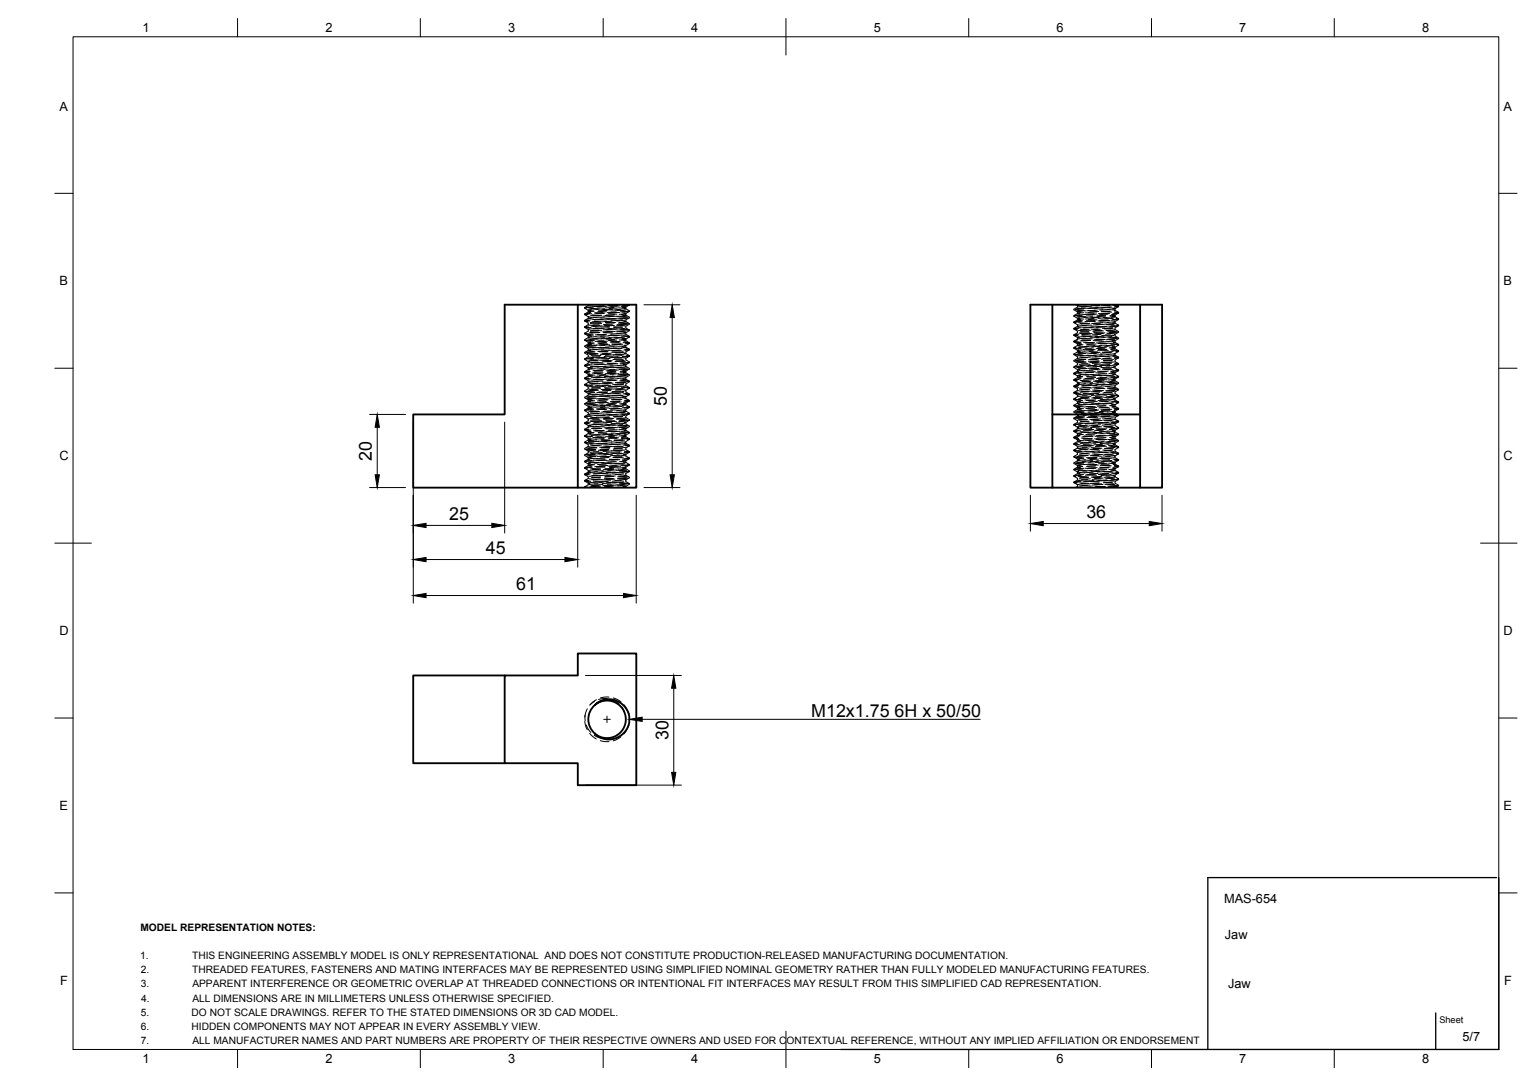
ISO-10303-21;
HEADER;
/* Generated by software containing ST-Developer
 * from STEP Tools, Inc. (www.steptools.com) 
 */

FILE_DESCRIPTION(
/* description */ ('Independent four-jaw lathe chuck,200mm body,40mm bore,36\X2\2013\X0\7
6mm nominal opposed jaw opening. Four shared machined T-jaws and model
ed partial M12x1.75 feed screws, native independent screw/slider links
, removable bolted bronze-bearing cartridges, fully captured ring/wash
er/head thrust stacks and registered bolted backplate. Custom spindle 
interface; no compatibility, speed, grip force or safety rating assign
ed.'),
/* implementation_level */ '2;1');

FILE_NAME(
/* name */ 'Jaw.step',
/* time_stamp */ '2026-11-09T20:24:54-08:00',
/* author */ (''),
/* organization */ (''),
/* preprocessor_version */ 'ST-DEVELOPER v20.2',
/* originating_system */ 'Autodesk Translation Framework v15.17.0.0',
/* authorisation */ '');

FILE_SCHEMA (('AUTOMOTIVE_DESIGN { 1 0 10303 214 3 1 1 }'));
ENDSEC;

DATA;
#10=MECHANICAL_DESIGN_GEOMETRIC_PRESENTATION_REPRESENTATION('',(#238),#69491);
#216=SHAPE_REPRESENTATION_RELATIONSHIP('SRR','None',#69573,#227);
#227=ADVANCED_BREP_SHAPE_REPRESENTATION('',(#249),#69482);
#238=STYLED_ITEM('',(#69637),#249);
#249=MANIFOLD_SOLID_BREP('Body1',#14733);
#290=B_SPLINE_SURFACE_WITH_KNOTS('',3,3,((#46765,#46766,#46767,#46768,#46769,
#46770,#46771,#46772,#46773,#46774,#46775,#46776,#46777,#46778,#46779,#46780,
#46781,#46782,#46783,#46784,#46785,#46786,#46787,#46788,#46789,#46790,#46791,
#46792,#46793,#46794,#46795,#46796,#46797,#46798,#46799,#46800,#46801,#46802,
#46803,#46804,#46805,#46806,#46807,#46808,#46809,#46810,#46811,#46812,#46813,
#46814,#46815,#46816,#46817,#46818,#46819,#46820,#46821,#46822,#46823,#46824,
#46825,#46826,#46827,#46828,#46829,#46830,#46831,#46832,#46833,#46834,#46835,
#46836,#46837,#46838,#46839,#46840,#46841,#46842,#46843,#46844,#46845,#46846,
#46847,#46848,#46849,#46850,#46851,#46852,#46853,#46854,#46855,#46856,#46857,
#46858,#46859,#46860,#46861,#46862,#46863,#46864,#46865,#46866,#46867,#46868,
#46869,#46870,#46871,#46872,#46873,#46874,#46875,#46876,#46877,#46878,#46879,
#46880,#46881,#46882,#46883,#46884,#46885,#46886,#46887,#46888,#46889,#46890,
#46891,#46892,#46893,#46894,#46895,#46896,#46897,#46898,#46899,#46900,#46901,
#46902,#46903,#46904,#46905,#46906,#46907,#46908,#46909,#46910,#46911,#46912,
#46913,#46914,#46915,#46916,#46917,#46918,#46919,#46920,#46921,#46922,#46923,
#46924,#46925,#46926,#46927,#46928,#46929,#46930,#46931,#46932,#46933,#46934,
#46935,#46936,#46937,#46938,#46939,#46940,#46941,#46942,#46943,#46944,#46945,
#46946,#46947,#46948,#46949,#46950,#46951,#46952,#46953,#46954,#46955,#46956,
#46957,#46958,#46959,#46960,#46961,#46962,#46963,#46964,#46965,#46966,#46967,
#46968,#46969,#46970,#46971,#46972,#46973,#46974,#46975,#46976,#46977,#46978,
#46979,#46980,#46981,#46982,#46983,#46984,#46985,#46986,#46987,#46988,#46989,
#46990,#46991,#46992,#46993,#46994,#46995,#46996,#46997,#46998,#46999,#47000,
#47001,#47002,#47003,#47004,#47005,#47006,#47007,#47008,#47009,#47010,#47011,
#47012,#47013,#47014,#47015,#47016,#47017,#47018,#47019,#47020,#47021,#47022,
#47023,#47024,#47025,#47026,#47027,#47028,#47029,#47030,#47031,#47032,#47033,
#47034,#47035,#47036,#47037,#47038,#47039,#47040,#47041,#47042,#47043,#47044,
#47045,#47046,#47047,#47048,#47049,#47050,#47051,#47052,#47053,#47054,#47055,
#47056,#47057,#47058,#47059,#47060,#47061,#47062,#47063,#47064,#47065,#47066,
#47067,#47068,#47069,#47070,#47071,#47072,#47073,#47074,#47075,#47076,#47077,
#47078,#47079,#47080,#47081,#47082,#47083,#47084,#47085,#47086,#47087,#47088,
#47089,#47090,#47091,#47092,#47093,#47094,#47095,#47096,#47097,#47098,#47099,
#47100,#47101,#47102,#47103,#47104,#47105,#47106,#47107,#47108,#47109,#47110,
#47111,#47112,#47113,#47114,#47115,#47116,#47117,#47118,#47119,#47120,#47121,
#47122,#47123,#47124,#47125,#47126,#47127,#47128,#47129,#47130,#47131),
(#47132,#47133,#47134,#47135,#47136,#47137,#47138,#47139,#47140,#47141,
#47142,#47143,#47144,#47145,#47146,#47147,#47148,#47149,#47150,#47151,#47152,
#47153,#47154,#47155,#47156,#47157,#47158,#47159,#47160,#47161,#47162,#47163,
#47164,#47165,#47166,#47167,#47168,#47169,#47170,#47171,#47172,#47173,#47174,
#47175,#47176,#47177,#47178,#47179,#47180,#47181,#47182,#47183,#47184,#47185,
#47186,#47187,#47188,#47189,#47190,#47191,#47192,#47193,#47194,#47195,#47196,
#47197,#47198,#47199,#47200,#47201,#47202,#47203,#47204,#47205,#47206,#47207,
#47208,#47209,#47210,#47211,#47212,#47213,#47214,#47215,#47216,#47217,#47218,
#47219,#47220,#47221,#47222,#47223,#47224,#47225,#47226,#47227,#47228,#47229,
#47230,#47231,#47232,#47233,#47234,#47235,#47236,#47237,#47238,#47239,#47240,
#47241,#47242,#47243,#47244,#47245,#47246,#47247,#47248,#47249,#47250,#47251,
#47252,#47253,#47254,#47255,#47256,#47257,#47258,#47259,#47260,#47261,#47262,
#47263,#47264,#47265,#47266,#47267,#47268,#47269,#47270,#47271,#47272,#47273,
#47274,#47275,#47276,#47277,#47278,#47279,#47280,#47281,#47282,#47283,#47284,
#47285,#47286,#47287,#47288,#47289,#47290,#47291,#47292,#47293,#47294,#47295,
#47296,#47297,#47298,#47299,#47300,#47301,#47302,#47303,#47304,#47305,#47306,
#47307,#47308,#47309,#47310,#47311,#47312,#47313,#47314,#47315,#47316,#47317,
#47318,#47319,#47320,#47321,#47322,#47323,#47324,#47325,#47326,#47327,#47328,
#47329,#47330,#47331,#47332,#47333,#47334,#47335,#47336,#47337,#47338,#47339,
#47340,#47341,#47342,#47343,#47344,#47345,#47346,#47347,#47348,#47349,#47350,
#47351,#47352,#47353,#47354,#47355,#47356,#47357,#47358,#47359,#47360,#47361,
#47362,#47363,#47364,#47365,#47366,#47367,#47368,#47369,#47370,#47371,#47372,
#47373,#47374,#47375,#47376,#47377,#47378,#47379,#47380,#47381,#47382,#47383,
#47384,#47385,#47386,#47387,#47388,#47389,#47390,#47391,#47392,#47393,#47394,
#47395,#47396,#47397,#47398,#47399,#47400,#47401,#47402,#47403,#47404,#47405,
#47406,#47407,#47408,#47409,#47410,#47411,#47412,#47413,#47414,#47415,#47416,
#47417,#47418,#47419,#47420,#47421,#47422,#47423,#47424,#47425,#47426,#47427,
#47428,#47429,#47430,#47431,#47432,#47433,#47434,#47435,#47436,#47437,#47438,
#47439,#47440,#47441,#47442,#47443,#47444,#47445,#47446,#47447,#47448,#47449,
#47450,#47451,#47452,#47453,#47454,#47455,#47456,#47457,#47458,#47459,#47460,
#47461,#47462,#47463,#47464,#47465,#47466,#47467,#47468,#47469,#47470,#47471,
#47472,#47473,#47474,#47475,#47476,#47477,#47478,#47479,#47480,#47481,#47482,
#47483,#47484,#47485,#47486,#47487,#47488,#47489,#47490,#47491,#47492,#47493,
#47494,#47495,#47496,#47497,#47498),(#47499,#47500,#47501,#47502,#47503,
#47504,#47505,#47506,#47507,#47508,#47509,#47510,#47511,#47512,#47513,#47514,
#47515,#47516,#47517,#47518,#47519,#47520,#47521,#47522,#47523,#47524,#47525,
#47526,#47527,#47528,#47529,#47530,#47531,#47532,#47533,#47534,#47535,#47536,
#47537,#47538,#47539,#47540,#47541,#47542,#47543,#47544,#47545,#47546,#47547,
#47548,#47549,#47550,#47551,#47552,#47553,#47554,#47555,#47556,#47557,#47558,
#47559,#47560,#47561,#47562,#47563,#47564,#47565,#47566,#47567,#47568,#47569,
#47570,#47571,#47572,#47573,#47574,#47575,#47576,#47577,#47578,#47579,#47580,
#47581,#47582,#47583,#47584,#47585,#47586,#47587,#47588,#47589,#47590,#47591,
#47592,#47593,#47594,#47595,#47596,#47597,#47598,#47599,#47600,#47601,#47602,
#47603,#47604,#47605,#47606,#47607,#47608,#47609,#47610,#47611,#47612,#47613,
#47614,#47615,#47616,#47617,#47618,#47619,#47620,#47621,#47622,#47623,#47624,
#47625,#47626,#47627,#47628,#47629,#47630,#47631,#47632,#47633,#47634,#47635,
#47636,#47637,#47638,#47639,#47640,#47641,#47642,#47643,#47644,#47645,#47646,
#47647,#47648,#47649,#47650,#47651,#47652,#47653,#47654,#47655,#47656,#47657,
#47658,#47659,#47660,#47661,#47662,#47663,#47664,#47665,#47666,#47667,#47668,
#47669,#47670,#47671,#47672,#47673,#47674,#47675,#47676,#47677,#47678,#47679,
#47680,#47681,#47682,#47683,#47684,#47685,#47686,#47687,#47688,#47689,#47690,
#47691,#47692,#47693,#47694,#47695,#47696,#47697,#47698,#47699,#47700,#47701,
#47702,#47703,#47704,#47705,#47706,#47707,#47708,#47709,#47710,#47711,#47712,
#47713,#47714,#47715,#47716,#47717,#47718,#47719,#47720,#47721,#47722,#47723,
#47724,#47725,#47726,#47727,#47728,#47729,#47730,#47731,#47732,#47733,#47734,
#47735,#47736,#47737,#47738,#47739,#47740,#47741,#47742,#47743,#47744,#47745,
#47746,#47747,#47748,#47749,#47750,#47751,#47752,#47753,#47754,#47755,#47756,
#47757,#47758,#47759,#47760,#47761,#47762,#47763,#47764,#47765,#47766,#47767,
#47768,#47769,#47770,#47771,#47772,#47773,#47774,#47775,#47776,#47777,#47778,
#47779,#47780,#47781,#47782,#47783,#47784,#47785,#47786,#47787,#47788,#47789,
#47790,#47791,#47792,#47793,#47794,#47795,#47796,#47797,#47798,#47799,#47800,
#47801,#47802,#47803,#47804,#47805,#47806,#47807,#47808,#47809,#47810,#47811,
#47812,#47813,#47814,#47815,#47816,#47817,#47818,#47819,#47820,#47821,#47822,
#47823,#47824,#47825,#47826,#47827,#47828,#47829,#47830,#47831,#47832,#47833,
#47834,#47835,#47836,#47837,#47838,#47839,#47840,#47841,#47842,#47843,#47844,
#47845,#47846,#47847,#47848,#47849,#47850,#47851,#47852,#47853,#47854,#47855,
#47856,#47857,#47858,#47859,#47860,#47861,#47862,#47863,#47864,#47865),
(#47866,#47867,#47868,#47869,#47870,#47871,#47872,#47873,#47874,#47875,
#47876,#47877,#47878,#47879,#47880,#47881,#47882,#47883,#47884,#47885,#47886,
#47887,#47888,#47889,#47890,#47891,#47892,#47893,#47894,#47895,#47896,#47897,
#47898,#47899,#47900,#47901,#47902,#47903,#47904,#47905,#47906,#47907,#47908,
#47909,#47910,#47911,#47912,#47913,#47914,#47915,#47916,#47917,#47918,#47919,
#47920,#47921,#47922,#47923,#47924,#47925,#47926,#47927,#47928,#47929,#47930,
#47931,#47932,#47933,#47934,#47935,#47936,#47937,#47938,#47939,#47940,#47941,
#47942,#47943,#47944,#47945,#47946,#47947,#47948,#47949,#47950,#47951,#47952,
#47953,#47954,#47955,#47956,#47957,#47958,#47959,#47960,#47961,#47962,#47963,
#47964,#47965,#47966,#47967,#47968,#47969,#47970,#47971,#47972,#47973,#47974,
#47975,#47976,#47977,#47978,#47979,#47980,#47981,#47982,#47983,#47984,#47985,
#47986,#47987,#47988,#47989,#47990,#47991,#47992,#47993,#47994,#47995,#47996,
#47997,#47998,#47999,#48000,#48001,#48002,#48003,#48004,#48005,#48006,#48007,
#48008,#48009,#48010,#48011,#48012,#48013,#48014,#48015,#48016,#48017,#48018,
#48019,#48020,#48021,#48022,#48023,#48024,#48025,#48026,#48027,#48028,#48029,
#48030,#48031,#48032,#48033,#48034,#48035,#48036,#48037,#48038,#48039,#48040,
#48041,#48042,#48043,#48044,#48045,#48046,#48047,#48048,#48049,#48050,#48051,
#48052,#48053,#48054,#48055,#48056,#48057,#48058,#48059,#48060,#48061,#48062,
#48063,#48064,#48065,#48066,#48067,#48068,#48069,#48070,#48071,#48072,#48073,
#48074,#48075,#48076,#48077,#48078,#48079,#48080,#48081,#48082,#48083,#48084,
#48085,#48086,#48087,#48088,#48089,#48090,#48091,#48092,#48093,#48094,#48095,
#48096,#48097,#48098,#48099,#48100,#48101,#48102,#48103,#48104,#48105,#48106,
#48107,#48108,#48109,#48110,#48111,#48112,#48113,#48114,#48115,#48116,#48117,
#48118,#48119,#48120,#48121,#48122,#48123,#48124,#48125,#48126,#48127,#48128,
#48129,#48130,#48131,#48132,#48133,#48134,#48135,#48136,#48137,#48138,#48139,
#48140,#48141,#48142,#48143,#48144,#48145,#48146,#48147,#48148,#48149,#48150,
#48151,#48152,#48153,#48154,#48155,#48156,#48157,#48158,#48159,#48160,#48161,
#48162,#48163,#48164,#48165,#48166,#48167,#48168,#48169,#48170,#48171,#48172,
#48173,#48174,#48175,#48176,#48177,#48178,#48179,#48180,#48181,#48182,#48183,
#48184,#48185,#48186,#48187,#48188,#48189,#48190,#48191,#48192,#48193,#48194,
#48195,#48196,#48197,#48198,#48199,#48200,#48201,#48202,#48203,#48204,#48205,
#48206,#48207,#48208,#48209,#48210,#48211,#48212,#48213,#48214,#48215,#48216,
#48217,#48218,#48219,#48220,#48221,#48222,#48223,#48224,#48225,#48226,#48227,
#48228,#48229,#48230,#48231,#48232)),.UNSPECIFIED.,.F.,.F.,.F.,(4,4),(4,
1,1,1,1,1,1,1,1,1,1,1,1,1,1,1,1,1,1,1,1,1,1,1,1,1,1,1,1,1,1,1,1,1,1,1,1,
1,1,1,1,1,1,1,1,1,1,1,1,1,1,1,1,1,1,1,1,1,1,1,1,1,1,1,1,1,1,1,1,1,1,1,1,
1,1,1,1,1,1,1,1,1,1,1,1,1,1,1,1,1,1,1,1,1,1,1,1,1,1,1,1,1,1,1,1,1,1,1,1,
1,1,1,1,1,1,1,1,1,1,1,1,1,1,1,1,1,1,1,1,1,1,1,1,1,1,1,1,1,1,1,1,1,1,1,1,
1,1,1,1,1,1,1,1,1,1,1,1,1,1,1,1,1,1,1,1,1,1,1,1,1,1,1,1,1,1,1,1,1,1,1,1,
1,1,1,1,1,1,1,1,1,1,1,1,1,1,1,1,1,1,1,1,1,1,1,1,1,1,1,1,1,1,1,1,1,1,1,1,
1,1,1,1,1,1,1,1,1,1,1,1,1,1,1,1,1,1,1,1,1,1,1,1,1,1,1,1,1,1,1,1,1,1,1,1,
1,1,1,1,1,1,1,1,1,1,1,1,1,1,1,1,1,1,1,1,1,1,1,1,1,1,1,1,1,1,1,1,1,1,1,1,
1,1,1,1,1,1,1,1,1,1,1,1,1,1,1,1,1,1,1,1,1,1,1,1,1,1,1,1,1,1,1,1,1,1,1,1,
1,1,1,1,1,1,1,1,1,1,1,1,1,1,1,1,1,1,1,1,1,1,1,1,1,1,1,1,1,1,1,1,1,1,1,1,
1,1,1,4),(0.,0.112756507572734),(11.8517336648509,12.3504803140147,12.8492269631785,
13.3479736123423,13.8467202615061,14.3454669106698,14.8442135598336,15.3429602089974,
15.8417068581612,16.340453507325,16.8392001564888,17.3379468056525,17.8366934548163,
18.3354401039801,18.8341867531439,19.3329334023077,19.8316800514714,20.3304267006352,
20.829173349799,21.3279199989628,21.8266666481266,22.3254132972903,22.8241599464541,
23.3229065956179,23.8216532447817,24.3203998939455,24.8191465431093,25.317893192273,
25.8166398414368,26.3153864906006,26.8141331397644,27.3128797889282,27.8116264380919,
28.3103730872557,28.8091197364195,29.3078663855833,29.8066130347471,30.3053596839108,
30.8041063330746,31.3028529822384,31.8015996314022,32.300346280566,32.7990929297298,
33.2978395788935,33.7965862280573,34.2953328772211,34.7940795263849,35.2928261755487,
35.7915728247124,36.2903194738762,36.78906612304,37.2878127722038,37.7865594213676,
38.2853060705313,38.7840527196951,39.2827993688589,39.7815460180227,40.2802926671865,
40.7790393163503,41.277785965514,41.7765326146778,42.2752792638416,42.7740259130054,
43.2727725621692,43.7715192113329,44.2702658604967,44.7690125096605,45.2677591588243,
45.7665058079881,46.2652524571519,46.7639991063156,47.2627457554794,47.7614924046432,
48.260239053807,48.7589857029708,49.2577323521345,49.7564790012983,50.2552256504621,
50.7539722996259,51.2527189487897,51.7514655979534,52.2502122471172,52.748958896281,
53.2477055454448,53.7464521946086,54.2451988437724,54.7439454929361,55.2426921420999,
55.7414387912637,56.2401854404275,56.7389320895913,57.237678738755,57.7364253879188,
58.2351720370826,58.7339186862464,59.2326653354102,59.731411984574,60.2301586337377,
60.7289052829015,61.2276519320653,61.7263985812291,62.2251452303929,62.7238918795566,
63.2226385287204,63.7213851778842,64.220131827048,64.7188784762118,65.2176251253755,
65.7163717745393,66.2151184237031,66.7138650728669,67.2126117220307,67.7113583711945,
68.2101050203582,68.708851669522,69.2075983186858,69.7063449678496,70.2050916170134,
70.7038382661771,71.2025849153409,71.7013315645047,72.2000782136685,72.6988248628323,
73.197571511996,73.6963181611598,74.1950648103236,74.6938114594874,75.1925581086512,
75.6913047578149,76.1900514069787,76.6887980561425,77.1875447053063,77.6862913544701,
78.1850380036339,78.6837846527976,79.1825313019614,79.6812779511252,80.180024600289,
80.6787712494528,81.1775178986165,81.6762645477803,82.1750111969441,82.6737578461079,
83.1725044952717,83.6712511444355,84.1699977935992,84.668744442763,85.1674910919268,
85.6662377410906,86.1649843902544,86.6637310394181,87.1624776885819,87.6612243377457,
88.1599709869095,88.6587176360733,89.1574642852371,89.6562109344008,90.1549575835646,
90.6537042327284,91.1524508818922,91.651197531056,92.1499441802197,92.6486908293835,
93.1474374785473,93.6461841277111,94.1449307768749,94.6436774260386,95.1424240752024,
95.6411707243662,96.13991737353,96.6386640226938,97.1374106718576,97.6361573210213,
98.1349039701851,98.6336506193489,99.1323972685127,99.6311439176765,100.12989056684,
100.628637216004,101.127383865168,101.626130514332,102.124877163495,102.623623812659,
103.122370461823,103.621117110987,104.11986376015,104.618610409314,105.117357058478,
105.616103707642,106.114850356806,106.613597005969,107.112343655133,107.611090304297,
108.109836953461,108.608583602625,109.107330251788,109.606076900952,110.104823550116,
110.60357019928,111.102316848443,111.601063497607,112.099810146771,112.598556795935,
113.097303445099,113.596050094262,114.094796743426,114.59354339259,115.092290041754,
115.591036690917,116.089783340081,116.588529989245,117.087276638409,117.586023287573,
118.084769936736,118.5835165859,119.082263235064,119.581009884228,120.079756533392,
120.578503182555,121.077249831719,121.575996480883,122.074743130047,122.57348977921,
123.072236428374,123.570983077538,124.069729726702,124.568476375866,125.067223025029,
125.565969674193,126.064716323357,126.563462972521,127.062209621684,127.560956270848,
128.059702920012,128.558449569176,129.05719621834,129.555942867503,130.054689516667,
130.553436165831,131.052182814995,131.550929464158,132.049676113322,132.548422762486,
133.04716941165,133.545916060814,134.044662709977,134.543409359141,135.042156008305,
135.540902657469,136.039649306632,136.538395955796,137.03714260496,137.535889254124,
138.034635903288,138.533382552451,139.032129201615,139.530875850779,140.029622499943,
140.528369149107,141.02711579827,141.525862447434,142.024609096598,142.523355745762,
143.022102394925,143.520849044089,144.019595693253,144.518342342417,145.017088991581,
145.515835640744,146.014582289908,146.513328939072,147.012075588236,147.510822237399,
148.009568886563,148.508315535727,149.007062184891,149.505808834055,150.004555483218,
150.503302132382,151.002048781546,151.50079543071,151.999542079873,152.498288729037,
152.997035378201,153.495782027365,153.994528676529,154.493275325692,154.992021974856,
155.49076862402,155.989515273184,156.488261922348,156.987008571511,157.485755220675,
157.984501869839,158.483248519003,158.981995168166,159.48074181733,159.979488466494,
160.478235115658,160.976981764822,161.475728413985,161.974475063149,162.473221712313,
162.971968361477,163.47071501064,163.969461659804,164.468208308968,164.966954958132,
165.465701607296,165.964448256459,166.463194905623,166.961941554787,167.460688203951,
167.959434853114,168.458181502278,168.956928151442,169.455674800606,169.95442144977,
170.453168098933,170.951914748097,171.450661397261,171.949408046425,172.448154695589,
172.946901344752,173.445647993916,173.94439464308,174.443141292244,174.941887941407,
175.440634590571,175.939381239735,176.438127888899,176.936874538063,177.435621187226,
177.93436783639,178.433114485554,178.931861134718,179.430607783881,179.929354433045,
180.428101082209,180.926847731373,181.425594380537,181.9243410297,182.423087678864,
182.921834328028,183.420580977192,183.919327626356,184.418074275519,184.916820924683,
185.415567573847,185.914314223011,186.413060872174,186.911807521338,187.410554170502,
187.909300819666,188.40804746883,188.906794117993,189.405540767157,189.904287416321,
190.403034065485,190.901780714648,191.400527363812,191.899274012976,192.39802066214,
192.896767311304,193.395513960467),.UNSPECIFIED.);
#291=B_SPLINE_SURFACE_WITH_KNOTS('',3,3,((#48500,#48501,#48502,#48503,#48504,
#48505,#48506,#48507,#48508,#48509,#48510,#48511,#48512,#48513,#48514,#48515,
#48516,#48517,#48518,#48519,#48520,#48521,#48522,#48523,#48524,#48525,#48526,
#48527,#48528,#48529,#48530,#48531,#48532,#48533,#48534,#48535,#48536,#48537,
#48538,#48539,#48540,#48541,#48542,#48543,#48544,#48545,#48546,#48547,#48548,
#48549,#48550,#48551,#48552,#48553,#48554,#48555,#48556,#48557,#48558,#48559,
#48560,#48561,#48562,#48563,#48564,#48565,#48566,#48567,#48568,#48569,#48570,
#48571,#48572,#48573,#48574,#48575,#48576,#48577,#48578,#48579,#48580,#48581,
#48582,#48583,#48584,#48585,#48586,#48587,#48588,#48589,#48590,#48591,#48592,
#48593,#48594,#48595,#48596,#48597,#48598,#48599,#48600,#48601,#48602,#48603,
#48604,#48605,#48606,#48607,#48608,#48609,#48610,#48611,#48612,#48613,#48614,
#48615,#48616,#48617,#48618,#48619,#48620,#48621,#48622,#48623,#48624,#48625,
#48626,#48627,#48628,#48629,#48630,#48631,#48632,#48633,#48634,#48635,#48636,
#48637,#48638,#48639,#48640,#48641,#48642,#48643,#48644,#48645,#48646,#48647,
#48648,#48649,#48650,#48651,#48652,#48653,#48654,#48655,#48656,#48657,#48658,
#48659,#48660,#48661,#48662,#48663,#48664,#48665,#48666,#48667,#48668,#48669,
#48670,#48671,#48672,#48673,#48674,#48675,#48676,#48677,#48678,#48679,#48680,
#48681,#48682,#48683,#48684,#48685,#48686,#48687,#48688,#48689,#48690,#48691,
#48692,#48693,#48694,#48695,#48696,#48697,#48698,#48699,#48700,#48701,#48702,
#48703,#48704,#48705,#48706,#48707,#48708,#48709,#48710,#48711,#48712,#48713,
#48714,#48715,#48716,#48717,#48718,#48719,#48720,#48721,#48722,#48723,#48724,
#48725,#48726,#48727,#48728,#48729,#48730,#48731,#48732,#48733,#48734,#48735,
#48736,#48737,#48738,#48739,#48740,#48741,#48742,#48743,#48744,#48745,#48746,
#48747,#48748,#48749,#48750,#48751,#48752,#48753,#48754,#48755,#48756,#48757,
#48758,#48759,#48760,#48761,#48762,#48763,#48764,#48765,#48766,#48767,#48768,
#48769,#48770,#48771,#48772,#48773,#48774,#48775,#48776,#48777,#48778,#48779,
#48780,#48781,#48782,#48783,#48784,#48785,#48786,#48787,#48788,#48789,#48790,
#48791,#48792,#48793,#48794,#48795,#48796,#48797,#48798,#48799,#48800,#48801,
#48802,#48803,#48804,#48805,#48806,#48807,#48808,#48809,#48810,#48811,#48812,
#48813,#48814,#48815,#48816,#48817,#48818,#48819,#48820,#48821,#48822,#48823,
#48824,#48825,#48826,#48827,#48828,#48829,#48830,#48831,#48832,#48833,#48834,
#48835,#48836,#48837,#48838,#48839,#48840,#48841,#48842,#48843,#48844,#48845,
#48846,#48847,#48848,#48849,#48850,#48851,#48852,#48853,#48854,#48855,#48856,
#48857,#48858,#48859,#48860,#48861,#48862,#48863,#48864,#48865,#48866),
(#48867,#48868,#48869,#48870,#48871,#48872,#48873,#48874,#48875,#48876,
#48877,#48878,#48879,#48880,#48881,#48882,#48883,#48884,#48885,#48886,#48887,
#48888,#48889,#48890,#48891,#48892,#48893,#48894,#48895,#48896,#48897,#48898,
#48899,#48900,#48901,#48902,#48903,#48904,#48905,#48906,#48907,#48908,#48909,
#48910,#48911,#48912,#48913,#48914,#48915,#48916,#48917,#48918,#48919,#48920,
#48921,#48922,#48923,#48924,#48925,#48926,#48927,#48928,#48929,#48930,#48931,
#48932,#48933,#48934,#48935,#48936,#48937,#48938,#48939,#48940,#48941,#48942,
#48943,#48944,#48945,#48946,#48947,#48948,#48949,#48950,#48951,#48952,#48953,
#48954,#48955,#48956,#48957,#48958,#48959,#48960,#48961,#48962,#48963,#48964,
#48965,#48966,#48967,#48968,#48969,#48970,#48971,#48972,#48973,#48974,#48975,
#48976,#48977,#48978,#48979,#48980,#48981,#48982,#48983,#48984,#48985,#48986,
#48987,#48988,#48989,#48990,#48991,#48992,#48993,#48994,#48995,#48996,#48997,
#48998,#48999,#49000,#49001,#49002,#49003,#49004,#49005,#49006,#49007,#49008,
#49009,#49010,#49011,#49012,#49013,#49014,#49015,#49016,#49017,#49018,#49019,
#49020,#49021,#49022,#49023,#49024,#49025,#49026,#49027,#49028,#49029,#49030,
#49031,#49032,#49033,#49034,#49035,#49036,#49037,#49038,#49039,#49040,#49041,
#49042,#49043,#49044,#49045,#49046,#49047,#49048,#49049,#49050,#49051,#49052,
#49053,#49054,#49055,#49056,#49057,#49058,#49059,#49060,#49061,#49062,#49063,
#49064,#49065,#49066,#49067,#49068,#49069,#49070,#49071,#49072,#49073,#49074,
#49075,#49076,#49077,#49078,#49079,#49080,#49081,#49082,#49083,#49084,#49085,
#49086,#49087,#49088,#49089,#49090,#49091,#49092,#49093,#49094,#49095,#49096,
#49097,#49098,#49099,#49100,#49101,#49102,#49103,#49104,#49105,#49106,#49107,
#49108,#49109,#49110,#49111,#49112,#49113,#49114,#49115,#49116,#49117,#49118,
#49119,#49120,#49121,#49122,#49123,#49124,#49125,#49126,#49127,#49128,#49129,
#49130,#49131,#49132,#49133,#49134,#49135,#49136,#49137,#49138,#49139,#49140,
#49141,#49142,#49143,#49144,#49145,#49146,#49147,#49148,#49149,#49150,#49151,
#49152,#49153,#49154,#49155,#49156,#49157,#49158,#49159,#49160,#49161,#49162,
#49163,#49164,#49165,#49166,#49167,#49168,#49169,#49170,#49171,#49172,#49173,
#49174,#49175,#49176,#49177,#49178,#49179,#49180,#49181,#49182,#49183,#49184,
#49185,#49186,#49187,#49188,#49189,#49190,#49191,#49192,#49193,#49194,#49195,
#49196,#49197,#49198,#49199,#49200,#49201,#49202,#49203,#49204,#49205,#49206,
#49207,#49208,#49209,#49210,#49211,#49212,#49213,#49214,#49215,#49216,#49217,
#49218,#49219,#49220,#49221,#49222,#49223,#49224,#49225,#49226,#49227,#49228,
#49229,#49230,#49231,#49232,#49233),(#49234,#49235,#49236,#49237,#49238,
#49239,#49240,#49241,#49242,#49243,#49244,#49245,#49246,#49247,#49248,#49249,
#49250,#49251,#49252,#49253,#49254,#49255,#49256,#49257,#49258,#49259,#49260,
#49261,#49262,#49263,#49264,#49265,#49266,#49267,#49268,#49269,#49270,#49271,
#49272,#49273,#49274,#49275,#49276,#49277,#49278,#49279,#49280,#49281,#49282,
#49283,#49284,#49285,#49286,#49287,#49288,#49289,#49290,#49291,#49292,#49293,
#49294,#49295,#49296,#49297,#49298,#49299,#49300,#49301,#49302,#49303,#49304,
#49305,#49306,#49307,#49308,#49309,#49310,#49311,#49312,#49313,#49314,#49315,
#49316,#49317,#49318,#49319,#49320,#49321,#49322,#49323,#49324,#49325,#49326,
#49327,#49328,#49329,#49330,#49331,#49332,#49333,#49334,#49335,#49336,#49337,
#49338,#49339,#49340,#49341,#49342,#49343,#49344,#49345,#49346,#49347,#49348,
#49349,#49350,#49351,#49352,#49353,#49354,#49355,#49356,#49357,#49358,#49359,
#49360,#49361,#49362,#49363,#49364,#49365,#49366,#49367,#49368,#49369,#49370,
#49371,#49372,#49373,#49374,#49375,#49376,#49377,#49378,#49379,#49380,#49381,
#49382,#49383,#49384,#49385,#49386,#49387,#49388,#49389,#49390,#49391,#49392,
#49393,#49394,#49395,#49396,#49397,#49398,#49399,#49400,#49401,#49402,#49403,
#49404,#49405,#49406,#49407,#49408,#49409,#49410,#49411,#49412,#49413,#49414,
#49415,#49416,#49417,#49418,#49419,#49420,#49421,#49422,#49423,#49424,#49425,
#49426,#49427,#49428,#49429,#49430,#49431,#49432,#49433,#49434,#49435,#49436,
#49437,#49438,#49439,#49440,#49441,#49442,#49443,#49444,#49445,#49446,#49447,
#49448,#49449,#49450,#49451,#49452,#49453,#49454,#49455,#49456,#49457,#49458,
#49459,#49460,#49461,#49462,#49463,#49464,#49465,#49466,#49467,#49468,#49469,
#49470,#49471,#49472,#49473,#49474,#49475,#49476,#49477,#49478,#49479,#49480,
#49481,#49482,#49483,#49484,#49485,#49486,#49487,#49488,#49489,#49490,#49491,
#49492,#49493,#49494,#49495,#49496,#49497,#49498,#49499,#49500,#49501,#49502,
#49503,#49504,#49505,#49506,#49507,#49508,#49509,#49510,#49511,#49512,#49513,
#49514,#49515,#49516,#49517,#49518,#49519,#49520,#49521,#49522,#49523,#49524,
#49525,#49526,#49527,#49528,#49529,#49530,#49531,#49532,#49533,#49534,#49535,
#49536,#49537,#49538,#49539,#49540,#49541,#49542,#49543,#49544,#49545,#49546,
#49547,#49548,#49549,#49550,#49551,#49552,#49553,#49554,#49555,#49556,#49557,
#49558,#49559,#49560,#49561,#49562,#49563,#49564,#49565,#49566,#49567,#49568,
#49569,#49570,#49571,#49572,#49573,#49574,#49575,#49576,#49577,#49578,#49579,
#49580,#49581,#49582,#49583,#49584,#49585,#49586,#49587,#49588,#49589,#49590,
#49591,#49592,#49593,#49594,#49595,#49596,#49597,#49598,#49599,#49600),
(#49601,#49602,#49603,#49604,#49605,#49606,#49607,#49608,#49609,#49610,
#49611,#49612,#49613,#49614,#49615,#49616,#49617,#49618,#49619,#49620,#49621,
#49622,#49623,#49624,#49625,#49626,#49627,#49628,#49629,#49630,#49631,#49632,
#49633,#49634,#49635,#49636,#49637,#49638,#49639,#49640,#49641,#49642,#49643,
#49644,#49645,#49646,#49647,#49648,#49649,#49650,#49651,#49652,#49653,#49654,
#49655,#49656,#49657,#49658,#49659,#49660,#49661,#49662,#49663,#49664,#49665,
#49666,#49667,#49668,#49669,#49670,#49671,#49672,#49673,#49674,#49675,#49676,
#49677,#49678,#49679,#49680,#49681,#49682,#49683,#49684,#49685,#49686,#49687,
#49688,#49689,#49690,#49691,#49692,#49693,#49694,#49695,#49696,#49697,#49698,
#49699,#49700,#49701,#49702,#49703,#49704,#49705,#49706,#49707,#49708,#49709,
#49710,#49711,#49712,#49713,#49714,#49715,#49716,#49717,#49718,#49719,#49720,
#49721,#49722,#49723,#49724,#49725,#49726,#49727,#49728,#49729,#49730,#49731,
#49732,#49733,#49734,#49735,#49736,#49737,#49738,#49739,#49740,#49741,#49742,
#49743,#49744,#49745,#49746,#49747,#49748,#49749,#49750,#49751,#49752,#49753,
#49754,#49755,#49756,#49757,#49758,#49759,#49760,#49761,#49762,#49763,#49764,
#49765,#49766,#49767,#49768,#49769,#49770,#49771,#49772,#49773,#49774,#49775,
#49776,#49777,#49778,#49779,#49780,#49781,#49782,#49783,#49784,#49785,#49786,
#49787,#49788,#49789,#49790,#49791,#49792,#49793,#49794,#49795,#49796,#49797,
#49798,#49799,#49800,#49801,#49802,#49803,#49804,#49805,#49806,#49807,#49808,
#49809,#49810,#49811,#49812,#49813,#49814,#49815,#49816,#49817,#49818,#49819,
#49820,#49821,#49822,#49823,#49824,#49825,#49826,#49827,#49828,#49829,#49830,
#49831,#49832,#49833,#49834,#49835,#49836,#49837,#49838,#49839,#49840,#49841,
#49842,#49843,#49844,#49845,#49846,#49847,#49848,#49849,#49850,#49851,#49852,
#49853,#49854,#49855,#49856,#49857,#49858,#49859,#49860,#49861,#49862,#49863,
#49864,#49865,#49866,#49867,#49868,#49869,#49870,#49871,#49872,#49873,#49874,
#49875,#49876,#49877,#49878,#49879,#49880,#49881,#49882,#49883,#49884,#49885,
#49886,#49887,#49888,#49889,#49890,#49891,#49892,#49893,#49894,#49895,#49896,
#49897,#49898,#49899,#49900,#49901,#49902,#49903,#49904,#49905,#49906,#49907,
#49908,#49909,#49910,#49911,#49912,#49913,#49914,#49915,#49916,#49917,#49918,
#49919,#49920,#49921,#49922,#49923,#49924,#49925,#49926,#49927,#49928,#49929,
#49930,#49931,#49932,#49933,#49934,#49935,#49936,#49937,#49938,#49939,#49940,
#49941,#49942,#49943,#49944,#49945,#49946,#49947,#49948,#49949,#49950,#49951,
#49952,#49953,#49954,#49955,#49956,#49957,#49958,#49959,#49960,#49961,#49962,
#49963,#49964,#49965,#49966,#49967)),.UNSPECIFIED.,.F.,.F.,.F.,(4,4),(4,
1,1,1,1,1,1,1,1,1,1,1,1,1,1,1,1,1,1,1,1,1,1,1,1,1,1,1,1,1,1,1,1,1,1,1,1,
1,1,1,1,1,1,1,1,1,1,1,1,1,1,1,1,1,1,1,1,1,1,1,1,1,1,1,1,1,1,1,1,1,1,1,1,
1,1,1,1,1,1,1,1,1,1,1,1,1,1,1,1,1,1,1,1,1,1,1,1,1,1,1,1,1,1,1,1,1,1,1,1,
1,1,1,1,1,1,1,1,1,1,1,1,1,1,1,1,1,1,1,1,1,1,1,1,1,1,1,1,1,1,1,1,1,1,1,1,
1,1,1,1,1,1,1,1,1,1,1,1,1,1,1,1,1,1,1,1,1,1,1,1,1,1,1,1,1,1,1,1,1,1,1,1,
1,1,1,1,1,1,1,1,1,1,1,1,1,1,1,1,1,1,1,1,1,1,1,1,1,1,1,1,1,1,1,1,1,1,1,1,
1,1,1,1,1,1,1,1,1,1,1,1,1,1,1,1,1,1,1,1,1,1,1,1,1,1,1,1,1,1,1,1,1,1,1,1,
1,1,1,1,1,1,1,1,1,1,1,1,1,1,1,1,1,1,1,1,1,1,1,1,1,1,1,1,1,1,1,1,1,1,1,1,
1,1,1,1,1,1,1,1,1,1,1,1,1,1,1,1,1,1,1,1,1,1,1,1,1,1,1,1,1,1,1,1,1,1,1,1,
1,1,1,1,1,1,1,1,1,1,1,1,1,1,1,1,1,1,1,1,1,1,1,1,1,1,1,1,1,1,1,1,1,1,1,1,
1,1,1,4),(0.,0.112756507572734),(14.3984001269719,14.8971467761357,15.3958934252995,
15.8946400744633,16.393386723627,16.8921333727908,17.3908800219546,17.8896266711184,
18.3883733202822,18.887119969446,19.3858666186097,19.8846132677735,20.3833599169373,
20.8821065661011,21.3808532152649,21.8795998644286,22.3783465135924,22.8770931627562,
23.37583981192,23.8745864610838,24.3733331102476,24.8720797594113,25.3708264085751,
25.8695730577389,26.3683197069027,26.8670663560665,27.3658130052302,27.864559654394,
28.3633063035578,28.8620529527216,29.3607996018854,29.8595462510491,30.3582929002129,
30.8570395493767,31.3557861985405,31.8545328477043,32.353279496868,32.8520261460318,
33.3507727951956,33.8495194443594,34.3482660935232,34.847012742687,35.3457593918507,
35.8445060410145,36.3432526901783,36.8419993393421,37.3407459885059,37.8394926376697,
38.3382392868334,38.8369859359972,39.335732585161,39.8344792343248,40.3332258834886,
40.8319725326523,41.3307191818161,41.8294658309799,42.3282124801437,42.8269591293075,
43.3257057784712,43.824452427635,44.3231990767988,44.8219457259626,45.3206923751264,
45.8194390242901,46.3181856734539,46.8169323226177,47.3156789717815,47.8144256209453,
48.313172270109,48.8119189192728,49.3106655684366,49.8094122176004,50.3081588667642,
50.806905515928,51.3056521650917,51.8043988142555,52.3031454634193,52.8018921125831,
53.3006387617469,53.7993854109106,54.2981320600744,54.7968787092382,55.295625358402,
55.7943720075658,56.2931186567296,56.7918653058933,57.2906119550571,57.7893586042209,
58.2881052533847,58.7868519025485,59.2855985517122,59.784345200876,60.2830918500398,
60.7818384992036,61.2805851483674,61.7793317975311,62.2780784466949,62.7768250958587,
63.2755717450225,63.7743183941863,64.2730650433501,64.7718116925138,65.2705583416776,
65.7693049908414,66.2680516400052,66.766798289169,67.2655449383327,67.7642915874965,
68.2630382366603,68.7617848858241,69.2605315349879,69.7592781841516,70.2580248333154,
70.7567714824792,71.255518131643,71.7542647808068,72.2530114299706,72.7517580791343,
73.2505047282981,73.7492513774619,74.2479980266257,74.7467446757895,75.2454913249532,
75.744237974117,76.2429846232808,76.7417312724446,77.2404779216084,77.7392245707722,
78.2379712199359,78.7367178690997,79.2354645182635,79.7342111674273,80.2329578165911,
80.7317044657548,81.2304511149186,81.7291977640824,82.2279444132462,82.72669106241,
83.2254377115737,83.7241843607375,84.2229310099013,84.7216776590651,85.2204243082289,
85.7191709573926,86.2179176065564,86.7166642557202,87.215410904884,87.7141575540478,
88.2129042032116,88.7116508523753,89.2103975015391,89.7091441507029,90.2078907998667,
90.7066374490305,91.2053840981942,91.704130747358,92.2028773965218,92.7016240456856,
93.2003706948494,93.6991173440131,94.1978639931769,94.6966106423407,95.1953572915045,
95.6941039406683,96.1928505898321,96.6915972389958,97.1903438881596,97.6890905373234,
98.1878371864872,98.686583835651,99.1853304848147,99.6840771339785,100.182823783142,
100.681570432306,101.18031708147,101.679063730634,102.177810379797,102.676557028961,
103.175303678125,103.674050327289,104.172796976453,104.671543625616,105.17029027478,
105.669036923944,106.167783573108,106.666530222271,107.165276871435,107.664023520599,
108.162770169763,108.661516818927,109.16026346809,109.659010117254,110.157756766418,
110.656503415582,111.155250064746,111.653996713909,112.152743363073,112.651490012237,
113.150236661401,113.648983310564,114.147729959728,114.646476608892,115.145223258056,
115.64396990722,116.142716556383,116.641463205547,117.140209854711,117.638956503875,
118.137703153038,118.636449802202,119.135196451366,119.63394310053,120.132689749694,
120.631436398857,121.130183048021,121.628929697185,122.127676346349,122.626422995512,
123.125169644676,123.62391629384,124.122662943004,124.621409592168,125.120156241331,
125.618902890495,126.117649539659,126.616396188823,127.115142837986,127.61388948715,
128.112636136314,128.611382785478,129.110129434642,129.608876083805,130.107622732969,
130.606369382133,131.105116031297,131.603862680461,132.102609329624,132.601355978788,
133.100102627952,133.598849277116,134.097595926279,134.596342575443,135.095089224607,
135.593835873771,136.092582522935,136.591329172098,137.090075821262,137.588822470426,
138.08756911959,138.586315768753,139.085062417917,139.583809067081,140.082555716245,
140.581302365409,141.080049014572,141.578795663736,142.0775423129,142.576288962064,
143.075035611227,143.573782260391,144.072528909555,144.571275558719,145.070022207883,
145.568768857046,146.06751550621,146.566262155374,147.065008804538,147.563755453702,
148.062502102865,148.561248752029,149.059995401193,149.558742050357,150.05748869952,
150.556235348684,151.054981997848,151.553728647012,152.052475296176,152.551221945339,
153.049968594503,153.548715243667,154.047461892831,154.546208541994,155.044955191158,
155.543701840322,156.042448489486,156.54119513865,157.039941787813,157.538688436977,
158.037435086141,158.536181735305,159.034928384469,159.533675033632,160.032421682796,
160.53116833196,161.029914981124,161.528661630287,162.027408279451,162.526154928615,
163.024901577779,163.523648226943,164.022394876106,164.52114152527,165.019888174434,
165.518634823598,166.017381472761,166.516128121925,167.014874771089,167.513621420253,
168.012368069417,168.51111471858,169.009861367744,169.508608016908,170.007354666072,
170.506101315235,171.004847964399,171.503594613563,172.002341262727,172.501087911891,
172.999834561054,173.498581210218,173.997327859382,174.496074508546,174.99482115771,
175.493567806873,175.992314456037,176.491061105201,176.989807754365,177.488554403528,
177.987301052692,178.486047701856,178.98479435102,179.483541000184,179.982287649347,
180.481034298511,180.979780947675,181.478527596839,181.977274246002,182.476020895166,
182.97476754433,183.473514193494,183.972260842658,184.471007491821,184.969754140985,
185.468500790149,185.967247439313,186.465994088476,186.96474073764,187.463487386804,
187.962234035968,188.460980685132,188.959727334295,189.458473983459,189.957220632623,
190.455967281787,190.954713930951,191.453460580114,191.952207229278,192.450953878442,
192.949700527606,193.448447176769,193.947193825933,194.445940475097,194.944687124261,
195.443433773425,195.942180422588),.UNSPECIFIED.);
#343=FACE_BOUND('',#1808,.T.);
#344=FACE_BOUND('',#1820,.T.);
#450=PLANE('',#15433);
#451=PLANE('',#15435);
#452=PLANE('',#15436);
#453=PLANE('',#15437);
#454=PLANE('',#15438);
#455=PLANE('',#15439);
#456=PLANE('',#15440);
#457=PLANE('',#15441);
#458=PLANE('',#15442);
#459=PLANE('',#15443);
#460=PLANE('',#15444);
#461=PLANE('',#15445);
#921=FACE_OUTER_BOUND('',#1747,.T.);
#922=FACE_OUTER_BOUND('',#1748,.T.);
#923=FACE_OUTER_BOUND('',#1749,.T.);
#924=FACE_OUTER_BOUND('',#1750,.T.);
#925=FACE_OUTER_BOUND('',#1751,.T.);
#926=FACE_OUTER_BOUND('',#1752,.T.);
#927=FACE_OUTER_BOUND('',#1753,.T.);
#928=FACE_OUTER_BOUND('',#1754,.T.);
#929=FACE_OUTER_BOUND('',#1755,.T.);
#930=FACE_OUTER_BOUND('',#1756,.T.);
#931=FACE_OUTER_BOUND('',#1757,.T.);
#932=FACE_OUTER_BOUND('',#1758,.T.);
#933=FACE_OUTER_BOUND('',#1759,.T.);
#934=FACE_OUTER_BOUND('',#1760,.T.);
#935=FACE_OUTER_BOUND('',#1761,.T.);
#936=FACE_OUTER_BOUND('',#1762,.T.);
#937=FACE_OUTER_BOUND('',#1763,.T.);
#938=FACE_OUTER_BOUND('',#1764,.T.);
#939=FACE_OUTER_BOUND('',#1765,.T.);
#940=FACE_OUTER_BOUND('',#1766,.T.);
#941=FACE_OUTER_BOUND('',#1767,.T.);
#942=FACE_OUTER_BOUND('',#1768,.T.);
#943=FACE_OUTER_BOUND('',#1769,.T.);
#944=FACE_OUTER_BOUND('',#1770,.T.);
#945=FACE_OUTER_BOUND('',#1771,.T.);
#946=FACE_OUTER_BOUND('',#1772,.T.);
#947=FACE_OUTER_BOUND('',#1773,.T.);
#948=FACE_OUTER_BOUND('',#1774,.T.);
#949=FACE_OUTER_BOUND('',#1775,.T.);
#950=FACE_OUTER_BOUND('',#1776,.T.);
#951=FACE_OUTER_BOUND('',#1777,.T.);
#952=FACE_OUTER_BOUND('',#1778,.T.);
#953=FACE_OUTER_BOUND('',#1779,.T.);
#954=FACE_OUTER_BOUND('',#1780,.T.);
#955=FACE_OUTER_BOUND('',#1781,.T.);
#956=FACE_OUTER_BOUND('',#1782,.T.);
#957=FACE_OUTER_BOUND('',#1783,.T.);
#958=FACE_OUTER_BOUND('',#1784,.T.);
#959=FACE_OUTER_BOUND('',#1785,.T.);
#960=FACE_OUTER_BOUND('',#1786,.T.);
#961=FACE_OUTER_BOUND('',#1787,.T.);
#962=FACE_OUTER_BOUND('',#1788,.T.);
#963=FACE_OUTER_BOUND('',#1789,.T.);
#964=FACE_OUTER_BOUND('',#1790,.T.);
#965=FACE_OUTER_BOUND('',#1791,.T.);
#966=FACE_OUTER_BOUND('',#1792,.T.);
#967=FACE_OUTER_BOUND('',#1793,.T.);
#968=FACE_OUTER_BOUND('',#1794,.T.);
#969=FACE_OUTER_BOUND('',#1795,.T.);
#970=FACE_OUTER_BOUND('',#1796,.T.);
#971=FACE_OUTER_BOUND('',#1797,.T.);
#972=FACE_OUTER_BOUND('',#1798,.T.);
#973=FACE_OUTER_BOUND('',#1799,.T.);
#974=FACE_OUTER_BOUND('',#1800,.T.);
#975=FACE_OUTER_BOUND('',#1801,.T.);
#976=FACE_OUTER_BOUND('',#1802,.T.);
#977=FACE_OUTER_BOUND('',#1803,.T.);
#978=FACE_OUTER_BOUND('',#1804,.T.);
#979=FACE_OUTER_BOUND('',#1805,.T.);
#980=FACE_OUTER_BOUND('',#1806,.T.);
#981=FACE_OUTER_BOUND('',#1807,.T.);
#982=FACE_OUTER_BOUND('',#1809,.T.);
#983=FACE_OUTER_BOUND('',#1810,.T.);
#984=FACE_OUTER_BOUND('',#1811,.T.);
#985=FACE_OUTER_BOUND('',#1812,.T.);
#986=FACE_OUTER_BOUND('',#1813,.T.);
#987=FACE_OUTER_BOUND('',#1814,.T.);
#988=FACE_OUTER_BOUND('',#1815,.T.);
#989=FACE_OUTER_BOUND('',#1816,.T.);
#990=FACE_OUTER_BOUND('',#1817,.T.);
#991=FACE_OUTER_BOUND('',#1818,.T.);
#992=FACE_OUTER_BOUND('',#1819,.T.);
#993=FACE_OUTER_BOUND('',#1821,.T.);
#1747=EDGE_LOOP('',(#11237,#11238,#11239,#11240));
#1748=EDGE_LOOP('',(#11241,#11242,#11243,#11244));
#1749=EDGE_LOOP('',(#11245,#11246,#11247,#11248));
#1750=EDGE_LOOP('',(#11249,#11250,#11251,#11252));
#1751=EDGE_LOOP('',(#11253,#11254,#11255,#11256));
#1752=EDGE_LOOP('',(#11257,#11258,#11259,#11260));
#1753=EDGE_LOOP('',(#11261,#11262,#11263,#11264));
#1754=EDGE_LOOP('',(#11265,#11266,#11267,#11268));
#1755=EDGE_LOOP('',(#11269,#11270,#11271,#11272));
#1756=EDGE_LOOP('',(#11273,#11274,#11275,#11276));
#1757=EDGE_LOOP('',(#11277,#11278,#11279,#11280));
#1758=EDGE_LOOP('',(#11281,#11282,#11283,#11284));
#1759=EDGE_LOOP('',(#11285,#11286,#11287,#11288));
#1760=EDGE_LOOP('',(#11289,#11290,#11291,#11292));
#1761=EDGE_LOOP('',(#11293,#11294,#11295,#11296));
#1762=EDGE_LOOP('',(#11297,#11298,#11299,#11300));
#1763=EDGE_LOOP('',(#11301,#11302,#11303,#11304));
#1764=EDGE_LOOP('',(#11305,#11306,#11307,#11308));
#1765=EDGE_LOOP('',(#11309,#11310,#11311,#11312));
#1766=EDGE_LOOP('',(#11313,#11314,#11315,#11316));
#1767=EDGE_LOOP('',(#11317,#11318,#11319,#11320));
#1768=EDGE_LOOP('',(#11321,#11322,#11323,#11324));
#1769=EDGE_LOOP('',(#11325,#11326,#11327,#11328));
#1770=EDGE_LOOP('',(#11329,#11330,#11331,#11332));
#1771=EDGE_LOOP('',(#11333,#11334,#11335,#11336));
#1772=EDGE_LOOP('',(#11337,#11338,#11339,#11340));
#1773=EDGE_LOOP('',(#11341,#11342,#11343,#11344));
#1774=EDGE_LOOP('',(#11345,#11346,#11347,#11348));
#1775=EDGE_LOOP('',(#11349,#11350,#11351,#11352));
#1776=EDGE_LOOP('',(#11353,#11354,#11355,#11356));
#1777=EDGE_LOOP('',(#11357,#11358,#11359,#11360));
#1778=EDGE_LOOP('',(#11361,#11362,#11363,#11364));
#1779=EDGE_LOOP('',(#11365,#11366,#11367,#11368));
#1780=EDGE_LOOP('',(#11369,#11370,#11371,#11372));
#1781=EDGE_LOOP('',(#11373,#11374,#11375,#11376));
#1782=EDGE_LOOP('',(#11377,#11378,#11379,#11380));
#1783=EDGE_LOOP('',(#11381,#11382,#11383,#11384));
#1784=EDGE_LOOP('',(#11385,#11386,#11387,#11388));
#1785=EDGE_LOOP('',(#11389,#11390,#11391,#11392));
#1786=EDGE_LOOP('',(#11393,#11394,#11395,#11396));
#1787=EDGE_LOOP('',(#11397,#11398,#11399,#11400));
#1788=EDGE_LOOP('',(#11401,#11402,#11403,#11404));
#1789=EDGE_LOOP('',(#11405,#11406,#11407,#11408));
#1790=EDGE_LOOP('',(#11409,#11410,#11411,#11412));
#1791=EDGE_LOOP('',(#11413,#11414,#11415,#11416));
#1792=EDGE_LOOP('',(#11417,#11418,#11419,#11420));
#1793=EDGE_LOOP('',(#11421,#11422,#11423,#11424));
#1794=EDGE_LOOP('',(#11425,#11426,#11427,#11428));
#1795=EDGE_LOOP('',(#11429,#11430,#11431,#11432));
#1796=EDGE_LOOP('',(#11433,#11434,#11435,#11436));
#1797=EDGE_LOOP('',(#11437,#11438,#11439,#11440));
#1798=EDGE_LOOP('',(#11441,#11442,#11443,#11444));
#1799=EDGE_LOOP('',(#11445,#11446,#11447,#11448));
#1800=EDGE_LOOP('',(#11449,#11450,#11451,#11452));
#1801=EDGE_LOOP('',(#11453,#11454,#11455,#11456));
#1802=EDGE_LOOP('',(#11457,#11458,#11459,#11460));
#1803=EDGE_LOOP('',(#11461,#11462,#11463,#11464));
#1804=EDGE_LOOP('',(#11465,#11466,#11467,#11468));
#1805=EDGE_LOOP('',(#11469,#11470,#11471,#11472,#11473,#11474,#11475,#11476,
#11477,#11478,#11479,#11480,#11481,#11482,#11483,#11484,#11485,#11486,#11487,
#11488,#11489,#11490,#11491,#11492,#11493,#11494,#11495,#11496,#11497,#11498,
#11499,#11500,#11501,#11502,#11503,#11504,#11505,#11506,#11507,#11508,#11509,
#11510,#11511,#11512,#11513,#11514,#11515,#11516,#11517,#11518,#11519,#11520,
#11521,#11522,#11523,#11524,#11525,#11526,#11527,#11528,#11529));
#1806=EDGE_LOOP('',(#11530,#11531,#11532,#11533,#11534,#11535,#11536,#11537,
#11538,#11539,#11540,#11541,#11542,#11543,#11544,#11545,#11546,#11547,#11548,
#11549,#11550,#11551,#11552,#11553,#11554,#11555,#11556,#11557,#11558,#11559,
#11560,#11561,#11562,#11563,#11564,#11565,#11566,#11567,#11568,#11569,#11570,
#11571,#11572,#11573,#11574,#11575,#11576,#11577,#11578,#11579,#11580,#11581,
#11582,#11583,#11584,#11585,#11586,#11587,#11588,#11589,#11590));
#1807=EDGE_LOOP('',(#11591,#11592,#11593,#11594,#11595,#11596,#11597,#11598));
#1808=EDGE_LOOP('',(#11599,#11600,#11601,#11602));
#1809=EDGE_LOOP('',(#11603,#11604,#11605,#11606));
#1810=EDGE_LOOP('',(#11607,#11608,#11609,#11610));
#1811=EDGE_LOOP('',(#11611,#11612,#11613,#11614));
#1812=EDGE_LOOP('',(#11615,#11616,#11617,#11618));
#1813=EDGE_LOOP('',(#11619,#11620,#11621,#11622,#11623,#11624));
#1814=EDGE_LOOP('',(#11625,#11626,#11627,#11628,#11629,#11630));
#1815=EDGE_LOOP('',(#11631,#11632,#11633,#11634));
#1816=EDGE_LOOP('',(#11635,#11636,#11637,#11638));
#1817=EDGE_LOOP('',(#11639,#11640,#11641,#11642));
#1818=EDGE_LOOP('',(#11643,#11644,#11645,#11646));
#1819=EDGE_LOOP('',(#11647,#11648,#11649,#11650,#11651,#11652,#11653,#11654));
#1820=EDGE_LOOP('',(#11655,#11656,#11657,#11658));
#1821=EDGE_LOOP('',(#11659,#11660,#11661,#11662));
#2287=CIRCLE('',#15372,5.13675);
#2288=CIRCLE('',#15400,5.13675);
#2289=CIRCLE('',#15402,6.11324999999999);
#2290=CIRCLE('',#15431,6.11325);
#2951=B_SPLINE_CURVE_WITH_KNOTS('',3,(#43271,#43272,#43273,#43274,#43275,
#43276,#43277,#43278,#43279,#43280,#43281,#43282,#43283,#43284,#43285,#43286,
#43287,#43288,#43289,#43290,#43291,#43292,#43293,#43294,#43295,#43296,#43297,
#43298),.UNSPECIFIED.,.F.,.F.,(4,3,3,3,3,3,3,3,3,4),(177.238751742006,177.553807102306,
178.05255375147,178.551300400634,179.050047049798,179.548793698961,180.047540348125,
180.546286997289,181.045033646453,181.543780295616),.UNSPECIFIED.);
#2952=B_SPLINE_CURVE_WITH_KNOTS('',3,(#43301,#43302,#43303,#43304,#43305,
#43306,#43307,#43308,#43309,#43310,#43311,#43312,#43313,#43314,#43315,#43316,
#43317,#43318,#43319,#43320,#43321,#43322,#43323,#43324,#43325,#43326,#43327,
#43328,#43329,#43330,#43331,#43332,#43333,#43334,#43335,#43336,#43337,#43338,
#43339,#43340),.UNSPECIFIED.,.F.,.F.,(4,3,3,3,3,3,3,3,3,3,3,3,3,4),(-179.519580205131,
-179.050047049798,-178.551300400634,-178.05255375147,-177.553807102306,
-177.055060453142,-176.556313803979,-176.057567154815,-175.558820505651,
-175.060073856487,-174.561327207324,-174.06258055816,-173.563833908996,
-173.502232896947),.UNSPECIFIED.);
#2953=B_SPLINE_CURVE_WITH_KNOTS('',3,(#43345,#43346,#43347,#43348,#43349,
#43350,#43351,#43352,#43353,#43354,#43355,#43356,#43357,#43358,#43359,#43360,
#43361,#43362,#43363,#43364,#43365,#43366,#43367,#43368,#43369,#43370,#43371,
#43372,#43373,#43374,#43375,#43376,#43377,#43378,#43379,#43380,#43381,#43382,
#43383,#43384,#43385,#43386,#43387),.UNSPECIFIED.,.F.,.F.,(4,3,3,3,3,3,
3,3,3,3,3,3,3,3,4),(170.955566434826,171.070100663177,171.568847312341,
172.067593961505,172.566340610668,173.065087259832,173.563833908996,174.06258055816,
174.561327207323,175.060073856487,175.558820505651,176.057567154815,176.556313803979,
177.055060453142,177.238751742006),.UNSPECIFIED.);
#2954=B_SPLINE_CURVE_WITH_KNOTS('',3,(#43388,#43389,#43390,#43391,#43392,
#43393,#43394,#43395,#43396,#43397,#43398,#43399,#43400,#43401,#43402,#43403,
#43404,#43405,#43406,#43407,#43408,#43409,#43410,#43411,#43412,#43413,#43414,
#43415,#43416,#43417,#43418,#43419,#43420,#43421,#43422,#43423,#43424,#43425,
#43426,#43427),.UNSPECIFIED.,.F.,.F.,(4,3,3,3,3,3,3,3,3,3,3,3,3,4),(-173.502232896947,
-173.065087259832,-172.566340610668,-172.067593961505,-171.568847312341,
-171.070100663177,-170.571354014013,-170.072607364849,-169.573860715686,
-169.075114066522,-168.576367417358,-168.077620768194,-167.578874119031,
-167.219047589767),.UNSPECIFIED.);
#2955=B_SPLINE_CURVE_WITH_KNOTS('',3,(#43432,#43433,#43434,#43435,#43436,
#43437,#43438,#43439,#43440,#43441,#43442,#43443,#43444,#43445,#43446,#43447,
#43448,#43449,#43450,#43451,#43452,#43453,#43454,#43455,#43456,#43457,#43458,
#43459,#43460,#43461,#43462,#43463,#43464,#43465,#43466,#43467,#43468,#43469,
#43470,#43471),.UNSPECIFIED.,.F.,.F.,(4,3,3,3,3,3,3,3,3,3,3,3,3,4),(164.672381127646,
165.085140873212,165.583887522375,166.082634171539,166.581380820703,167.080127469867,
167.578874119031,168.077620768194,168.576367417358,169.075114066522,169.573860715686,
170.072607364849,170.571354014013,170.955566434826),.UNSPECIFIED.);
#2956=B_SPLINE_CURVE_WITH_KNOTS('',3,(#43472,#43473,#43474,#43475,#43476,
#43477,#43478,#43479,#43480,#43481,#43482,#43483,#43484,#43485,#43486,#43487,
#43488,#43489,#43490,#43491,#43492,#43493,#43494,#43495,#43496,#43497,#43498,
#43499,#43500,#43501,#43502,#43503,#43504,#43505,#43506,#43507,#43508,#43509,
#43510,#43511,#43512,#43513,#43514),.UNSPECIFIED.,.F.,.F.,(4,3,3,3,3,3,
3,3,3,3,3,3,3,3,4),(-167.219047589767,-167.080127469867,-166.581380820703,
-166.082634171539,-165.583887522375,-165.085140873212,-164.586394224048,
-164.087647574884,-163.58890092572,-163.090154276557,-162.591407627393,
-162.092660978229,-161.593914329065,-161.095167679901,-160.935862282588),
 .UNSPECIFIED.);
#2957=B_SPLINE_CURVE_WITH_KNOTS('',3,(#43519,#43520,#43521,#43522,#43523,
#43524,#43525,#43526,#43527,#43528,#43529,#43530,#43531,#43532,#43533,#43534,
#43535,#43536,#43537,#43538,#43539,#43540,#43541,#43542,#43543,#43544,#43545,
#43546,#43547,#43548,#43549,#43550,#43551,#43552,#43553,#43554,#43555,#43556,
#43557,#43558,#43559,#43560,#43561),.UNSPECIFIED.,.F.,.F.,(4,3,3,3,3,3,
3,3,3,3,3,3,3,3,4),(158.389195820467,158.601434434082,159.100181083246,
159.59892773241,160.097674381574,160.596421030738,161.095167679901,161.593914329065,
162.092660978229,162.591407627393,163.090154276556,163.58890092572,164.087647574884,
164.586394224048,164.672381127646),.UNSPECIFIED.);
#2958=B_SPLINE_CURVE_WITH_KNOTS('',3,(#43562,#43563,#43564,#43565,#43566,
#43567,#43568,#43569,#43570,#43571,#43572,#43573,#43574,#43575,#43576,#43577,
#43578,#43579,#43580,#43581,#43582,#43583,#43584,#43585,#43586,#43587,#43588,
#43589,#43590,#43591,#43592,#43593,#43594,#43595,#43596,#43597,#43598,#43599,
#43600,#43601),.UNSPECIFIED.,.F.,.F.,(4,3,3,3,3,3,3,3,3,3,3,3,3,4),(-160.935862282588,
-160.596421030738,-160.097674381574,-159.59892773241,-159.100181083246,
-158.601434434082,-158.102687784919,-157.603941135755,-157.105194486591,
-156.606447837427,-156.107701188264,-155.6089545391,-155.110207889936,-154.652676975408),
 .UNSPECIFIED.);
#2959=B_SPLINE_CURVE_WITH_KNOTS('',3,(#43606,#43607,#43608,#43609,#43610,
#43611,#43612,#43613,#43614,#43615,#43616,#43617,#43618,#43619,#43620,#43621,
#43622,#43623,#43624,#43625,#43626,#43627,#43628,#43629,#43630,#43631,#43632,
#43633,#43634,#43635,#43636,#43637,#43638,#43639,#43640,#43641,#43642,#43643,
#43644,#43645,#43646,#43647,#43648),.UNSPECIFIED.,.F.,.F.,(4,3,3,3,3,3,
3,3,3,3,3,3,3,3,4),(152.106010513287,152.117727994953,152.616474644117,
153.115221293281,153.613967942445,154.112714591608,154.611461240772,155.110207889936,
155.6089545391,156.107701188264,156.606447837427,157.105194486591,157.603941135755,
158.102687784919,158.389195820467),.UNSPECIFIED.);
#2960=B_SPLINE_CURVE_WITH_KNOTS('',3,(#43649,#43650,#43651,#43652,#43653,
#43654,#43655,#43656,#43657,#43658,#43659,#43660,#43661,#43662,#43663,#43664,
#43665,#43666,#43667,#43668,#43669,#43670,#43671,#43672,#43673,#43674,#43675,
#43676,#43677,#43678,#43679,#43680,#43681,#43682,#43683,#43684,#43685,#43686,
#43687,#43688,#43689,#43690,#43691),.UNSPECIFIED.,.F.,.F.,(4,3,3,3,3,3,
3,3,3,3,3,3,3,3,4),(-154.652676975408,-154.611461240772,-154.112714591608,
-153.613967942445,-153.115221293281,-152.616474644117,-152.117727994953,
-151.61898134579,-151.120234696626,-150.621488047462,-150.122741398298,
-149.623994749134,-149.125248099971,-148.626501450807,-148.369491668229),
 .UNSPECIFIED.);
#2961=B_SPLINE_CURVE_WITH_KNOTS('',3,(#43696,#43697,#43698,#43699,#43700,
#43701,#43702,#43703,#43704,#43705,#43706,#43707,#43708,#43709,#43710,#43711,
#43712,#43713,#43714,#43715,#43716,#43717,#43718,#43719,#43720,#43721,#43722,
#43723,#43724,#43725,#43726,#43727,#43728,#43729,#43730,#43731,#43732,#43733,
#43734,#43735),.UNSPECIFIED.,.F.,.F.,(4,3,3,3,3,3,3,3,3,3,3,3,3,4),(145.822825206108,
146.132768204988,146.631514854152,147.130261503315,147.629008152479,148.127754801643,
148.626501450807,149.125248099971,149.623994749134,150.122741398298,150.621488047462,
151.120234696626,151.61898134579,152.106010513287),.UNSPECIFIED.);
#2962=B_SPLINE_CURVE_WITH_KNOTS('',3,(#43736,#43737,#43738,#43739,#43740,
#43741,#43742,#43743,#43744,#43745,#43746,#43747,#43748,#43749,#43750,#43751,
#43752,#43753,#43754,#43755,#43756,#43757,#43758,#43759,#43760,#43761,#43762,
#43763,#43764,#43765,#43766,#43767,#43768,#43769,#43770,#43771,#43772,#43773,
#43774,#43775,#43776,#43777,#43778),.UNSPECIFIED.,.F.,.F.,(4,3,3,3,3,3,
3,3,3,3,3,3,3,3,4),(-148.369491668229,-148.127754801643,-147.629008152479,
-147.130261503316,-146.631514854152,-146.132768204988,-145.634021555824,
-145.13527490666,-144.636528257497,-144.137781608333,-143.639034959169,
-143.140288310005,-142.641541660841,-142.142795011678,-142.086306361049),
 .UNSPECIFIED.);
#2963=B_SPLINE_CURVE_WITH_KNOTS('',3,(#43783,#43784,#43785,#43786,#43787,
#43788,#43789,#43790,#43791,#43792,#43793,#43794,#43795,#43796,#43797,#43798,
#43799,#43800,#43801,#43802,#43803,#43804,#43805,#43806,#43807,#43808,#43809,
#43810,#43811,#43812,#43813,#43814,#43815,#43816,#43817,#43818,#43819,#43820,
#43821,#43822,#43823,#43824,#43825),.UNSPECIFIED.,.F.,.F.,(4,3,3,3,3,3,
3,3,3,3,3,3,3,3,4),(139.539639898928,139.649061765859,140.147808415023,
140.646555064186,141.14530171335,141.644048362514,142.142795011678,142.641541660841,
143.140288310005,143.639034959169,144.137781608333,144.636528257497,145.13527490666,
145.634021555824,145.822825206108),.UNSPECIFIED.);
#2964=B_SPLINE_CURVE_WITH_KNOTS('',3,(#43826,#43827,#43828,#43829,#43830,
#43831,#43832,#43833,#43834,#43835,#43836,#43837,#43838,#43839,#43840,#43841,
#43842,#43843,#43844,#43845,#43846,#43847,#43848,#43849,#43850,#43851,#43852,
#43853,#43854,#43855,#43856,#43857,#43858,#43859,#43860,#43861,#43862,#43863,
#43864,#43865),.UNSPECIFIED.,.F.,.F.,(4,3,3,3,3,3,3,3,3,3,3,3,3,4),(-142.086306361049,
-141.644048362514,-141.14530171335,-140.646555064186,-140.147808415023,
-139.649061765859,-139.150315116695,-138.651568467531,-138.152821818367,
-137.654075169204,-137.15532852004,-136.656581870876,-136.157835221712,
-135.80312105387),.UNSPECIFIED.);
#2965=B_SPLINE_CURVE_WITH_KNOTS('',3,(#43870,#43871,#43872,#43873,#43874,
#43875,#43876,#43877,#43878,#43879,#43880,#43881,#43882,#43883,#43884,#43885,
#43886,#43887,#43888,#43889,#43890,#43891,#43892,#43893,#43894,#43895,#43896,
#43897,#43898,#43899,#43900,#43901,#43902,#43903,#43904,#43905,#43906,#43907,
#43908,#43909),.UNSPECIFIED.,.F.,.F.,(4,3,3,3,3,3,3,3,3,3,3,3,3,4),(133.256454591749,
133.664101975893,134.162848625057,134.661595274221,135.160341923385,135.659088572549,
136.157835221712,136.656581870876,137.15532852004,137.654075169204,138.152821818367,
138.651568467531,139.150315116695,139.539639898928),.UNSPECIFIED.);
#2966=B_SPLINE_CURVE_WITH_KNOTS('',3,(#43910,#43911,#43912,#43913,#43914,
#43915,#43916,#43917,#43918,#43919,#43920,#43921,#43922,#43923,#43924,#43925,
#43926,#43927,#43928,#43929,#43930,#43931,#43932,#43933,#43934,#43935,#43936,
#43937,#43938,#43939,#43940,#43941,#43942,#43943,#43944,#43945,#43946,#43947,
#43948,#43949,#43950,#43951,#43952),.UNSPECIFIED.,.F.,.F.,(4,3,3,3,3,3,
3,3,3,3,3,3,3,3,4),(-135.80312105387,-135.659088572549,-135.160341923385,
-134.661595274221,-134.162848625057,-133.664101975893,-133.16535532673,
-132.666608677566,-132.167862028402,-131.669115379238,-131.170368730075,
-130.671622080911,-130.172875431747,-129.674128782583,-129.51993574669),
 .UNSPECIFIED.);
#2967=B_SPLINE_CURVE_WITH_KNOTS('',3,(#43957,#43958,#43959,#43960,#43961,
#43962,#43963,#43964,#43965,#43966,#43967,#43968,#43969,#43970,#43971,#43972,
#43973,#43974,#43975,#43976,#43977,#43978,#43979,#43980,#43981,#43982,#43983,
#43984,#43985,#43986,#43987,#43988,#43989,#43990,#43991,#43992,#43993,#43994,
#43995,#43996,#43997,#43998,#43999),.UNSPECIFIED.,.F.,.F.,(4,3,3,3,3,3,
3,3,3,3,3,3,3,3,4),(126.973269284569,127.180395536764,127.679142185928,
128.177888835092,128.676635484256,129.175382133419,129.674128782583,130.172875431747,
130.671622080911,131.170368730074,131.669115379238,132.167862028402,132.666608677566,
133.16535532673,133.256454591749),.UNSPECIFIED.);
#2968=B_SPLINE_CURVE_WITH_KNOTS('',3,(#44000,#44001,#44002,#44003,#44004,
#44005,#44006,#44007,#44008,#44009,#44010,#44011,#44012,#44013,#44014,#44015,
#44016,#44017,#44018,#44019,#44020,#44021,#44022,#44023,#44024,#44025,#44026,
#44027,#44028,#44029,#44030,#44031,#44032,#44033,#44034,#44035,#44036,#44037,
#44038,#44039),.UNSPECIFIED.,.F.,.F.,(4,3,3,3,3,3,3,3,3,3,3,3,3,4),(-129.51993574669,
-129.175382133419,-128.676635484256,-128.177888835092,-127.679142185928,
-127.180395536764,-126.6816488876,-126.182902238437,-125.684155589273,-125.185408940109,
-124.686662290945,-124.187915641782,-123.689168992618,-123.23675043951),
 .UNSPECIFIED.);
#2969=B_SPLINE_CURVE_WITH_KNOTS('',3,(#44044,#44045,#44046,#44047,#44048,
#44049,#44050,#44051,#44052,#44053,#44054,#44055,#44056,#44057,#44058,#44059,
#44060,#44061,#44062,#44063,#44064,#44065,#44066,#44067,#44068,#44069,#44070,
#44071,#44072,#44073,#44074,#44075,#44076,#44077,#44078,#44079,#44080,#44081,
#44082,#44083,#44084,#44085,#44086),.UNSPECIFIED.,.F.,.F.,(4,3,3,3,3,3,
3,3,3,3,3,3,3,3,4),(120.690083977389,120.696689097635,121.195435746799,
121.694182395963,122.192929045126,122.69167569429,123.190422343454,123.689168992618,
124.187915641782,124.686662290945,125.185408940109,125.684155589273,126.182902238437,
126.6816488876,126.973269284569),.UNSPECIFIED.);
#2970=B_SPLINE_CURVE_WITH_KNOTS('',3,(#44087,#44088,#44089,#44090,#44091,
#44092,#44093,#44094,#44095,#44096,#44097,#44098,#44099,#44100,#44101,#44102,
#44103,#44104,#44105,#44106,#44107,#44108,#44109,#44110,#44111,#44112,#44113,
#44114,#44115,#44116,#44117,#44118,#44119,#44120,#44121,#44122,#44123,#44124,
#44125,#44126,#44127,#44128,#44129),.UNSPECIFIED.,.F.,.F.,(4,3,3,3,3,3,
3,3,3,3,3,3,3,3,4),(-123.23675043951,-123.190422343454,-122.69167569429,
-122.192929045126,-121.694182395963,-121.195435746799,-120.696689097635,
-120.197942448471,-119.699195799308,-119.200449150144,-118.70170250098,
-118.202955851816,-117.704209202652,-117.205462553489,-116.953565132331),
 .UNSPECIFIED.);
#2971=B_SPLINE_CURVE_WITH_KNOTS('',3,(#44134,#44135,#44136,#44137,#44138,
#44139,#44140,#44141,#44142,#44143,#44144,#44145,#44146,#44147,#44148,#44149,
#44150,#44151,#44152,#44153,#44154,#44155,#44156,#44157,#44158,#44159,#44160,
#44161,#44162,#44163,#44164,#44165,#44166,#44167,#44168,#44169,#44170,#44171,
#44172,#44173),.UNSPECIFIED.,.F.,.F.,(4,3,3,3,3,3,3,3,3,3,3,3,3,4),(114.40689867021,
114.71172930767,115.210475956833,115.709222605997,116.207969255161,116.706715904325,
117.205462553489,117.704209202652,118.202955851816,118.70170250098,119.200449150144,
119.699195799308,120.197942448471,120.690083977389),.UNSPECIFIED.);
#2972=B_SPLINE_CURVE_WITH_KNOTS('',3,(#44174,#44175,#44176,#44177,#44178,
#44179,#44180,#44181,#44182,#44183,#44184,#44185,#44186,#44187,#44188,#44189,
#44190,#44191,#44192,#44193,#44194,#44195,#44196,#44197,#44198,#44199,#44200,
#44201,#44202,#44203,#44204,#44205,#44206,#44207,#44208,#44209,#44210,#44211,
#44212,#44213,#44214,#44215,#44216),.UNSPECIFIED.,.F.,.F.,(4,3,3,3,3,3,
3,3,3,3,3,3,3,3,4),(-116.953565132331,-116.706715904325,-116.207969255161,
-115.709222605997,-115.210475956834,-114.71172930767,-114.212982658506,
-113.714236009342,-113.215489360178,-112.716742711015,-112.217996061851,
-111.719249412687,-111.220502763523,-110.721756114359,-110.670379825151),
 .UNSPECIFIED.);
#2973=B_SPLINE_CURVE_WITH_KNOTS('',3,(#44221,#44222,#44223,#44224,#44225,
#44226,#44227,#44228,#44229,#44230,#44231,#44232,#44233,#44234,#44235,#44236,
#44237,#44238,#44239,#44240,#44241,#44242,#44243,#44244,#44245,#44246,#44247,
#44248,#44249,#44250,#44251,#44252,#44253,#44254,#44255,#44256,#44257,#44258,
#44259,#44260,#44261,#44262,#44263),.UNSPECIFIED.,.F.,.F.,(4,3,3,3,3,3,
3,3,3,3,3,3,3,3,4),(108.12371336303,108.228022868541,108.726769517704,109.225516166868,
109.724262816032,110.223009465196,110.721756114359,111.220502763523,111.719249412687,
112.217996061851,112.716742711015,113.215489360178,113.714236009342,114.212982658506,
114.40689867021),.UNSPECIFIED.);
#2974=B_SPLINE_CURVE_WITH_KNOTS('',3,(#44264,#44265,#44266,#44267,#44268,
#44269,#44270,#44271,#44272,#44273,#44274,#44275,#44276,#44277,#44278,#44279,
#44280,#44281,#44282,#44283,#44284,#44285,#44286,#44287,#44288,#44289,#44290,
#44291,#44292,#44293,#44294,#44295,#44296,#44297,#44298,#44299,#44300,#44301,
#44302,#44303),.UNSPECIFIED.,.F.,.F.,(4,3,3,3,3,3,3,3,3,3,3,3,3,4),(-110.670379825151,
-110.223009465196,-109.724262816032,-109.225516166868,-108.726769517704,
-108.228022868541,-107.729276219377,-107.230529570213,-106.731782921049,
-106.233036271885,-105.734289622722,-105.235542973558,-104.736796324394,
-104.387194517972),.UNSPECIFIED.);
#2975=B_SPLINE_CURVE_WITH_KNOTS('',3,(#44308,#44309,#44310,#44311,#44312,
#44313,#44314,#44315,#44316,#44317,#44318,#44319,#44320,#44321,#44322,#44323,
#44324,#44325,#44326,#44327,#44328,#44329,#44330,#44331,#44332,#44333,#44334,
#44335,#44336,#44337,#44338,#44339,#44340,#44341,#44342,#44343,#44344,#44345,
#44346,#44347),.UNSPECIFIED.,.F.,.F.,(4,3,3,3,3,3,3,3,3,3,3,3,3,4),(101.840528055851,
102.243063078575,102.741809727739,103.240556376903,103.739303026067,104.23804967523,
104.736796324394,105.235542973558,105.734289622722,106.233036271885,106.731782921049,
107.230529570213,107.729276219377,108.12371336303),.UNSPECIFIED.);
#2976=B_SPLINE_CURVE_WITH_KNOTS('',3,(#44348,#44349,#44350,#44351,#44352,
#44353,#44354,#44355,#44356,#44357,#44358,#44359,#44360,#44361,#44362,#44363,
#44364,#44365,#44366,#44367,#44368,#44369,#44370,#44371,#44372,#44373,#44374,
#44375,#44376,#44377,#44378,#44379,#44380,#44381,#44382,#44383,#44384,#44385,
#44386,#44387,#44388,#44389,#44390),.UNSPECIFIED.,.F.,.F.,(4,3,3,3,3,3,
3,3,3,3,3,3,3,3,4),(-104.387194517972,-104.23804967523,-103.739303026067,
-103.240556376903,-102.741809727739,-102.243063078575,-101.744316429411,
-101.245569780248,-100.746823131084,-100.24807648192,-99.7493298327563,
-99.2505831835925,-98.7518365344287,-98.2530898852649,-98.104009210792),
 .UNSPECIFIED.);
#2977=B_SPLINE_CURVE_WITH_KNOTS('',3,(#44395,#44396,#44397,#44398,#44399,
#44400,#44401,#44402,#44403,#44404,#44405,#44406,#44407,#44408,#44409,#44410,
#44411,#44412,#44413,#44414,#44415,#44416,#44417,#44418,#44419,#44420,#44421,
#44422,#44423,#44424,#44425,#44426,#44427,#44428,#44429,#44430,#44431,#44432,
#44433,#44434,#44435,#44436,#44437),.UNSPECIFIED.,.F.,.F.,(4,3,3,3,3,3,
3,3,3,3,3,3,3,3,4),(95.557342748671,95.759356639446,96.2581032886098,96.7568499377736,
97.2555965869374,97.7543432361011,98.2530898852649,98.7518365344287,99.2505831835925,
99.7493298327563,100.24807648192,100.746823131084,101.245569780248,101.744316429411,
101.840528055851),.UNSPECIFIED.);
#2978=B_SPLINE_CURVE_WITH_KNOTS('',3,(#44438,#44439,#44440,#44441,#44442,
#44443,#44444,#44445,#44446,#44447,#44448,#44449,#44450,#44451,#44452,#44453,
#44454,#44455,#44456,#44457,#44458,#44459,#44460,#44461,#44462,#44463,#44464,
#44465,#44466,#44467,#44468,#44469,#44470,#44471,#44472,#44473,#44474,#44475,
#44476,#44477),.UNSPECIFIED.,.F.,.F.,(4,3,3,3,3,3,3,3,3,3,3,3,3,4),(-98.104009210792,
-97.7543432361011,-97.2555965869374,-96.7568499377736,-96.2581032886098,
-95.759356639446,-95.2606099902822,-94.7618633411185,-94.2631166919547,
-93.7643700427909,-93.2656233936271,-92.7668767444633,-92.2681300952996,
-91.8208239036124),.UNSPECIFIED.);
#2979=B_SPLINE_CURVE_WITH_KNOTS('',3,(#44482,#44483,#44484,#44485,#44486,
#44487,#44488,#44489,#44490,#44491,#44492,#44493,#44494,#44495,#44496,#44497,
#44498,#44499,#44500,#44501,#44502,#44503,#44504,#44505,#44506,#44507,#44508,
#44509,#44510,#44511,#44512,#44513,#44514,#44515,#44516,#44517,#44518,#44519,
#44520,#44521),.UNSPECIFIED.,.F.,.F.,(4,3,3,3,3,3,3,3,3,3,3,3,3,4),(89.2741574414915,
89.7743968494806,90.2731434986444,90.7718901478082,91.270636796972,91.7693834461358,
92.2681300952995,92.7668767444633,93.2656233936271,93.7643700427909,94.2631166919547,
94.7618633411184,95.2606099902822,95.557342748671),.UNSPECIFIED.);
#2980=B_SPLINE_CURVE_WITH_KNOTS('',3,(#44522,#44523,#44524,#44525,#44526,
#44527,#44528,#44529,#44530,#44531,#44532,#44533,#44534,#44535,#44536,#44537,
#44538,#44539,#44540,#44541,#44542,#44543,#44544,#44545,#44546,#44547,#44548,
#44549,#44550,#44551,#44552,#44553,#44554,#44555,#44556,#44557,#44558,#44559,
#44560,#44561,#44562,#44563,#44564),.UNSPECIFIED.,.F.,.F.,(4,3,3,3,3,3,
3,3,3,3,3,3,3,3,4),(-91.8208239036124,-91.7693834461358,-91.270636796972,
-90.7718901478082,-90.2731434986444,-89.7743968494807,-89.2756502003169,
-88.7769035511531,-88.2781569019893,-87.7794102528255,-87.2806636036618,
-86.781916954498,-86.2831703053342,-85.7844236561704,-85.5376385964328),
 .UNSPECIFIED.);
#2981=B_SPLINE_CURVE_WITH_KNOTS('',3,(#44569,#44570,#44571,#44572,#44573,
#44574,#44575,#44576,#44577,#44578,#44579,#44580,#44581,#44582,#44583,#44584,
#44585,#44586,#44587,#44588,#44589,#44590,#44591,#44592,#44593,#44594,#44595,
#44596,#44597,#44598,#44599,#44600,#44601,#44602,#44603,#44604,#44605,#44606,
#44607,#44608),.UNSPECIFIED.,.F.,.F.,(4,3,3,3,3,3,3,3,3,3,3,3,3,4),(82.9909721343118,
83.2906904103515,83.7894370595153,84.288183708679,84.7869303578428,85.2856770070066,
85.7844236561704,86.2831703053342,86.7819169544979,87.2806636036617,87.7794102528255,
88.2781569019893,88.7769035511531,89.2741574414915),.UNSPECIFIED.);
#2982=B_SPLINE_CURVE_WITH_KNOTS('',3,(#44609,#44610,#44611,#44612,#44613,
#44614,#44615,#44616,#44617,#44618,#44619,#44620,#44621,#44622,#44623,#44624,
#44625,#44626,#44627,#44628,#44629,#44630,#44631,#44632,#44633,#44634,#44635,
#44636,#44637,#44638,#44639,#44640,#44641,#44642,#44643,#44644,#44645,#44646,
#44647,#44648,#44649,#44650,#44651),.UNSPECIFIED.,.F.,.F.,(4,3,3,3,3,3,
3,3,3,3,3,3,3,3,4),(-85.5376385964328,-85.2856770070066,-84.7869303578428,
-84.2881837086791,-83.7894370595153,-83.2906904103515,-82.7919437611877,
-82.2931971120239,-81.7944504628602,-81.2957038136964,-80.7969571645326,
-80.2982105153688,-79.799463866205,-79.3007172170413,-79.2544532892532),
 .UNSPECIFIED.);
#2983=B_SPLINE_CURVE_WITH_KNOTS('',3,(#44656,#44657,#44658,#44659,#44660,
#44661,#44662,#44663,#44664,#44665,#44666,#44667,#44668,#44669,#44670,#44671,
#44672,#44673,#44674,#44675,#44676,#44677,#44678,#44679,#44680,#44681,#44682,
#44683,#44684,#44685,#44686,#44687,#44688,#44689,#44690,#44691,#44692,#44693,
#44694,#44695,#44696,#44697,#44698),.UNSPECIFIED.,.F.,.F.,(4,3,3,3,3,3,
3,3,3,3,3,3,3,3,4),(76.7077868271323,76.8069839712223,77.3057306203861,
77.8044772695499,78.3032239187137,78.8019705678775,79.3007172170412,79.799463866205,
80.2982105153688,80.7969571645326,81.2957038136963,81.7944504628601,82.2931971120239,
82.7919437611877,82.9909721343118),.UNSPECIFIED.);
#2984=B_SPLINE_CURVE_WITH_KNOTS('',3,(#44699,#44700,#44701,#44702,#44703,
#44704,#44705,#44706,#44707,#44708,#44709,#44710,#44711,#44712,#44713,#44714,
#44715,#44716,#44717,#44718,#44719,#44720,#44721,#44722,#44723,#44724,#44725,
#44726,#44727,#44728,#44729,#44730,#44731,#44732,#44733,#44734,#44735,#44736,
#44737,#44738),.UNSPECIFIED.,.F.,.F.,(4,3,3,3,3,3,3,3,3,3,3,3,3,4),(-79.2544532892532,
-78.8019705678775,-78.3032239187137,-77.8044772695499,-77.3057306203861,
-76.8069839712224,-76.3082373220585,-75.8094906728948,-75.310744023731,
-74.8119973745672,-74.3132507254034,-73.8145040762396,-73.3157574270759,
-72.9712679820736),.UNSPECIFIED.);
#2985=B_SPLINE_CURVE_WITH_KNOTS('',3,(#44743,#44744,#44745,#44746,#44747,
#44748,#44749,#44750,#44751,#44752,#44753,#44754,#44755,#44756,#44757,#44758,
#44759,#44760,#44761,#44762,#44763,#44764,#44765,#44766,#44767,#44768,#44769,
#44770,#44771,#44772,#44773,#44774,#44775,#44776,#44777,#44778,#44779,#44780,
#44781,#44782),.UNSPECIFIED.,.F.,.F.,(4,3,3,3,3,3,3,3,3,3,3,3,3,4),(70.4246015199527,
70.8220241812569,71.3207708304207,71.8195174795845,72.3182641287483,72.8170107779121,
73.3157574270759,73.8145040762396,74.3132507254034,74.8119973745672,75.310744023731,
75.8094906728948,76.3082373220586,76.7077868271323),.UNSPECIFIED.);
#2986=B_SPLINE_CURVE_WITH_KNOTS('',3,(#44783,#44784,#44785,#44786,#44787,
#44788,#44789,#44790,#44791,#44792,#44793,#44794,#44795,#44796,#44797,#44798,
#44799,#44800,#44801,#44802,#44803,#44804,#44805,#44806,#44807,#44808,#44809,
#44810,#44811,#44812,#44813,#44814,#44815,#44816,#44817,#44818,#44819,#44820,
#44821,#44822,#44823,#44824,#44825),.UNSPECIFIED.,.F.,.F.,(4,3,3,3,3,3,
3,3,3,3,3,3,3,3,4),(-72.9712679820736,-72.8170107779121,-72.3182641287483,
-71.8195174795845,-71.3207708304207,-70.8220241812569,-70.3232775320932,
-69.8245308829294,-69.3257842337656,-68.8270375846018,-68.328290935438,
-67.8295442862743,-67.3307976371105,-66.8320509879467,-66.688082674894),
 .UNSPECIFIED.);
#2987=B_SPLINE_CURVE_WITH_KNOTS('',3,(#44830,#44831,#44832,#44833,#44834,
#44835,#44836,#44837,#44838,#44839,#44840,#44841,#44842,#44843,#44844,#44845,
#44846,#44847,#44848,#44849,#44850,#44851,#44852,#44853,#44854,#44855,#44856,
#44857,#44858,#44859,#44860,#44861,#44862,#44863,#44864,#44865,#44866,#44867,
#44868,#44869,#44870,#44871,#44872),.UNSPECIFIED.,.F.,.F.,(4,3,3,3,3,3,
3,3,3,3,3,3,3,3,4),(64.1414162127731,64.3383177421278,64.8370643912916,
65.3358110404554,65.8345576896191,66.3333043387829,66.8320509879467,67.3307976371105,
67.8295442862743,68.328290935438,68.8270375846018,69.3257842337656,69.8245308829294,
70.3232775320932,70.4246015199527),.UNSPECIFIED.);
#2988=B_SPLINE_CURVE_WITH_KNOTS('',3,(#44873,#44874,#44875,#44876,#44877,
#44878,#44879,#44880,#44881,#44882,#44883,#44884,#44885,#44886,#44887,#44888,
#44889,#44890,#44891,#44892,#44893,#44894,#44895,#44896,#44897,#44898,#44899,
#44900,#44901,#44902,#44903,#44904,#44905,#44906,#44907,#44908,#44909,#44910,
#44911,#44912),.UNSPECIFIED.,.F.,.F.,(4,3,3,3,3,3,3,3,3,3,3,3,3,4),(-66.688082674894,
-66.3333043387829,-65.8345576896191,-65.3358110404554,-64.8370643912916,
-64.3383177421278,-63.839571092964,-63.3408244438002,-62.8420777946365,
-62.3433311454727,-61.8445844963089,-61.3458378471451,-60.8470911979813,
-60.4048973677144),.UNSPECIFIED.);
#2989=B_SPLINE_CURVE_WITH_KNOTS('',3,(#44917,#44918,#44919,#44920,#44921,
#44922,#44923,#44924,#44925,#44926,#44927,#44928,#44929,#44930,#44931,#44932,
#44933,#44934,#44935,#44936,#44937,#44938,#44939,#44940,#44941,#44942,#44943,
#44944,#44945,#44946,#44947,#44948,#44949,#44950,#44951,#44952,#44953,#44954,
#44955,#44956),.UNSPECIFIED.,.F.,.F.,(4,3,3,3,3,3,3,3,3,3,3,3,3,4),(57.8582309055935,
58.3533579521624,58.8521046013262,59.35085125049,59.8495978996538,60.3483445488176,
60.8470911979813,61.3458378471451,61.8445844963089,62.3433311454727,62.8420777946365,
63.3408244438002,63.839571092964,64.1414162127731),.UNSPECIFIED.);
#2990=B_SPLINE_CURVE_WITH_KNOTS('',3,(#44957,#44958,#44959,#44960,#44961,
#44962,#44963,#44964,#44965,#44966,#44967,#44968,#44969,#44970,#44971,#44972,
#44973,#44974,#44975,#44976,#44977,#44978,#44979,#44980,#44981,#44982,#44983,
#44984,#44985,#44986,#44987,#44988,#44989,#44990,#44991,#44992,#44993,#44994,
#44995,#44996,#44997,#44998,#44999),.UNSPECIFIED.,.F.,.F.,(4,3,3,3,3,3,
3,3,3,3,3,3,3,3,4),(-60.4048973677144,-60.3483445488176,-59.8495978996538,
-59.35085125049,-58.8521046013262,-58.3533579521624,-57.8546113029987,-57.3558646538349,
-56.8571180046711,-56.3583713555073,-55.8596247063435,-55.3608780571797,
-54.862131408016,-54.3633847588522,-54.1217120605348),.UNSPECIFIED.);
#2991=B_SPLINE_CURVE_WITH_KNOTS('',3,(#45004,#45005,#45006,#45007,#45008,
#45009,#45010,#45011,#45012,#45013,#45014,#45015,#45016,#45017,#45018,#45019,
#45020,#45021,#45022,#45023,#45024,#45025,#45026,#45027,#45028,#45029,#45030,
#45031,#45032,#45033,#45034,#45035,#45036,#45037,#45038,#45039,#45040,#45041,
#45042,#45043,#45044,#45045,#45046),.UNSPECIFIED.,.F.,.F.,(4,3,3,3,3,3,
3,3,3,3,3,3,3,3,4),(51.5750455984139,51.8696515130333,52.3683981621971,
52.8671448113608,53.3658914605246,53.8646381096884,54.3633847588522,54.862131408016,
55.3608780571797,55.8596247063435,56.3583713555073,56.8571180046711,57.3558646538349,
57.8546113029986,57.8582309055935),.UNSPECIFIED.);
#2992=B_SPLINE_CURVE_WITH_KNOTS('',3,(#45047,#45048,#45049,#45050,#45051,
#45052,#45053,#45054,#45055,#45056,#45057,#45058,#45059,#45060,#45061,#45062,
#45063,#45064,#45065,#45066,#45067,#45068,#45069,#45070,#45071,#45072,#45073,
#45074,#45075,#45076,#45077,#45078,#45079,#45080,#45081,#45082,#45083,#45084,
#45085,#45086,#45087,#45088,#45089),.UNSPECIFIED.,.F.,.F.,(4,3,3,3,3,3,
3,3,3,3,3,3,3,3,4),(-54.1217120605348,-53.8646381096884,-53.3658914605246,
-52.8671448113608,-52.3683981621971,-51.8696515130333,-51.3709048638695,
-50.8721582147057,-50.3734115655419,-49.8746649163781,-49.3759182672144,
-48.8771716180506,-48.3784249688868,-47.879678319723,-47.8385267533553),
 .UNSPECIFIED.);
#2993=B_SPLINE_CURVE_WITH_KNOTS('',3,(#45094,#45095,#45096,#45097,#45098,
#45099,#45100,#45101,#45102,#45103,#45104,#45105,#45106,#45107,#45108,#45109,
#45110,#45111,#45112,#45113,#45114,#45115,#45116,#45117,#45118,#45119,#45120,
#45121,#45122,#45123,#45124,#45125,#45126,#45127,#45128,#45129,#45130,#45131,
#45132,#45133,#45134,#45135,#45136),.UNSPECIFIED.,.F.,.F.,(4,3,3,3,3,3,
3,3,3,3,3,3,3,3,4),(45.2918602912343,45.3859450739041,45.8846917230679,
46.3834383722317,46.8821850213954,47.3809316705592,47.879678319723,48.3784249688868,
48.8771716180506,49.3759182672144,49.8746649163781,50.3734115655419,50.8721582147057,
51.3709048638695,51.5750455984139),.UNSPECIFIED.);
#2994=B_SPLINE_CURVE_WITH_KNOTS('',3,(#45137,#45138,#45139,#45140,#45141,
#45142,#45143,#45144,#45145,#45146,#45147,#45148,#45149,#45150,#45151,#45152,
#45153,#45154,#45155,#45156,#45157,#45158,#45159,#45160,#45161,#45162,#45163,
#45164,#45165,#45166,#45167,#45168,#45169,#45170,#45171,#45172,#45173,#45174,
#45175,#45176),.UNSPECIFIED.,.F.,.F.,(4,3,3,3,3,3,3,3,3,3,3,3,3,4),(-47.8385267533553,
-47.3809316705592,-46.8821850213955,-46.3834383722317,-45.8846917230679,
-45.3859450739041,-44.8871984247403,-44.3884517755765,-43.8897051264128,
-43.390958477249,-42.8922118280852,-42.3934651789214,-41.8947185297576,
-41.5553414461757),.UNSPECIFIED.);
#2995=B_SPLINE_CURVE_WITH_KNOTS('',3,(#45181,#45182,#45183,#45184,#45185,
#45186,#45187,#45188,#45189,#45190,#45191,#45192,#45193,#45194,#45195,#45196,
#45197,#45198,#45199,#45200,#45201,#45202,#45203,#45204,#45205,#45206,#45207,
#45208,#45209,#45210,#45211,#45212,#45213,#45214,#45215,#45216,#45217,#45218,
#45219,#45220),.UNSPECIFIED.,.F.,.F.,(4,3,3,3,3,3,3,3,3,3,3,3,3,4),(39.0086749840547,
39.4009852839387,39.8997319331025,40.3984785822663,40.8972252314301,41.3959718805938,
41.8947185297576,42.3934651789214,42.8922118280852,43.390958477249,43.8897051264128,
44.3884517755765,44.8871984247403,45.2918602912343),.UNSPECIFIED.);
#2996=B_SPLINE_CURVE_WITH_KNOTS('',3,(#45221,#45222,#45223,#45224,#45225,
#45226,#45227,#45228,#45229,#45230,#45231,#45232,#45233,#45234,#45235,#45236,
#45237,#45238,#45239,#45240,#45241,#45242,#45243,#45244,#45245,#45246,#45247,
#45248,#45249,#45250,#45251,#45252,#45253,#45254,#45255,#45256,#45257,#45258,
#45259,#45260,#45261,#45262,#45263),.UNSPECIFIED.,.F.,.F.,(4,3,3,3,3,3,
3,3,3,3,3,3,3,3,4),(-41.5553414461757,-41.3959718805939,-40.8972252314301,
-40.3984785822663,-39.8997319331025,-39.4009852839387,-38.902238634775,
-38.4034919856112,-37.9047453364474,-37.4059986872836,-36.9072520381198,
-36.4085053889561,-35.9097587397923,-35.4110120906285,-35.2721561389961),
 .UNSPECIFIED.);
#2997=B_SPLINE_CURVE_WITH_KNOTS('',3,(#45268,#45269,#45270,#45271,#45272,
#45273,#45274,#45275,#45276,#45277,#45278,#45279,#45280,#45281,#45282,#45283,
#45284,#45285,#45286,#45287,#45288,#45289,#45290,#45291,#45292,#45293,#45294,
#45295,#45296,#45297,#45298,#45299,#45300,#45301,#45302,#45303,#45304,#45305,
#45306,#45307,#45308,#45309,#45310),.UNSPECIFIED.,.F.,.F.,(4,3,3,3,3,3,
3,3,3,3,3,3,3,3,4),(32.7254896768751,32.9172788448096,33.4160254939734,
33.9147721431371,34.4135187923009,34.9122654414647,35.4110120906285,35.9097587397923,
36.408505388956,36.9072520381198,37.4059986872836,37.9047453364474,38.4034919856112,
38.9022386347749,39.0086749840547),.UNSPECIFIED.);
#2998=B_SPLINE_CURVE_WITH_KNOTS('',3,(#45311,#45312,#45313,#45314,#45315,
#45316,#45317,#45318,#45319,#45320,#45321,#45322,#45323,#45324,#45325,#45326,
#45327,#45328,#45329,#45330,#45331,#45332,#45333,#45334,#45335,#45336,#45337,
#45338,#45339,#45340,#45341,#45342,#45343,#45344,#45345,#45346,#45347,#45348,
#45349,#45350),.UNSPECIFIED.,.F.,.F.,(4,3,3,3,3,3,3,3,3,3,3,3,3,4),(-35.2721561389961,
-34.9122654414647,-34.4135187923009,-33.9147721431371,-33.4160254939734,
-32.9172788448096,-32.4185321956458,-31.919785546482,-31.4210388973182,
-30.9222922481544,-30.4235455989907,-29.9247989498269,-29.4260523006631,
-28.9889708318165),.UNSPECIFIED.);
#2999=B_SPLINE_CURVE_WITH_KNOTS('',3,(#45355,#45356,#45357,#45358,#45359,
#45360,#45361,#45362,#45363,#45364,#45365,#45366,#45367,#45368,#45369,#45370,
#45371,#45372,#45373,#45374,#45375,#45376,#45377,#45378,#45379,#45380,#45381,
#45382,#45383,#45384,#45385,#45386,#45387,#45388,#45389,#45390,#45391,#45392,
#45393,#45394),.UNSPECIFIED.,.F.,.F.,(4,3,3,3,3,3,3,3,3,3,3,3,3,4),(26.4423043696955,
26.9323190548442,27.431065704008,27.9298123531718,28.4285590023355,28.9273056514993,
29.4260523006631,29.9247989498269,30.4235455989907,30.9222922481544,31.4210388973182,
31.919785546482,32.4185321956458,32.7254896768751),.UNSPECIFIED.);
#3000=B_SPLINE_CURVE_WITH_KNOTS('',3,(#45395,#45396,#45397,#45398,#45399,
#45400,#45401,#45402,#45403,#45404,#45405,#45406,#45407,#45408,#45409,#45410,
#45411,#45412,#45413,#45414,#45415,#45416,#45417,#45418,#45419,#45420,#45421,
#45422,#45423,#45424,#45425,#45426,#45427,#45428,#45429,#45430,#45431,#45432,
#45433,#45434,#45435,#45436,#45437),.UNSPECIFIED.,.F.,.F.,(4,3,3,3,3,3,
3,3,3,3,3,3,3,3,4),(-28.9889708318165,-28.9273056514993,-28.4285590023355,
-27.9298123531718,-27.431065704008,-26.9323190548442,-26.4335724056804,
-25.9348257565166,-25.4360791073528,-24.9373324581891,-24.4385858090253,
-23.9398391598615,-23.4410925106977,-22.9423458615339,-22.7057855246369),
 .UNSPECIFIED.);
#3001=B_SPLINE_CURVE_WITH_KNOTS('',3,(#45442,#45443,#45444,#45445,#45446,
#45447,#45448,#45449,#45450,#45451,#45452,#45453,#45454,#45455,#45456,#45457,
#45458,#45459,#45460,#45461,#45462,#45463,#45464,#45465,#45466,#45467,#45468,
#45469,#45470,#45471,#45472,#45473,#45474,#45475,#45476,#45477,#45478,#45479,
#45480,#45481,#45482,#45483,#45484),.UNSPECIFIED.,.F.,.F.,(4,3,3,3,3,3,
3,3,3,3,3,3,3,3,4),(20.1591190625159,20.448612615715,20.9473592648788,21.4461059140426,
21.9448525632064,22.4435992123702,22.9423458615339,23.4410925106977,23.9398391598615,
24.4385858090253,24.9373324581891,25.4360791073529,25.9348257565166,26.4335724056804,
26.4423043696955),.UNSPECIFIED.);
#3002=B_SPLINE_CURVE_WITH_KNOTS('',3,(#45485,#45486,#45487,#45488,#45489,
#45490,#45491,#45492,#45493,#45494,#45495,#45496,#45497,#45498,#45499,#45500,
#45501,#45502,#45503,#45504,#45505,#45506,#45507,#45508,#45509,#45510,#45511,
#45512,#45513,#45514,#45515,#45516,#45517,#45518,#45519,#45520,#45521,#45522,
#45523,#45524,#45525,#45526,#45527),.UNSPECIFIED.,.F.,.F.,(4,3,3,3,3,3,
3,3,3,3,3,3,3,3,4),(-22.7057855246369,-22.4435992123702,-21.9448525632064,
-21.4461059140426,-20.9473592648788,-20.448612615715,-19.9498659665513,
-19.4511193173875,-18.9523726682237,-18.4536260190599,-17.9548793698961,
-17.4561327207323,-16.9573860715686,-16.4586394224048,-16.4226002174573),
 .UNSPECIFIED.);
#3003=B_SPLINE_CURVE_WITH_KNOTS('',3,(#45532,#45533,#45534,#45535,#45536,
#45537,#45538,#45539,#45540,#45541,#45542,#45543,#45544,#45545,#45546,#45547,
#45548,#45549,#45550,#45551,#45552,#45553,#45554,#45555,#45556,#45557,#45558,
#45559,#45560,#45561,#45562,#45563,#45564,#45565,#45566,#45567,#45568,#45569,
#45570,#45571,#45572,#45573,#45574),.UNSPECIFIED.,.F.,.F.,(4,3,3,3,3,3,
3,3,3,3,3,3,3,3,4),(13.8759337553364,13.9649061765859,14.4636528257497,
14.9623994749134,15.4611461240772,15.959892773241,16.4586394224048,16.9573860715686,
17.4561327207323,17.9548793698961,18.4536260190599,18.9523726682237,19.4511193173875,
19.9498659665513,20.1591190625159),.UNSPECIFIED.);
#3004=B_SPLINE_CURVE_WITH_KNOTS('',3,(#45575,#45576,#45577,#45578,#45579,
#45580,#45581,#45582,#45583,#45584,#45585,#45586,#45587,#45588,#45589,#45590,
#45591,#45592,#45593,#45594,#45595,#45596,#45597,#45598,#45599,#45600,#45601,
#45602,#45603,#45604,#45605,#45606,#45607,#45608,#45609,#45610,#45611,#45612,
#45613,#45614),.UNSPECIFIED.,.F.,.F.,(4,3,3,3,3,3,3,3,3,3,3,3,3,4),(-16.4226002174573,
-15.959892773241,-15.4611461240772,-14.9623994749134,-14.4636528257497,
-13.9649061765859,-13.4661595274221,-12.9674128782583,-12.4686662290945,
-11.9699195799308,-11.471172930767,-10.9724262816032,-10.4736796324394,
-10.1394149102777),.UNSPECIFIED.);
#3005=B_SPLINE_CURVE_WITH_KNOTS('',3,(#45620,#45621,#45622,#45623,#45624,
#45625,#45626,#45627,#45628,#45629,#45630,#45631,#45632,#45633,#45634,#45635,
#45636,#45637,#45638,#45639,#45640,#45641,#45642,#45643,#45644),
 .UNSPECIFIED.,.F.,.F.,(4,3,3,3,3,3,3,3,4),(-3.85622960309811,-3.49122654414647,
-2.99247989498269,-2.49373324581891,-1.99498659665513,-1.49623994749134,
-0.997493298327563,-0.498746649163781,0.),.UNSPECIFIED.);
#3006=B_SPLINE_CURVE_WITH_KNOTS('',3,(#45647,#45648,#45649,#45650,#45651,
#45652,#45653,#45654,#45655,#45656,#45657,#45658,#45659,#45660,#45661,#45662,
#45663,#45664,#45665,#45666,#45667,#45668,#45669,#45670,#45671,#45672,#45673,
#45674,#45675,#45676,#45677,#45678,#45679,#45680,#45681,#45682,#45683),
 .UNSPECIFIED.,.F.,.F.,(4,3,3,3,3,3,3,3,3,3,3,3,4),(2.02420009048538,2.49373324581891,
2.99247989498269,3.49122654414647,3.98997319331025,4.48871984247403,4.98746649163781,
5.4862131408016,5.98495978996538,6.48370643912916,6.98245308829294,7.48119973745672,
7.59274844815678),.UNSPECIFIED.);
#3007=B_SPLINE_CURVE_WITH_KNOTS('',3,(#45689,#45690,#45691,#45692,#45693,
#45694,#45695),.UNSPECIFIED.,.F.,.F.,(4,1,1,1,4),(191.637151868977,191.899274012976,
192.39802066214,192.896767311304,193.395513960467),.UNSPECIFIED.);
#3008=B_SPLINE_CURVE_WITH_KNOTS('',3,(#45698,#45699,#45700,#45701,#45702,
#45703,#45704,#45705),.UNSPECIFIED.,.F.,.F.,(4,1,1,1,1,4),(191.637151868977,
191.952207229278,192.450953878442,192.949700527606,193.448447176769,193.917980332103),
 .UNSPECIFIED.);
#3009=B_SPLINE_CURVE_WITH_KNOTS('',3,(#45710,#45711,#45712,#45713,#45714,
#45715,#45716,#45717,#45718,#45719,#45720,#45721,#45722,#45723,#45724,#45725,
#45726),.UNSPECIFIED.,.F.,.F.,(4,1,1,1,1,1,1,1,1,1,1,1,1,1,4),(185.353966561798,
185.415567573847,185.914314223011,186.413060872174,186.911807521338,187.410554170502,
187.909300819666,188.40804746883,188.906794117993,189.405540767157,189.904287416321,
190.403034065485,190.901780714648,191.400527363812,191.637151868977),
 .UNSPECIFIED.);
#3010=B_SPLINE_CURVE_WITH_KNOTS('',3,(#45727,#45728,#45729,#45730,#45731,
#45732,#45733,#45734,#45735,#45736,#45737,#45738,#45739,#45740,#45741,#45742,
#45743),.UNSPECIFIED.,.F.,.F.,(4,1,1,1,1,1,1,1,1,1,1,1,1,1,4),(185.353966561798,
185.468500790149,185.967247439313,186.465994088476,186.96474073764,187.463487386804,
187.962234035968,188.460980685132,188.959727334295,189.458473983459,189.957220632623,
190.455967281787,190.954713930951,191.453460580114,191.637151868977),
 .UNSPECIFIED.);
#3011=B_SPLINE_CURVE_WITH_KNOTS('',3,(#45748,#45749,#45750,#45751,#45752,
#45753,#45754,#45755,#45756,#45757,#45758,#45759,#45760,#45761,#45762,#45763),
 .UNSPECIFIED.,.F.,.F.,(4,1,1,1,1,1,1,1,1,1,1,1,1,4),(179.070781254618,
179.430607783881,179.929354433045,180.428101082209,180.926847731373,181.425594380537,
181.9243410297,182.423087678864,182.921834328028,183.420580977192,183.919327626356,
184.418074275519,184.916820924683,185.353966561798),.UNSPECIFIED.);
#3012=B_SPLINE_CURVE_WITH_KNOTS('',3,(#45764,#45765,#45766,#45767,#45768,
#45769,#45770,#45771,#45772,#45773,#45774,#45775,#45776,#45777,#45778,#45779),
 .UNSPECIFIED.,.F.,.F.,(4,1,1,1,1,1,1,1,1,1,1,1,1,4),(179.070781254618,
179.483541000184,179.982287649347,180.481034298511,180.979780947675,181.478527596839,
181.977274246002,182.476020895166,182.97476754433,183.473514193494,183.972260842658,
184.471007491821,184.969754140985,185.353966561798),.UNSPECIFIED.);
#3013=B_SPLINE_CURVE_WITH_KNOTS('',3,(#45784,#45785,#45786,#45787,#45788,
#45789,#45790,#45791,#45792,#45793,#45794,#45795,#45796,#45797,#45798,#45799,
#45800),.UNSPECIFIED.,.F.,.F.,(4,1,1,1,1,1,1,1,1,1,1,1,1,1,4),(172.787595947439,
172.946901344752,173.445647993916,173.94439464308,174.443141292244,174.941887941407,
175.440634590571,175.939381239735,176.438127888899,176.936874538063,177.435621187226,
177.93436783639,178.433114485554,178.931861134718,179.070781254618),
 .UNSPECIFIED.);
#3014=B_SPLINE_CURVE_WITH_KNOTS('',3,(#45801,#45802,#45803,#45804,#45805,
#45806,#45807,#45808,#45809,#45810,#45811,#45812,#45813,#45814,#45815,#45816,
#45817),.UNSPECIFIED.,.F.,.F.,(4,1,1,1,1,1,1,1,1,1,1,1,1,1,4),(172.787595947439,
172.999834561054,173.498581210218,173.997327859382,174.496074508546,174.99482115771,
175.493567806873,175.992314456037,176.491061105201,176.989807754365,177.488554403528,
177.987301052692,178.486047701856,178.98479435102,179.070781254618),
 .UNSPECIFIED.);
#3015=B_SPLINE_CURVE_WITH_KNOTS('',3,(#45822,#45823,#45824,#45825,#45826,
#45827,#45828,#45829,#45830,#45831,#45832,#45833,#45834,#45835,#45836,#45837),
 .UNSPECIFIED.,.F.,.F.,(4,1,1,1,1,1,1,1,1,1,1,1,1,4),(166.504410640259,
166.961941554787,167.460688203951,167.959434853114,168.458181502278,168.956928151442,
169.455674800606,169.95442144977,170.453168098933,170.951914748097,171.450661397261,
171.949408046425,172.448154695589,172.787595947439),.UNSPECIFIED.);
#3016=B_SPLINE_CURVE_WITH_KNOTS('',3,(#45838,#45839,#45840,#45841,#45842,
#45843,#45844,#45845,#45846,#45847,#45848,#45849,#45850,#45851,#45852,#45853,
#45854),.UNSPECIFIED.,.F.,.F.,(4,1,1,1,1,1,1,1,1,1,1,1,1,1,4),(166.504410640259,
166.516128121925,167.014874771089,167.513621420253,168.012368069417,168.51111471858,
169.009861367744,169.508608016908,170.007354666072,170.506101315235,171.004847964399,
171.503594613563,172.002341262727,172.501087911891,172.787595947439),
 .UNSPECIFIED.);
#3017=B_SPLINE_CURVE_WITH_KNOTS('',3,(#45859,#45860,#45861,#45862,#45863,
#45864,#45865,#45866,#45867,#45868,#45869,#45870,#45871,#45872,#45873,#45874,
#45875),.UNSPECIFIED.,.F.,.F.,(4,1,1,1,1,1,1,1,1,1,1,1,1,1,4),(160.22122533308,
160.478235115658,160.976981764822,161.475728413985,161.974475063149,162.473221712313,
162.971968361477,163.47071501064,163.969461659804,164.468208308968,164.966954958132,
165.465701607296,165.964448256459,166.463194905623,166.504410640259),
 .UNSPECIFIED.);
#3018=B_SPLINE_CURVE_WITH_KNOTS('',3,(#45876,#45877,#45878,#45879,#45880,
#45881,#45882,#45883,#45884,#45885,#45886,#45887,#45888,#45889,#45890,#45891),
 .UNSPECIFIED.,.F.,.F.,(4,1,1,1,1,1,1,1,1,1,1,1,1,4),(160.22122533308,160.53116833196,
161.029914981124,161.528661630287,162.027408279451,162.526154928615,163.024901577779,
163.523648226943,164.022394876106,164.52114152527,165.019888174434,165.518634823598,
166.017381472761,166.504410640259),.UNSPECIFIED.);
#3019=B_SPLINE_CURVE_WITH_KNOTS('',3,(#45896,#45897,#45898,#45899,#45900,
#45901,#45902,#45903,#45904,#45905,#45906,#45907,#45908,#45909,#45910,#45911,
#45912),.UNSPECIFIED.,.F.,.F.,(4,1,1,1,1,1,1,1,1,1,1,1,1,1,4),(153.9380400259,
153.994528676529,154.493275325692,154.992021974856,155.49076862402,155.989515273184,
156.488261922348,156.987008571511,157.485755220675,157.984501869839,158.483248519003,
158.981995168166,159.48074181733,159.979488466494,160.22122533308),
 .UNSPECIFIED.);
#3020=B_SPLINE_CURVE_WITH_KNOTS('',3,(#45913,#45914,#45915,#45916,#45917,
#45918,#45919,#45920,#45921,#45922,#45923,#45924,#45925,#45926,#45927,#45928,
#45929),.UNSPECIFIED.,.F.,.F.,(4,1,1,1,1,1,1,1,1,1,1,1,1,1,4),(153.9380400259,
154.047461892831,154.546208541994,155.044955191158,155.543701840322,156.042448489486,
156.54119513865,157.039941787813,157.538688436977,158.037435086141,158.536181735305,
159.034928384469,159.533675033632,160.032421682796,160.22122533308),
 .UNSPECIFIED.);
#3021=B_SPLINE_CURVE_WITH_KNOTS('',3,(#45934,#45935,#45936,#45937,#45938,
#45939,#45940,#45941,#45942,#45943,#45944,#45945,#45946,#45947,#45948,#45949),
 .UNSPECIFIED.,.F.,.F.,(4,1,1,1,1,1,1,1,1,1,1,1,1,4),(147.65485471872,148.009568886563,
148.508315535727,149.007062184891,149.505808834055,150.004555483218,150.503302132382,
151.002048781546,151.50079543071,151.999542079873,152.498288729037,152.997035378201,
153.495782027365,153.9380400259),.UNSPECIFIED.);
#3022=B_SPLINE_CURVE_WITH_KNOTS('',3,(#45950,#45951,#45952,#45953,#45954,
#45955,#45956,#45957,#45958,#45959,#45960,#45961,#45962,#45963,#45964,#45965),
 .UNSPECIFIED.,.F.,.F.,(4,1,1,1,1,1,1,1,1,1,1,1,1,4),(147.65485471872,148.062502102865,
148.561248752029,149.059995401193,149.558742050357,150.05748869952,150.556235348684,
151.054981997848,151.553728647012,152.052475296176,152.551221945339,153.049968594503,
153.548715243667,153.9380400259),.UNSPECIFIED.);
#3023=B_SPLINE_CURVE_WITH_KNOTS('',3,(#45970,#45971,#45972,#45973,#45974,
#45975,#45976,#45977,#45978,#45979,#45980,#45981,#45982,#45983,#45984,#45985,
#45986),.UNSPECIFIED.,.F.,.F.,(4,1,1,1,1,1,1,1,1,1,1,1,1,1,4),(141.371669411541,
141.525862447434,142.024609096598,142.523355745762,143.022102394925,143.520849044089,
144.019595693253,144.518342342417,145.017088991581,145.515835640744,146.014582289908,
146.513328939072,147.012075588236,147.510822237399,147.65485471872),
 .UNSPECIFIED.);
#3024=B_SPLINE_CURVE_WITH_KNOTS('',3,(#45987,#45988,#45989,#45990,#45991,
#45992,#45993,#45994,#45995,#45996,#45997,#45998,#45999,#46000,#46001,#46002,
#46003),.UNSPECIFIED.,.F.,.F.,(4,1,1,1,1,1,1,1,1,1,1,1,1,1,4),(141.371669411541,
141.578795663736,142.0775423129,142.576288962064,143.075035611227,143.573782260391,
144.072528909555,144.571275558719,145.070022207883,145.568768857046,146.06751550621,
146.566262155374,147.065008804538,147.563755453702,147.65485471872),
 .UNSPECIFIED.);
#3025=B_SPLINE_CURVE_WITH_KNOTS('',3,(#46008,#46009,#46010,#46011,#46012,
#46013,#46014,#46015,#46016,#46017,#46018,#46019,#46020,#46021,#46022,#46023),
 .UNSPECIFIED.,.F.,.F.,(4,1,1,1,1,1,1,1,1,1,1,1,1,4),(135.088484104361,
135.540902657469,136.039649306632,136.538395955796,137.03714260496,137.535889254124,
138.034635903288,138.533382552451,139.032129201615,139.530875850779,140.029622499943,
140.528369149107,141.02711579827,141.371669411541),.UNSPECIFIED.);
#3026=B_SPLINE_CURVE_WITH_KNOTS('',3,(#46024,#46025,#46026,#46027,#46028,
#46029,#46030,#46031,#46032,#46033,#46034,#46035,#46036,#46037,#46038,#46039,
#46040),.UNSPECIFIED.,.F.,.F.,(4,1,1,1,1,1,1,1,1,1,1,1,1,1,4),(135.088484104361,
135.095089224607,135.593835873771,136.092582522935,136.591329172098,137.090075821262,
137.588822470426,138.08756911959,138.586315768753,139.085062417917,139.583809067081,
140.082555716245,140.581302365409,141.080049014572,141.371669411541),
 .UNSPECIFIED.);
#3027=B_SPLINE_CURVE_WITH_KNOTS('',3,(#46045,#46046,#46047,#46048,#46049,
#46050,#46051,#46052,#46053,#46054,#46055,#46056,#46057,#46058,#46059,#46060,
#46061),.UNSPECIFIED.,.F.,.F.,(4,1,1,1,1,1,1,1,1,1,1,1,1,1,4),(128.805298797182,
129.05719621834,129.555942867503,130.054689516667,130.553436165831,131.052182814995,
131.550929464158,132.049676113322,132.548422762486,133.04716941165,133.545916060814,
134.044662709977,134.543409359141,135.042156008305,135.088484104361),
 .UNSPECIFIED.);
#3028=B_SPLINE_CURVE_WITH_KNOTS('',3,(#46062,#46063,#46064,#46065,#46066,
#46067,#46068,#46069,#46070,#46071,#46072,#46073,#46074,#46075,#46076,#46077),
 .UNSPECIFIED.,.F.,.F.,(4,1,1,1,1,1,1,1,1,1,1,1,1,4),(128.805298797182,
129.110129434642,129.608876083805,130.107622732969,130.606369382133,131.105116031297,
131.603862680461,132.102609329624,132.601355978788,133.100102627952,133.598849277116,
134.097595926279,134.596342575443,135.088484104361),.UNSPECIFIED.);
#3029=B_SPLINE_CURVE_WITH_KNOTS('',3,(#46082,#46083,#46084,#46085,#46086,
#46087,#46088,#46089,#46090,#46091,#46092,#46093,#46094,#46095,#46096,#46097,
#46098),.UNSPECIFIED.,.F.,.F.,(4,1,1,1,1,1,1,1,1,1,1,1,1,1,4),(122.522113490002,
122.57348977921,123.072236428374,123.570983077538,124.069729726702,124.568476375866,
125.067223025029,125.565969674193,126.064716323357,126.563462972521,127.062209621684,
127.560956270848,128.059702920012,128.558449569176,128.805298797182),
 .UNSPECIFIED.);
#3030=B_SPLINE_CURVE_WITH_KNOTS('',3,(#46099,#46100,#46101,#46102,#46103,
#46104,#46105,#46106,#46107,#46108,#46109,#46110,#46111,#46112,#46113,#46114,
#46115),.UNSPECIFIED.,.F.,.F.,(4,1,1,1,1,1,1,1,1,1,1,1,1,1,4),(122.522113490002,
122.626422995512,123.125169644676,123.62391629384,124.122662943004,124.621409592168,
125.120156241331,125.618902890495,126.117649539659,126.616396188823,127.115142837986,
127.61388948715,128.112636136314,128.611382785478,128.805298797182),
 .UNSPECIFIED.);
#3031=B_SPLINE_CURVE_WITH_KNOTS('',3,(#46120,#46121,#46122,#46123,#46124,
#46125,#46126,#46127,#46128,#46129,#46130,#46131,#46132,#46133,#46134,#46135),
 .UNSPECIFIED.,.F.,.F.,(4,1,1,1,1,1,1,1,1,1,1,1,1,4),(116.238928182823,
116.588529989245,117.087276638409,117.586023287573,118.084769936736,118.5835165859,
119.082263235064,119.581009884228,120.079756533392,120.578503182555,121.077249831719,
121.575996480883,122.074743130047,122.522113490002),.UNSPECIFIED.);
#3032=B_SPLINE_CURVE_WITH_KNOTS('',3,(#46136,#46137,#46138,#46139,#46140,
#46141,#46142,#46143,#46144,#46145,#46146,#46147,#46148,#46149,#46150,#46151),
 .UNSPECIFIED.,.F.,.F.,(4,1,1,1,1,1,1,1,1,1,1,1,1,4),(116.238928182823,
116.641463205547,117.140209854711,117.638956503875,118.137703153038,118.636449802202,
119.135196451366,119.63394310053,120.132689749694,120.631436398857,121.130183048021,
121.628929697185,122.127676346349,122.522113490002),.UNSPECIFIED.);
#3033=B_SPLINE_CURVE_WITH_KNOTS('',3,(#46156,#46157,#46158,#46159,#46160,
#46161,#46162,#46163,#46164,#46165,#46166,#46167,#46168,#46169,#46170,#46171,
#46172),.UNSPECIFIED.,.F.,.F.,(4,1,1,1,1,1,1,1,1,1,1,1,1,1,4),(109.955742875643,
110.104823550116,110.60357019928,111.102316848443,111.601063497607,112.099810146771,
112.598556795935,113.097303445099,113.596050094262,114.094796743426,114.59354339259,
115.092290041754,115.591036690917,116.089783340081,116.238928182823),
 .UNSPECIFIED.);
#3034=B_SPLINE_CURVE_WITH_KNOTS('',3,(#46173,#46174,#46175,#46176,#46177,
#46178,#46179,#46180,#46181,#46182,#46183,#46184,#46185,#46186,#46187,#46188,
#46189),.UNSPECIFIED.,.F.,.F.,(4,1,1,1,1,1,1,1,1,1,1,1,1,1,4),(109.955742875643,
110.157756766418,110.656503415582,111.155250064746,111.653996713909,112.152743363073,
112.651490012237,113.150236661401,113.648983310564,114.147729959728,114.646476608892,
115.145223258056,115.64396990722,116.142716556383,116.238928182823),
 .UNSPECIFIED.);
#3035=B_SPLINE_CURVE_WITH_KNOTS('',3,(#46194,#46195,#46196,#46197,#46198,
#46199,#46200,#46201,#46202,#46203,#46204,#46205,#46206,#46207,#46208,#46209),
 .UNSPECIFIED.,.F.,.F.,(4,1,1,1,1,1,1,1,1,1,1,1,1,4),(103.672557568463,
104.11986376015,104.618610409314,105.117357058478,105.616103707642,106.114850356806,
106.613597005969,107.112343655133,107.611090304297,108.109836953461,108.608583602625,
109.107330251788,109.606076900952,109.955742875643),.UNSPECIFIED.);
#3036=B_SPLINE_CURVE_WITH_KNOTS('',3,(#46210,#46211,#46212,#46213,#46214,
#46215,#46216,#46217,#46218,#46219,#46220,#46221,#46222,#46223,#46224,#46225,
#46226),.UNSPECIFIED.,.F.,.F.,(4,1,1,1,1,1,1,1,1,1,1,1,1,1,4),(103.672557568463,
103.674050327289,104.172796976453,104.671543625616,105.17029027478,105.669036923944,
106.167783573108,106.666530222271,107.165276871435,107.664023520599,108.162770169763,
108.661516818927,109.16026346809,109.659010117254,109.955742875643),
 .UNSPECIFIED.);
#3037=B_SPLINE_CURVE_WITH_KNOTS('',3,(#46231,#46232,#46233,#46234,#46235,
#46236,#46237,#46238,#46239,#46240,#46241,#46242,#46243,#46244,#46245,#46246,
#46247),.UNSPECIFIED.,.F.,.F.,(4,1,1,1,1,1,1,1,1,1,1,1,1,1,4),(97.3893722612838,
97.6361573210213,98.1349039701851,98.6336506193489,99.1323972685127,99.6311439176765,
100.12989056684,100.628637216004,101.127383865168,101.626130514332,102.124877163495,
102.623623812659,103.122370461823,103.621117110987,103.672557568463),
 .UNSPECIFIED.);
#3038=B_SPLINE_CURVE_WITH_KNOTS('',3,(#46248,#46249,#46250,#46251,#46252,
#46253,#46254,#46255,#46256,#46257,#46258,#46259,#46260,#46261,#46262,#46263),
 .UNSPECIFIED.,.F.,.F.,(4,1,1,1,1,1,1,1,1,1,1,1,1,4),(97.3893722612837,
97.6890905373234,98.1878371864872,98.686583835651,99.1853304848147,99.6840771339785,
100.182823783142,100.681570432306,101.18031708147,101.679063730634,102.177810379797,
102.676557028961,103.175303678125,103.672557568463),.UNSPECIFIED.);
#3039=B_SPLINE_CURVE_WITH_KNOTS('',3,(#46268,#46269,#46270,#46271,#46272,
#46273,#46274,#46275,#46276,#46277,#46278,#46279,#46280,#46281,#46282,#46283,
#46284),.UNSPECIFIED.,.F.,.F.,(4,1,1,1,1,1,1,1,1,1,1,1,1,1,4),(91.1061869541041,
91.1524508818922,91.651197531056,92.1499441802197,92.6486908293835,93.1474374785473,
93.6461841277111,94.1449307768749,94.6436774260386,95.1424240752024,95.6411707243662,
96.13991737353,96.6386640226938,97.1374106718576,97.3893722612838),
 .UNSPECIFIED.);
#3040=B_SPLINE_CURVE_WITH_KNOTS('',3,(#46285,#46286,#46287,#46288,#46289,
#46290,#46291,#46292,#46293,#46294,#46295,#46296,#46297,#46298,#46299,#46300,
#46301),.UNSPECIFIED.,.F.,.F.,(4,1,1,1,1,1,1,1,1,1,1,1,1,1,4),(91.1061869541041,
91.2053840981942,91.704130747358,92.2028773965218,92.7016240456856,93.2003706948494,
93.6991173440131,94.1978639931769,94.6966106423407,95.1953572915045,95.6941039406683,
96.1928505898321,96.6915972389958,97.1903438881596,97.3893722612837),
 .UNSPECIFIED.);
#3041=B_SPLINE_CURVE_WITH_KNOTS('',3,(#46306,#46307,#46308,#46309,#46310,
#46311,#46312,#46313,#46314,#46315,#46316,#46317,#46318,#46319,#46320,#46321),
 .UNSPECIFIED.,.F.,.F.,(4,1,1,1,1,1,1,1,1,1,1,1,1,4),(84.8230016469246,
85.1674910919268,85.6662377410906,86.1649843902544,86.6637310394181,87.1624776885819,
87.6612243377457,88.1599709869095,88.6587176360733,89.1574642852371,89.6562109344008,
90.1549575835646,90.6537042327284,91.1061869541041),.UNSPECIFIED.);
#3042=B_SPLINE_CURVE_WITH_KNOTS('',3,(#46322,#46323,#46324,#46325,#46326,
#46327,#46328,#46329,#46330,#46331,#46332,#46333,#46334,#46335,#46336,#46337),
 .UNSPECIFIED.,.F.,.F.,(4,1,1,1,1,1,1,1,1,1,1,1,1,4),(84.8230016469245,
85.2204243082289,85.7191709573926,86.2179176065564,86.7166642557202,87.215410904884,
87.7141575540478,88.2129042032116,88.7116508523753,89.2103975015391,89.7091441507029,
90.2078907998667,90.7066374490305,91.1061869541041),.UNSPECIFIED.);
#3043=B_SPLINE_CURVE_WITH_KNOTS('',3,(#46342,#46343,#46344,#46345,#46346,
#46347,#46348,#46349,#46350,#46351,#46352,#46353,#46354,#46355,#46356,#46357,
#46358),.UNSPECIFIED.,.F.,.F.,(4,1,1,1,1,1,1,1,1,1,1,1,1,1,4),(78.539816339745,
78.6837846527976,79.1825313019614,79.6812779511252,80.180024600289,80.6787712494528,
81.1775178986165,81.6762645477803,82.1750111969441,82.6737578461079,83.1725044952717,
83.6712511444355,84.1699977935992,84.668744442763,84.8230016469246),
 .UNSPECIFIED.);
#3044=B_SPLINE_CURVE_WITH_KNOTS('',3,(#46359,#46360,#46361,#46362,#46363,
#46364,#46365,#46366,#46367,#46368,#46369,#46370,#46371,#46372,#46373,#46374,
#46375),.UNSPECIFIED.,.F.,.F.,(4,1,1,1,1,1,1,1,1,1,1,1,1,1,4),(78.539816339745,
78.7367178690997,79.2354645182635,79.7342111674273,80.2329578165911,80.7317044657548,
81.2304511149186,81.7291977640824,82.2279444132462,82.72669106241,83.2254377115737,
83.7241843607375,84.2229310099013,84.7216776590651,84.8230016469245),
 .UNSPECIFIED.);
#3045=B_SPLINE_CURVE_WITH_KNOTS('',3,(#46380,#46381,#46382,#46383,#46384,
#46385,#46386,#46387,#46388,#46389,#46390,#46391,#46392,#46393,#46394,#46395),
 .UNSPECIFIED.,.F.,.F.,(4,1,1,1,1,1,1,1,1,1,1,1,1,4),(72.2566310325654,
72.6988248628323,73.197571511996,73.6963181611598,74.1950648103236,74.6938114594874,
75.1925581086512,75.6913047578149,76.1900514069787,76.6887980561425,77.1875447053063,
77.6862913544701,78.1850380036339,78.539816339745),.UNSPECIFIED.);
#3046=B_SPLINE_CURVE_WITH_KNOTS('',3,(#46396,#46397,#46398,#46399,#46400,
#46401,#46402,#46403,#46404,#46405,#46406,#46407,#46408,#46409,#46410,#46411),
 .UNSPECIFIED.,.F.,.F.,(4,1,1,1,1,1,1,1,1,1,1,1,1,4),(72.2566310325654,
72.7517580791343,73.2505047282981,73.7492513774619,74.2479980266257,74.7467446757895,
75.2454913249532,75.744237974117,76.2429846232808,76.7417312724446,77.2404779216084,
77.7392245707722,78.2379712199359,78.539816339745),.UNSPECIFIED.);
#3047=B_SPLINE_CURVE_WITH_KNOTS('',3,(#46416,#46417,#46418,#46419,#46420,
#46421,#46422,#46423,#46424,#46425,#46426,#46427,#46428,#46429,#46430,#46431,
#46432),.UNSPECIFIED.,.F.,.F.,(4,1,1,1,1,1,1,1,1,1,1,1,1,1,4),(65.9734457253858,
66.2151184237031,66.7138650728669,67.2126117220307,67.7113583711945,68.2101050203582,
68.708851669522,69.2075983186858,69.7063449678496,70.2050916170134,70.7038382661771,
71.2025849153409,71.7013315645047,72.2000782136685,72.2566310325654),
 .UNSPECIFIED.);
#3048=B_SPLINE_CURVE_WITH_KNOTS('',3,(#46433,#46434,#46435,#46436,#46437,
#46438,#46439,#46440,#46441,#46442,#46443,#46444,#46445,#46446,#46447,#46448,
#46449),.UNSPECIFIED.,.F.,.F.,(4,1,1,1,1,1,1,1,1,1,1,1,1,1,4),(65.9734457253858,
66.2680516400052,66.766798289169,67.2655449383327,67.7642915874965,68.2630382366603,
68.7617848858241,69.2605315349879,69.7592781841516,70.2580248333154,70.7567714824792,
71.255518131643,71.7542647808068,72.2530114299706,72.2566310325654),
 .UNSPECIFIED.);
#3049=B_SPLINE_CURVE_WITH_KNOTS('',3,(#46454,#46455,#46456,#46457,#46458,
#46459,#46460,#46461,#46462,#46463,#46464,#46465,#46466,#46467,#46468,#46469,
#46470),.UNSPECIFIED.,.F.,.F.,(4,1,1,1,1,1,1,1,1,1,1,1,1,1,4),(59.6902604182062,
59.731411984574,60.2301586337377,60.7289052829015,61.2276519320653,61.7263985812291,
62.2251452303929,62.7238918795566,63.2226385287204,63.7213851778842,64.220131827048,
64.7188784762118,65.2176251253755,65.7163717745393,65.9734457253858),
 .UNSPECIFIED.);
#3050=B_SPLINE_CURVE_WITH_KNOTS('',3,(#46471,#46472,#46473,#46474,#46475,
#46476,#46477,#46478,#46479,#46480,#46481,#46482,#46483,#46484,#46485,#46486,
#46487),.UNSPECIFIED.,.F.,.F.,(4,1,1,1,1,1,1,1,1,1,1,1,1,1,4),(59.6902604182062,
59.784345200876,60.2830918500398,60.7818384992036,61.2805851483674,61.7793317975311,
62.2780784466949,62.7768250958587,63.2755717450225,63.7743183941863,64.2730650433501,
64.7718116925138,65.2705583416776,65.7693049908414,65.9734457253858),
 .UNSPECIFIED.);
#3051=B_SPLINE_CURVE_WITH_KNOTS('',3,(#46492,#46493,#46494,#46495,#46496,
#46497,#46498,#46499,#46500,#46501,#46502,#46503,#46504,#46505,#46506,#46507),
 .UNSPECIFIED.,.F.,.F.,(4,1,1,1,1,1,1,1,1,1,1,1,1,4),(53.4070751110266,
53.7464521946086,54.2451988437724,54.7439454929361,55.2426921420999,55.7414387912637,
56.2401854404275,56.7389320895913,57.237678738755,57.7364253879188,58.2351720370826,
58.7339186862464,59.2326653354102,59.6902604182062),.UNSPECIFIED.);
#3052=B_SPLINE_CURVE_WITH_KNOTS('',3,(#46508,#46509,#46510,#46511,#46512,
#46513,#46514,#46515,#46516,#46517,#46518,#46519,#46520,#46521,#46522,#46523),
 .UNSPECIFIED.,.F.,.F.,(4,1,1,1,1,1,1,1,1,1,1,1,1,4),(53.4070751110266,
53.7993854109106,54.2981320600744,54.7968787092382,55.295625358402,55.7943720075658,
56.2931186567296,56.7918653058933,57.2906119550571,57.7893586042209,58.2881052533847,
58.7868519025485,59.2855985517122,59.6902604182062),.UNSPECIFIED.);
#3053=B_SPLINE_CURVE_WITH_KNOTS('',3,(#46528,#46529,#46530,#46531,#46532,
#46533,#46534,#46535,#46536,#46537,#46538,#46539,#46540,#46541,#46542,#46543,
#46544),.UNSPECIFIED.,.F.,.F.,(4,1,1,1,1,1,1,1,1,1,1,1,1,1,4),(47.123889803847,
47.2627457554794,47.7614924046432,48.260239053807,48.7589857029708,49.2577323521345,
49.7564790012983,50.2552256504621,50.7539722996259,51.2527189487897,51.7514655979534,
52.2502122471172,52.748958896281,53.2477055454448,53.4070751110266),
 .UNSPECIFIED.);
#3054=B_SPLINE_CURVE_WITH_KNOTS('',3,(#46545,#46546,#46547,#46548,#46549,
#46550,#46551,#46552,#46553,#46554,#46555,#46556,#46557,#46558,#46559,#46560,
#46561),.UNSPECIFIED.,.F.,.F.,(4,1,1,1,1,1,1,1,1,1,1,1,1,1,4),(47.123889803847,
47.3156789717815,47.8144256209453,48.313172270109,48.8119189192728,49.3106655684366,
49.8094122176004,50.3081588667642,50.806905515928,51.3056521650917,51.8043988142555,
52.3031454634193,52.8018921125831,53.3006387617469,53.4070751110266),
 .UNSPECIFIED.);
#3055=B_SPLINE_CURVE_WITH_KNOTS('',3,(#46566,#46567,#46568,#46569,#46570,
#46571,#46572,#46573,#46574,#46575,#46576,#46577,#46578,#46579,#46580,#46581),
 .UNSPECIFIED.,.F.,.F.,(4,1,1,1,1,1,1,1,1,1,1,1,1,4),(40.8407044966674,
41.277785965514,41.7765326146778,42.2752792638416,42.7740259130054,43.2727725621692,
43.7715192113329,44.2702658604967,44.7690125096605,45.2677591588243,45.7665058079881,
46.2652524571519,46.7639991063156,47.123889803847),.UNSPECIFIED.);
#3056=B_SPLINE_CURVE_WITH_KNOTS('',3,(#46582,#46583,#46584,#46585,#46586,
#46587,#46588,#46589,#46590,#46591,#46592,#46593,#46594,#46595,#46596,#46597),
 .UNSPECIFIED.,.F.,.F.,(4,1,1,1,1,1,1,1,1,1,1,1,1,4),(40.8407044966674,
41.3307191818161,41.8294658309799,42.3282124801437,42.8269591293075,43.3257057784712,
43.824452427635,44.3231990767988,44.8219457259626,45.3206923751264,45.8194390242901,
46.3181856734539,46.8169323226177,47.123889803847),.UNSPECIFIED.);
#3057=B_SPLINE_CURVE_WITH_KNOTS('',3,(#46602,#46603,#46604,#46605,#46606,
#46607,#46608,#46609,#46610,#46611,#46612,#46613,#46614,#46615,#46616,#46617,
#46618),.UNSPECIFIED.,.F.,.F.,(4,1,1,1,1,1,1,1,1,1,1,1,1,1,4),(34.5575191894878,
34.7940795263849,35.2928261755487,35.7915728247124,36.2903194738762,36.78906612304,
37.2878127722038,37.7865594213676,38.2853060705313,38.7840527196951,39.2827993688589,
39.7815460180227,40.2802926671865,40.7790393163503,40.8407044966674),
 .UNSPECIFIED.);
#3058=B_SPLINE_CURVE_WITH_KNOTS('',3,(#46619,#46620,#46621,#46622,#46623,
#46624,#46625,#46626,#46627,#46628,#46629,#46630,#46631,#46632,#46633,#46634,
#46635),.UNSPECIFIED.,.F.,.F.,(4,1,1,1,1,1,1,1,1,1,1,1,1,1,4),(34.5575191894878,
34.847012742687,35.3457593918507,35.8445060410145,36.3432526901783,36.8419993393421,
37.3407459885059,37.8394926376697,38.3382392868334,38.8369859359972,39.335732585161,
39.8344792343248,40.3332258834886,40.8319725326523,40.8407044966674),
 .UNSPECIFIED.);
#3059=B_SPLINE_CURVE_WITH_KNOTS('',3,(#46640,#46641,#46642,#46643,#46644,
#46645,#46646,#46647,#46648,#46649,#46650,#46651,#46652,#46653,#46654,#46655,
#46656),.UNSPECIFIED.,.F.,.F.,(4,1,1,1,1,1,1,1,1,1,1,1,1,1,4),(28.2743338823083,
28.3103730872557,28.8091197364195,29.3078663855833,29.8066130347471,30.3053596839108,
30.8041063330746,31.3028529822384,31.8015996314022,32.300346280566,32.7990929297298,
33.2978395788935,33.7965862280573,34.2953328772211,34.5575191894878),
 .UNSPECIFIED.);
#3060=B_SPLINE_CURVE_WITH_KNOTS('',3,(#46657,#46658,#46659,#46660,#46661,
#46662,#46663,#46664,#46665,#46666,#46667,#46668,#46669,#46670,#46671,#46672,
#46673),.UNSPECIFIED.,.F.,.F.,(4,1,1,1,1,1,1,1,1,1,1,1,1,1,4),(28.2743338823082,
28.3633063035578,28.8620529527216,29.3607996018854,29.8595462510491,30.3582929002129,
30.8570395493767,31.3557861985405,31.8545328477043,32.353279496868,32.8520261460318,
33.3507727951956,33.8495194443594,34.3482660935232,34.5575191894878),
 .UNSPECIFIED.);
#3061=B_SPLINE_CURVE_WITH_KNOTS('',3,(#46678,#46679,#46680,#46681,#46682,
#46683,#46684,#46685,#46686,#46687,#46688,#46689,#46690,#46691,#46692,#46693),
 .UNSPECIFIED.,.F.,.F.,(4,1,1,1,1,1,1,1,1,1,1,1,1,4),(21.9911485751287,
22.3254132972903,22.8241599464541,23.3229065956179,23.8216532447817,24.3203998939455,
24.8191465431093,25.317893192273,25.8166398414368,26.3153864906006,26.8141331397644,
27.3128797889282,27.8116264380919,28.2743338823083),.UNSPECIFIED.);
#3062=B_SPLINE_CURVE_WITH_KNOTS('',3,(#46694,#46695,#46696,#46697,#46698,
#46699,#46700,#46701,#46702,#46703,#46704,#46705,#46706,#46707,#46708,#46709),
 .UNSPECIFIED.,.F.,.F.,(4,1,1,1,1,1,1,1,1,1,1,1,1,4),(21.9911485751286,
22.3783465135924,22.8770931627562,23.37583981192,23.8745864610838,24.3733331102476,
24.8720797594113,25.3708264085751,25.8695730577389,26.3683197069027,26.8670663560665,
27.3658130052302,27.864559654394,28.2743338823082),.UNSPECIFIED.);
#3063=B_SPLINE_CURVE_WITH_KNOTS('',3,(#46715,#46716,#46717,#46718,#46719,
#46720),.UNSPECIFIED.,.F.,.F.,(4,1,1,4),(14.3984001269719,14.8971467761357,
15.3958934252995,15.7079632679491),.UNSPECIFIED.);
#3064=B_SPLINE_CURVE_WITH_KNOTS('',3,(#46723,#46724,#46725,#46726,#46727,
#46728,#46729),.UNSPECIFIED.,.F.,.F.,(4,1,1,1,4),(13.8759337553363,14.3454669106698,
14.8442135598336,15.3429602089974,15.7079632679491),.UNSPECIFIED.);
#3065=B_SPLINE_CURVE_WITH_KNOTS('',3,(#46731,#46732,#46733,#46734,#46735,
#46736,#46737,#46738,#46739,#46740,#46741,#46742,#46743,#46744,#46745,#46746,
#46747),.UNSPECIFIED.,.F.,.F.,(4,1,1,1,1,1,1,1,1,1,1,1,1,1,4),(15.7079632679491,
15.8417068581612,16.340453507325,16.8392001564888,17.3379468056525,17.8366934548163,
18.3354401039801,18.8341867531439,19.3329334023077,19.8316800514714,20.3304267006352,
20.829173349799,21.3279199989628,21.8266666481266,21.9911485751287),
 .UNSPECIFIED.);
#3066=B_SPLINE_CURVE_WITH_KNOTS('',3,(#46748,#46749,#46750,#46751,#46752,
#46753,#46754,#46755,#46756,#46757,#46758,#46759,#46760,#46761,#46762,#46763,
#46764),.UNSPECIFIED.,.F.,.F.,(4,1,1,1,1,1,1,1,1,1,1,1,1,1,4),(15.7079632679491,
15.8946400744633,16.393386723627,16.8921333727908,17.3908800219546,17.8896266711184,
18.3883733202822,18.887119969446,19.3858666186097,19.8846132677735,20.3833599169373,
20.8821065661011,21.3808532152649,21.8795998644286,21.9911485751286),
 .UNSPECIFIED.);
#3067=B_SPLINE_CURVE_WITH_KNOTS('',3,(#48233,#48234,#48235,#48236,#48237,
#48238,#48239,#48240,#48241,#48242,#48243,#48244,#48245,#48246,#48247,#48248,
#48249,#48250,#48251,#48252,#48253,#48254,#48255,#48256,#48257,#48258,#48259,
#48260,#48261,#48262,#48263,#48264,#48265,#48266,#48267,#48268,#48269,#48270,
#48271,#48272,#48273,#48274,#48275,#48276,#48277,#48278,#48279,#48280,#48281,
#48282,#48283,#48284,#48285,#48286,#48287,#48288,#48289,#48290,#48291,#48292,
#48293,#48294,#48295,#48296,#48297,#48298,#48299,#48300,#48301,#48302,#48303,
#48304,#48305,#48306,#48307,#48308,#48309,#48310,#48311,#48312,#48313,#48314,
#48315,#48316,#48317,#48318,#48319,#48320,#48321,#48322,#48323,#48324,#48325,
#48326,#48327,#48328,#48329,#48330,#48331,#48332,#48333,#48334,#48335,#48336,
#48337,#48338,#48339,#48340,#48341,#48342,#48343,#48344),.UNSPECIFIED.,
 .F.,.F.,(4,3,3,3,3,3,3,3,3,3,3,3,3,3,3,3,3,3,3,3,3,3,3,3,3,3,3,3,3,3,3,
3,3,3,3,3,3,4),(0.,0.0505771409544137,0.101554208126943,0.152189059755351,
0.202216159570862,0.226885015823025,0.234012168591673,0.240461808082327,
0.29007953191694,0.300891584579511,0.350695312223996,0.400404404445326,
0.447850031768845,0.461476807659048,0.467766229912276,0.516330065625832,
0.564490190484642,0.590186913739402,0.638696313987249,0.667316948881319,
0.678175806101206,0.686355565587849,0.733761702748627,0.781038646687326,
0.827499605987411,0.867661393139807,0.884230290042188,0.893713740355506,
0.900277340341249,0.946756252637673,0.993258125372732,1.01069632764838,
1.01980492182733,1.02788458752219,1.07342337960794,1.11826391008869,1.13276374357791,
1.14791015664662),.UNSPECIFIED.);
#3068=B_SPLINE_CURVE_WITH_KNOTS('',3,(#48345,#48346,#48347,#48348,#48349,
#48350,#48351,#48352,#48353,#48354,#48355,#48356,#48357,#48358,#48359,#48360,
#48361,#48362,#48363,#48364,#48365,#48366,#48367,#48368,#48369,#48370,#48371,
#48372,#48373,#48374,#48375,#48376,#48377,#48378,#48379,#48380,#48381,#48382,
#48383,#48384,#48385,#48386,#48387,#48388,#48389,#48390,#48391,#48392,#48393,
#48394,#48395,#48396,#48397,#48398,#48399,#48400,#48401,#48402,#48403,#48404,
#48405,#48406,#48407,#48408,#48409,#48410,#48411,#48412,#48413,#48414,#48415,
#48416,#48417,#48418,#48419,#48420,#48421,#48422,#48423,#48424,#48425,#48426,
#48427,#48428,#48429,#48430,#48431,#48432,#48433,#48434,#48435,#48436,#48437,
#48438,#48439,#48440,#48441,#48442,#48443,#48444,#48445,#48446,#48447,#48448,
#48449,#48450,#48451,#48452,#48453,#48454,#48455,#48456),.UNSPECIFIED.,
 .F.,.F.,(4,3,3,3,3,3,3,3,3,3,3,3,3,3,3,3,3,3,3,3,3,3,3,3,3,3,3,3,3,3,3,
3,3,3,3,3,3,4),(0.,0.0443052074552335,0.0893948843442793,0.135141488872234,
0.180815870205597,0.19390940453382,0.201667660370645,0.207452222581038,
0.254168163209598,0.263945580324931,0.310166557321201,0.356931398910231,
0.40263742170911,0.412236182291169,0.41809909587038,0.465725175667907,0.513886757864765,
0.539755490105746,0.587673806547005,0.617618173044032,0.628955317157287,
0.635419183001384,0.684153162333737,0.73336012390645,0.782633804055213,
0.827228738523219,0.845892924266055,0.856064133573895,0.862657049097381,
0.91218656093736,0.962309907572726,0.982868071148884,0.998253759458264,
1.00640638253346,1.05732616428783,1.10834517305652,1.1258557104086,1.14369947197755),
 .UNSPECIFIED.);
#3069=B_SPLINE_CURVE_WITH_KNOTS('',3,(#48457,#48458,#48459,#48460,#48461,
#48462,#48463,#48464,#48465,#48466,#48467,#48468,#48469,#48470,#48471,#48472,
#48473,#48474,#48475,#48476,#48477,#48478,#48479,#48480,#48481,#48482,#48483,
#48484,#48485,#48486,#48487,#48488,#48489,#48490,#48491,#48492,#48493,#48494,
#48495,#48496,#48497,#48498,#48499),.UNSPECIFIED.,.F.,.F.,(4,3,3,3,3,3,
3,3,3,3,3,3,3,3,4),(-10.1394149102777,-9.97493298327562,-9.47618633411184,
-8.97743968494806,-8.47869303578428,-7.9799463866205,-7.48119973745672,
-6.98245308829294,-6.48370643912916,-5.98495978996538,-5.4862131408016,
-4.98746649163782,-4.48871984247403,-3.98997319331025,-3.85622960309811),
 .UNSPECIFIED.);
#3070=B_SPLINE_CURVE_WITH_KNOTS('',3,(#49968,#49969,#49970,#49971,#49972,
#49973,#49974,#49975,#49976,#49977,#49978,#49979,#49980,#49981,#49982,#49983,
#49984,#49985,#49986,#49987,#49988,#49989,#49990,#49991,#49992,#49993,#49994,
#49995,#49996,#49997,#49998,#49999,#50000,#50001,#50002,#50003,#50004,#50005,
#50006,#50007,#50008,#50009,#50010,#50011,#50012,#50013,#50014,#50015,#50016,
#50017,#50018,#50019,#50020,#50021,#50022,#50023,#50024,#50025,#50026,#50027,
#50028,#50029,#50030,#50031,#50032,#50033,#50034,#50035,#50036,#50037,#50038,
#50039,#50040,#50041,#50042,#50043,#50044,#50045,#50046,#50047,#50048,#50049,
#50050,#50051,#50052,#50053,#50054,#50055,#50056,#50057,#50058,#50059,#50060,
#50061,#50062,#50063,#50064,#50065,#50066,#50067,#50068,#50069,#50070,#50071,
#50072,#50073,#50074,#50075,#50076,#50077,#50078,#50079),.UNSPECIFIED.,
 .F.,.F.,(4,3,3,3,3,3,3,3,3,3,3,3,3,3,3,3,3,3,3,3,3,3,3,3,3,3,3,3,3,3,3,
3,3,3,3,3,3,4),(0.,0.0443052464394431,0.0893949539526172,0.13514156535071,
0.180815937906565,0.19390953278588,0.201668332261212,0.207452743931054,
0.254168704708716,0.263945580324925,0.310166527100594,0.356931351724118,
0.402637386319524,0.412236112021009,0.418099029289404,0.465725083881085,
0.513886660859732,0.539755490105741,0.58767381564034,0.617618181000692,
0.628955400664764,0.635419179939423,0.684153173701215,0.733360142889101,
0.782633822702733,0.827228738523158,0.845892924265991,0.856064134176901,
0.862657049292299,0.912186558109282,0.962309904124215,0.98286806942716,
0.998253758909606,1.00640638216257,1.05732616367401,1.1083451721479,1.12585571040848,
1.14369947197742),.UNSPECIFIED.);
#3071=B_SPLINE_CURVE_WITH_KNOTS('',3,(#50080,#50081,#50082,#50083,#50084,
#50085,#50086,#50087,#50088,#50089,#50090,#50091,#50092,#50093,#50094,#50095,
#50096,#50097,#50098,#50099,#50100,#50101,#50102,#50103,#50104,#50105,#50106,
#50107,#50108,#50109,#50110,#50111,#50112,#50113,#50114,#50115,#50116,#50117,
#50118,#50119),.UNSPECIFIED.,.F.,.F.,(4,3,3,3,3,3,3,3,3,3,3,3,3,4),(7.59274844815678,
7.9799463866205,8.47869303578429,8.97743968494807,9.47618633411185,9.97493298327563,
10.4736796324394,10.9724262816032,11.471172930767,11.9699195799308,12.4686662290945,
12.9674128782583,13.4661595274221,13.8759337553364),.UNSPECIFIED.);
#3072=B_SPLINE_CURVE_WITH_KNOTS('',3,(#50120,#50121,#50122,#50123,#50124,
#50125,#50126,#50127,#50128,#50129,#50130,#50131,#50132,#50133,#50134,#50135,
#50136,#50137,#50138,#50139,#50140,#50141,#50142,#50143,#50144,#50145,#50146,
#50147,#50148,#50149,#50150,#50151,#50152,#50153,#50154,#50155,#50156,#50157,
#50158,#50159,#50160,#50161,#50162,#50163,#50164,#50165,#50166,#50167,#50168,
#50169,#50170,#50171,#50172,#50173,#50174,#50175,#50176,#50177,#50178,#50179,
#50180,#50181,#50182,#50183,#50184,#50185,#50186,#50187,#50188,#50189,#50190,
#50191,#50192,#50193,#50194,#50195,#50196,#50197,#50198,#50199,#50200,#50201,
#50202,#50203,#50204,#50205,#50206,#50207,#50208,#50209,#50210,#50211,#50212,
#50213,#50214,#50215,#50216,#50217,#50218,#50219,#50220,#50221,#50222,#50223,
#50224,#50225,#50226,#50227,#50228,#50229,#50230,#50231),.UNSPECIFIED.,
 .F.,.F.,(4,3,3,3,3,3,3,3,3,3,3,3,3,3,3,3,3,3,3,3,3,3,3,3,3,3,3,3,3,3,3,
3,3,3,3,3,3,4),(0.,0.050577164702863,0.101554237110135,0.152189070454327,
0.202216145640601,0.226885005375326,0.234012130381444,0.240461803926884,
0.290079515630049,0.3008915845795,0.350695306957134,0.400404402970159,0.447850030662475,
0.461476805155705,0.46776622895846,0.516330065384172,0.564490196514962,
0.590186913739423,0.638696314494036,0.667316949324757,0.678175808158324,
0.686355565879716,0.7337617036123,0.781038648491377,0.827499614280347,0.867661393139803,
0.884230290042183,0.893713740915346,0.900277341547724,0.946756255255806,
0.993258127336325,1.01069632936652,1.01980492495367,1.02788458707311,1.07342337690414,
1.11826390001064,1.13276374357788,1.14791015664662),.UNSPECIFIED.);
#3945=LINE('',#43269,#4793);
#3946=LINE('',#43344,#4794);
#3947=LINE('',#43431,#4795);
#3948=LINE('',#43518,#4796);
#3949=LINE('',#43605,#4797);
#3950=LINE('',#43695,#4798);
#3951=LINE('',#43782,#4799);
#3952=LINE('',#43869,#4800);
#3953=LINE('',#43956,#4801);
#3954=LINE('',#44043,#4802);
#3955=LINE('',#44133,#4803);
#3956=LINE('',#44220,#4804);
#3957=LINE('',#44307,#4805);
#3958=LINE('',#44394,#4806);
#3959=LINE('',#44481,#4807);
#3960=LINE('',#44568,#4808);
#3961=LINE('',#44655,#4809);
#3962=LINE('',#44742,#4810);
#3963=LINE('',#44829,#4811);
#3964=LINE('',#44916,#4812);
#3965=LINE('',#45003,#4813);
#3966=LINE('',#45093,#4814);
#3967=LINE('',#45180,#4815);
#3968=LINE('',#45267,#4816);
#3969=LINE('',#45354,#4817);
#3970=LINE('',#45441,#4818);
#3971=LINE('',#45531,#4819);
#3972=LINE('',#45618,#4820);
#3973=LINE('',#45687,#4821);
#3974=LINE('',#45709,#4822);
#3975=LINE('',#45747,#4823);
#3976=LINE('',#45783,#4824);
#3977=LINE('',#45821,#4825);
#3978=LINE('',#45858,#4826);
#3979=LINE('',#45895,#4827);
#3980=LINE('',#45933,#4828);
#3981=LINE('',#45969,#4829);
#3982=LINE('',#46007,#4830);
#3983=LINE('',#46044,#4831);
#3984=LINE('',#46081,#4832);
#3985=LINE('',#46119,#4833);
#3986=LINE('',#46155,#4834);
#3987=LINE('',#46193,#4835);
#3988=LINE('',#46230,#4836);
#3989=LINE('',#46267,#4837);
#3990=LINE('',#46305,#4838);
#3991=LINE('',#46341,#4839);
#3992=LINE('',#46379,#4840);
#3993=LINE('',#46415,#4841);
#3994=LINE('',#46453,#4842);
#3995=LINE('',#46491,#4843);
#3996=LINE('',#46527,#4844);
#3997=LINE('',#46565,#4845);
#3998=LINE('',#46601,#4846);
#3999=LINE('',#46639,#4847);
#4000=LINE('',#46677,#4848);
#4001=LINE('',#46713,#4849);
#4002=LINE('',#50235,#4850);
#4003=LINE('',#50237,#4851);
#4004=LINE('',#50239,#4852);
#4005=LINE('',#50241,#4853);
#4006=LINE('',#50243,#4854);
#4007=LINE('',#50245,#4855);
#4008=LINE('',#50247,#4856);
#4009=LINE('',#50248,#4857);
#4010=LINE('',#50253,#4858);
#4011=LINE('',#50255,#4859);
#4012=LINE('',#50257,#4860);
#4013=LINE('',#50258,#4861);
#4014=LINE('',#50262,#4862);
#4015=LINE('',#50263,#4863);
#4016=LINE('',#50264,#4864);
#4017=LINE('',#50266,#4865);
#4018=LINE('',#50267,#4866);
#4019=LINE('',#50270,#4867);
#4020=LINE('',#50271,#4868);
#4021=LINE('',#50274,#4869);
#4022=LINE('',#50275,#4870);
#4023=LINE('',#50278,#4871);
#4024=LINE('',#50279,#4872);
#4025=LINE('',#50282,#4873);
#4026=LINE('',#50283,#4874);
#4027=LINE('',#50286,#4875);
#4028=LINE('',#50287,#4876);
#4029=LINE('',#50290,#4877);
#4030=LINE('',#50291,#4878);
#4031=LINE('',#50293,#4879);
#4793=VECTOR('',#17297,6.);
#4794=VECTOR('',#17302,6.);
#4795=VECTOR('',#17305,6.);
#4796=VECTOR('',#17308,6.);
#4797=VECTOR('',#17311,6.);
#4798=VECTOR('',#17314,6.);
#4799=VECTOR('',#17317,6.);
#4800=VECTOR('',#17320,6.);
#4801=VECTOR('',#17323,6.);
#4802=VECTOR('',#17326,6.);
#4803=VECTOR('',#17329,6.);
#4804=VECTOR('',#17332,6.);
#4805=VECTOR('',#17335,6.);
#4806=VECTOR('',#17338,6.);
#4807=VECTOR('',#17341,6.);
#4808=VECTOR('',#17344,6.);
#4809=VECTOR('',#17347,6.);
#4810=VECTOR('',#17350,6.);
#4811=VECTOR('',#17353,6.);
#4812=VECTOR('',#17356,6.);
#4813=VECTOR('',#17359,6.);
#4814=VECTOR('',#17362,6.);
#4815=VECTOR('',#17365,6.);
#4816=VECTOR('',#17368,6.);
#4817=VECTOR('',#17371,6.);
#4818=VECTOR('',#17374,6.);
#4819=VECTOR('',#17377,6.);
#4820=VECTOR('',#17380,6.);
#4821=VECTOR('',#17385,6.11325);
#4822=VECTOR('',#17390,6.11325);
#4823=VECTOR('',#17393,6.11325);
#4824=VECTOR('',#17396,6.11325);
#4825=VECTOR('',#17399,6.11325);
#4826=VECTOR('',#17402,6.11325);
#4827=VECTOR('',#17405,6.11325);
#4828=VECTOR('',#17408,6.11325);
#4829=VECTOR('',#17411,6.11325);
#4830=VECTOR('',#17414,6.11325);
#4831=VECTOR('',#17417,6.11325);
#4832=VECTOR('',#17420,6.11325);
#4833=VECTOR('',#17423,6.11325);
#4834=VECTOR('',#17426,6.11325);
#4835=VECTOR('',#17429,6.11325);
#4836=VECTOR('',#17432,6.11325);
#4837=VECTOR('',#17435,6.11325);
#4838=VECTOR('',#17438,6.11325);
#4839=VECTOR('',#17441,6.11325);
#4840=VECTOR('',#17444,6.11325);
#4841=VECTOR('',#17447,6.11325);
#4842=VECTOR('',#17450,6.11325);
#4843=VECTOR('',#17453,6.11325);
#4844=VECTOR('',#17456,6.11325);
#4845=VECTOR('',#17459,6.11325);
#4846=VECTOR('',#17462,6.11325);
#4847=VECTOR('',#17465,6.11325);
#4848=VECTOR('',#17468,6.11325);
#4849=VECTOR('',#17471,6.11325);
#4850=VECTOR('',#17478,10.);
#4851=VECTOR('',#17479,10.);
#4852=VECTOR('',#17480,10.);
#4853=VECTOR('',#17481,10.);
#4854=VECTOR('',#17482,10.);
#4855=VECTOR('',#17483,10.);
#4856=VECTOR('',#17484,10.);
#4857=VECTOR('',#17485,10.);
#4858=VECTOR('',#17490,10.);
#4859=VECTOR('',#17491,10.);
#4860=VECTOR('',#17492,10.);
#4861=VECTOR('',#17493,10.);
#4862=VECTOR('',#17496,10.);
#4863=VECTOR('',#17497,10.);
#4864=VECTOR('',#17498,10.);
#4865=VECTOR('',#17501,10.);
#4866=VECTOR('',#17502,10.);
#4867=VECTOR('',#17505,10.);
#4868=VECTOR('',#17506,10.);
#4869=VECTOR('',#17509,10.);
#4870=VECTOR('',#17510,10.);
#4871=VECTOR('',#17513,10.);
#4872=VECTOR('',#17514,10.);
#4873=VECTOR('',#17517,10.);
#4874=VECTOR('',#17518,10.);
#4875=VECTOR('',#17521,10.);
#4876=VECTOR('',#17522,10.);
#4877=VECTOR('',#17525,10.);
#4878=VECTOR('',#17526,10.);
#4879=VECTOR('',#17529,10.);
#5987=VERTEX_POINT('',#43267);
#5988=VERTEX_POINT('',#43268);
#5989=VERTEX_POINT('',#43270);
#5990=VERTEX_POINT('',#43299);
#5991=VERTEX_POINT('',#43342);
#5992=VERTEX_POINT('',#43343);
#5993=VERTEX_POINT('',#43429);
#5994=VERTEX_POINT('',#43430);
#5995=VERTEX_POINT('',#43516);
#5996=VERTEX_POINT('',#43517);
#5997=VERTEX_POINT('',#43603);
#5998=VERTEX_POINT('',#43604);
#5999=VERTEX_POINT('',#43693);
#6000=VERTEX_POINT('',#43694);
#6001=VERTEX_POINT('',#43780);
#6002=VERTEX_POINT('',#43781);
#6003=VERTEX_POINT('',#43867);
#6004=VERTEX_POINT('',#43868);
#6005=VERTEX_POINT('',#43954);
#6006=VERTEX_POINT('',#43955);
#6007=VERTEX_POINT('',#44041);
#6008=VERTEX_POINT('',#44042);
#6009=VERTEX_POINT('',#44131);
#6010=VERTEX_POINT('',#44132);
#6011=VERTEX_POINT('',#44218);
#6012=VERTEX_POINT('',#44219);
#6013=VERTEX_POINT('',#44305);
#6014=VERTEX_POINT('',#44306);
#6015=VERTEX_POINT('',#44392);
#6016=VERTEX_POINT('',#44393);
#6017=VERTEX_POINT('',#44479);
#6018=VERTEX_POINT('',#44480);
#6019=VERTEX_POINT('',#44566);
#6020=VERTEX_POINT('',#44567);
#6021=VERTEX_POINT('',#44653);
#6022=VERTEX_POINT('',#44654);
#6023=VERTEX_POINT('',#44740);
#6024=VERTEX_POINT('',#44741);
#6025=VERTEX_POINT('',#44827);
#6026=VERTEX_POINT('',#44828);
#6027=VERTEX_POINT('',#44914);
#6028=VERTEX_POINT('',#44915);
#6029=VERTEX_POINT('',#45001);
#6030=VERTEX_POINT('',#45002);
#6031=VERTEX_POINT('',#45091);
#6032=VERTEX_POINT('',#45092);
#6033=VERTEX_POINT('',#45178);
#6034=VERTEX_POINT('',#45179);
#6035=VERTEX_POINT('',#45265);
#6036=VERTEX_POINT('',#45266);
#6037=VERTEX_POINT('',#45352);
#6038=VERTEX_POINT('',#45353);
#6039=VERTEX_POINT('',#45439);
#6040=VERTEX_POINT('',#45440);
#6041=VERTEX_POINT('',#45529);
#6042=VERTEX_POINT('',#45530);
#6043=VERTEX_POINT('',#45616);
#6044=VERTEX_POINT('',#45617);
#6045=VERTEX_POINT('',#45619);
#6046=VERTEX_POINT('',#45645);
#6047=VERTEX_POINT('',#45685);
#6048=VERTEX_POINT('',#45686);
#6049=VERTEX_POINT('',#45688);
#6050=VERTEX_POINT('',#45696);
#6051=VERTEX_POINT('',#45707);
#6052=VERTEX_POINT('',#45708);
#6053=VERTEX_POINT('',#45745);
#6054=VERTEX_POINT('',#45746);
#6055=VERTEX_POINT('',#45781);
#6056=VERTEX_POINT('',#45782);
#6057=VERTEX_POINT('',#45819);
#6058=VERTEX_POINT('',#45820);
#6059=VERTEX_POINT('',#45856);
#6060=VERTEX_POINT('',#45857);
#6061=VERTEX_POINT('',#45893);
#6062=VERTEX_POINT('',#45894);
#6063=VERTEX_POINT('',#45931);
#6064=VERTEX_POINT('',#45932);
#6065=VERTEX_POINT('',#45967);
#6066=VERTEX_POINT('',#45968);
#6067=VERTEX_POINT('',#46005);
#6068=VERTEX_POINT('',#46006);
#6069=VERTEX_POINT('',#46042);
#6070=VERTEX_POINT('',#46043);
#6071=VERTEX_POINT('',#46079);
#6072=VERTEX_POINT('',#46080);
#6073=VERTEX_POINT('',#46117);
#6074=VERTEX_POINT('',#46118);
#6075=VERTEX_POINT('',#46153);
#6076=VERTEX_POINT('',#46154);
#6077=VERTEX_POINT('',#46191);
#6078=VERTEX_POINT('',#46192);
#6079=VERTEX_POINT('',#46228);
#6080=VERTEX_POINT('',#46229);
#6081=VERTEX_POINT('',#46265);
#6082=VERTEX_POINT('',#46266);
#6083=VERTEX_POINT('',#46303);
#6084=VERTEX_POINT('',#46304);
#6085=VERTEX_POINT('',#46339);
#6086=VERTEX_POINT('',#46340);
#6087=VERTEX_POINT('',#46377);
#6088=VERTEX_POINT('',#46378);
#6089=VERTEX_POINT('',#46413);
#6090=VERTEX_POINT('',#46414);
#6091=VERTEX_POINT('',#46451);
#6092=VERTEX_POINT('',#46452);
#6093=VERTEX_POINT('',#46489);
#6094=VERTEX_POINT('',#46490);
#6095=VERTEX_POINT('',#46525);
#6096=VERTEX_POINT('',#46526);
#6097=VERTEX_POINT('',#46563);
#6098=VERTEX_POINT('',#46564);
#6099=VERTEX_POINT('',#46599);
#6100=VERTEX_POINT('',#46600);
#6101=VERTEX_POINT('',#46637);
#6102=VERTEX_POINT('',#46638);
#6103=VERTEX_POINT('',#46675);
#6104=VERTEX_POINT('',#46676);
#6105=VERTEX_POINT('',#46711);
#6106=VERTEX_POINT('',#46712);
#6107=VERTEX_POINT('',#46714);
#6108=VERTEX_POINT('',#46721);
#6109=VERTEX_POINT('',#50233);
#6110=VERTEX_POINT('',#50234);
#6111=VERTEX_POINT('',#50236);
#6112=VERTEX_POINT('',#50238);
#6113=VERTEX_POINT('',#50240);
#6114=VERTEX_POINT('',#50242);
#6115=VERTEX_POINT('',#50244);
#6116=VERTEX_POINT('',#50246);
#6117=VERTEX_POINT('',#50251);
#6118=VERTEX_POINT('',#50252);
#6119=VERTEX_POINT('',#50254);
#6120=VERTEX_POINT('',#50256);
#6121=VERTEX_POINT('',#50260);
#6122=VERTEX_POINT('',#50261);
#6123=VERTEX_POINT('',#50269);
#6124=VERTEX_POINT('',#50273);
#6125=VERTEX_POINT('',#50277);
#6126=VERTEX_POINT('',#50281);
#6127=VERTEX_POINT('',#50285);
#6128=VERTEX_POINT('',#50289);
#7855=EDGE_CURVE('',#5987,#5988,#3945,.T.);
#7856=EDGE_CURVE('',#5988,#5989,#2951,.T.);
#7857=EDGE_CURVE('',#5990,#5989,#2287,.T.);
#7858=EDGE_CURVE('',#5990,#5987,#2952,.T.);
#7859=EDGE_CURVE('',#5991,#5992,#3946,.T.);
#7860=EDGE_CURVE('',#5992,#5988,#2953,.T.);
#7861=EDGE_CURVE('',#5987,#5991,#2954,.T.);
#7862=EDGE_CURVE('',#5993,#5994,#3947,.T.);
#7863=EDGE_CURVE('',#5994,#5992,#2955,.T.);
#7864=EDGE_CURVE('',#5991,#5993,#2956,.T.);
#7865=EDGE_CURVE('',#5995,#5996,#3948,.T.);
#7866=EDGE_CURVE('',#5996,#5994,#2957,.T.);
#7867=EDGE_CURVE('',#5993,#5995,#2958,.T.);
#7868=EDGE_CURVE('',#5997,#5998,#3949,.T.);
#7869=EDGE_CURVE('',#5998,#5996,#2959,.T.);
#7870=EDGE_CURVE('',#5995,#5997,#2960,.T.);
#7871=EDGE_CURVE('',#5999,#6000,#3950,.T.);
#7872=EDGE_CURVE('',#6000,#5998,#2961,.T.);
#7873=EDGE_CURVE('',#5997,#5999,#2962,.T.);
#7874=EDGE_CURVE('',#6001,#6002,#3951,.T.);
#7875=EDGE_CURVE('',#6002,#6000,#2963,.T.);
#7876=EDGE_CURVE('',#5999,#6001,#2964,.T.);
#7877=EDGE_CURVE('',#6003,#6004,#3952,.T.);
#7878=EDGE_CURVE('',#6004,#6002,#2965,.T.);
#7879=EDGE_CURVE('',#6001,#6003,#2966,.T.);
#7880=EDGE_CURVE('',#6005,#6006,#3953,.T.);
#7881=EDGE_CURVE('',#6006,#6004,#2967,.T.);
#7882=EDGE_CURVE('',#6003,#6005,#2968,.T.);
#7883=EDGE_CURVE('',#6007,#6008,#3954,.T.);
#7884=EDGE_CURVE('',#6008,#6006,#2969,.T.);
#7885=EDGE_CURVE('',#6005,#6007,#2970,.T.);
#7886=EDGE_CURVE('',#6009,#6010,#3955,.T.);
#7887=EDGE_CURVE('',#6010,#6008,#2971,.T.);
#7888=EDGE_CURVE('',#6007,#6009,#2972,.T.);
#7889=EDGE_CURVE('',#6011,#6012,#3956,.T.);
#7890=EDGE_CURVE('',#6012,#6010,#2973,.T.);
#7891=EDGE_CURVE('',#6009,#6011,#2974,.T.);
#7892=EDGE_CURVE('',#6013,#6014,#3957,.T.);
#7893=EDGE_CURVE('',#6014,#6012,#2975,.T.);
#7894=EDGE_CURVE('',#6011,#6013,#2976,.T.);
#7895=EDGE_CURVE('',#6015,#6016,#3958,.T.);
#7896=EDGE_CURVE('',#6016,#6014,#2977,.T.);
#7897=EDGE_CURVE('',#6013,#6015,#2978,.T.);
#7898=EDGE_CURVE('',#6017,#6018,#3959,.T.);
#7899=EDGE_CURVE('',#6018,#6016,#2979,.T.);
#7900=EDGE_CURVE('',#6015,#6017,#2980,.T.);
#7901=EDGE_CURVE('',#6019,#6020,#3960,.T.);
#7902=EDGE_CURVE('',#6020,#6018,#2981,.T.);
#7903=EDGE_CURVE('',#6017,#6019,#2982,.T.);
#7904=EDGE_CURVE('',#6021,#6022,#3961,.T.);
#7905=EDGE_CURVE('',#6022,#6020,#2983,.T.);
#7906=EDGE_CURVE('',#6019,#6021,#2984,.T.);
#7907=EDGE_CURVE('',#6023,#6024,#3962,.T.);
#7908=EDGE_CURVE('',#6024,#6022,#2985,.T.);
#7909=EDGE_CURVE('',#6021,#6023,#2986,.T.);
#7910=EDGE_CURVE('',#6025,#6026,#3963,.T.);
#7911=EDGE_CURVE('',#6026,#6024,#2987,.T.);
#7912=EDGE_CURVE('',#6023,#6025,#2988,.T.);
#7913=EDGE_CURVE('',#6027,#6028,#3964,.T.);
#7914=EDGE_CURVE('',#6028,#6026,#2989,.T.);
#7915=EDGE_CURVE('',#6025,#6027,#2990,.T.);
#7916=EDGE_CURVE('',#6029,#6030,#3965,.T.);
#7917=EDGE_CURVE('',#6030,#6028,#2991,.T.);
#7918=EDGE_CURVE('',#6027,#6029,#2992,.T.);
#7919=EDGE_CURVE('',#6031,#6032,#3966,.T.);
#7920=EDGE_CURVE('',#6032,#6030,#2993,.T.);
#7921=EDGE_CURVE('',#6029,#6031,#2994,.T.);
#7922=EDGE_CURVE('',#6033,#6034,#3967,.T.);
#7923=EDGE_CURVE('',#6034,#6032,#2995,.T.);
#7924=EDGE_CURVE('',#6031,#6033,#2996,.T.);
#7925=EDGE_CURVE('',#6035,#6036,#3968,.T.);
#7926=EDGE_CURVE('',#6036,#6034,#2997,.T.);
#7927=EDGE_CURVE('',#6033,#6035,#2998,.T.);
#7928=EDGE_CURVE('',#6037,#6038,#3969,.T.);
#7929=EDGE_CURVE('',#6038,#6036,#2999,.T.);
#7930=EDGE_CURVE('',#6035,#6037,#3000,.T.);
#7931=EDGE_CURVE('',#6039,#6040,#3970,.T.);
#7932=EDGE_CURVE('',#6040,#6038,#3001,.T.);
#7933=EDGE_CURVE('',#6037,#6039,#3002,.T.);
#7934=EDGE_CURVE('',#6041,#6042,#3971,.T.);
#7935=EDGE_CURVE('',#6042,#6040,#3003,.T.);
#7936=EDGE_CURVE('',#6039,#6041,#3004,.T.);
#7937=EDGE_CURVE('',#6043,#6044,#3972,.T.);
#7938=EDGE_CURVE('',#6043,#6045,#3005,.T.);
#7939=EDGE_CURVE('',#6046,#6045,#2288,.T.);
#7940=EDGE_CURVE('',#6046,#6044,#3006,.T.);
#7941=EDGE_CURVE('',#6047,#6048,#3973,.T.);
#7942=EDGE_CURVE('',#6048,#6049,#3007,.T.);
#7943=EDGE_CURVE('',#6050,#6049,#2289,.T.);
#7944=EDGE_CURVE('',#6047,#6050,#3008,.T.);
#7945=EDGE_CURVE('',#6051,#6052,#3974,.T.);
#7946=EDGE_CURVE('',#6052,#6048,#3009,.T.);
#7947=EDGE_CURVE('',#6051,#6047,#3010,.T.);
#7948=EDGE_CURVE('',#6053,#6054,#3975,.T.);
#7949=EDGE_CURVE('',#6054,#6052,#3011,.T.);
#7950=EDGE_CURVE('',#6053,#6051,#3012,.T.);
#7951=EDGE_CURVE('',#6055,#6056,#3976,.T.);
#7952=EDGE_CURVE('',#6056,#6054,#3013,.T.);
#7953=EDGE_CURVE('',#6055,#6053,#3014,.T.);
#7954=EDGE_CURVE('',#6057,#6058,#3977,.T.);
#7955=EDGE_CURVE('',#6058,#6056,#3015,.T.);
#7956=EDGE_CURVE('',#6057,#6055,#3016,.T.);
#7957=EDGE_CURVE('',#6059,#6060,#3978,.T.);
#7958=EDGE_CURVE('',#6060,#6058,#3017,.T.);
#7959=EDGE_CURVE('',#6059,#6057,#3018,.T.);
#7960=EDGE_CURVE('',#6061,#6062,#3979,.T.);
#7961=EDGE_CURVE('',#6062,#6060,#3019,.T.);
#7962=EDGE_CURVE('',#6061,#6059,#3020,.T.);
#7963=EDGE_CURVE('',#6063,#6064,#3980,.T.);
#7964=EDGE_CURVE('',#6064,#6062,#3021,.T.);
#7965=EDGE_CURVE('',#6063,#6061,#3022,.T.);
#7966=EDGE_CURVE('',#6065,#6066,#3981,.T.);
#7967=EDGE_CURVE('',#6066,#6064,#3023,.T.);
#7968=EDGE_CURVE('',#6065,#6063,#3024,.T.);
#7969=EDGE_CURVE('',#6067,#6068,#3982,.T.);
#7970=EDGE_CURVE('',#6068,#6066,#3025,.T.);
#7971=EDGE_CURVE('',#6067,#6065,#3026,.T.);
#7972=EDGE_CURVE('',#6069,#6070,#3983,.T.);
#7973=EDGE_CURVE('',#6070,#6068,#3027,.T.);
#7974=EDGE_CURVE('',#6069,#6067,#3028,.T.);
#7975=EDGE_CURVE('',#6071,#6072,#3984,.T.);
#7976=EDGE_CURVE('',#6072,#6070,#3029,.T.);
#7977=EDGE_CURVE('',#6071,#6069,#3030,.T.);
#7978=EDGE_CURVE('',#6073,#6074,#3985,.T.);
#7979=EDGE_CURVE('',#6074,#6072,#3031,.T.);
#7980=EDGE_CURVE('',#6073,#6071,#3032,.T.);
#7981=EDGE_CURVE('',#6075,#6076,#3986,.T.);
#7982=EDGE_CURVE('',#6076,#6074,#3033,.T.);
#7983=EDGE_CURVE('',#6075,#6073,#3034,.T.);
#7984=EDGE_CURVE('',#6077,#6078,#3987,.T.);
#7985=EDGE_CURVE('',#6078,#6076,#3035,.T.);
#7986=EDGE_CURVE('',#6077,#6075,#3036,.T.);
#7987=EDGE_CURVE('',#6079,#6080,#3988,.T.);
#7988=EDGE_CURVE('',#6080,#6078,#3037,.T.);
#7989=EDGE_CURVE('',#6079,#6077,#3038,.T.);
#7990=EDGE_CURVE('',#6081,#6082,#3989,.T.);
#7991=EDGE_CURVE('',#6082,#6080,#3039,.T.);
#7992=EDGE_CURVE('',#6081,#6079,#3040,.T.);
#7993=EDGE_CURVE('',#6083,#6084,#3990,.T.);
#7994=EDGE_CURVE('',#6084,#6082,#3041,.T.);
#7995=EDGE_CURVE('',#6083,#6081,#3042,.T.);
#7996=EDGE_CURVE('',#6085,#6086,#3991,.T.);
#7997=EDGE_CURVE('',#6086,#6084,#3043,.T.);
#7998=EDGE_CURVE('',#6085,#6083,#3044,.T.);
#7999=EDGE_CURVE('',#6087,#6088,#3992,.T.);
#8000=EDGE_CURVE('',#6088,#6086,#3045,.T.);
#8001=EDGE_CURVE('',#6087,#6085,#3046,.T.);
#8002=EDGE_CURVE('',#6089,#6090,#3993,.T.);
#8003=EDGE_CURVE('',#6090,#6088,#3047,.T.);
#8004=EDGE_CURVE('',#6089,#6087,#3048,.T.);
#8005=EDGE_CURVE('',#6091,#6092,#3994,.T.);
#8006=EDGE_CURVE('',#6092,#6090,#3049,.T.);
#8007=EDGE_CURVE('',#6091,#6089,#3050,.T.);
#8008=EDGE_CURVE('',#6093,#6094,#3995,.T.);
#8009=EDGE_CURVE('',#6094,#6092,#3051,.T.);
#8010=EDGE_CURVE('',#6093,#6091,#3052,.T.);
#8011=EDGE_CURVE('',#6095,#6096,#3996,.T.);
#8012=EDGE_CURVE('',#6096,#6094,#3053,.T.);
#8013=EDGE_CURVE('',#6095,#6093,#3054,.T.);
#8014=EDGE_CURVE('',#6097,#6098,#3997,.T.);
#8015=EDGE_CURVE('',#6098,#6096,#3055,.T.);
#8016=EDGE_CURVE('',#6097,#6095,#3056,.T.);
#8017=EDGE_CURVE('',#6099,#6100,#3998,.T.);
#8018=EDGE_CURVE('',#6100,#6098,#3057,.T.);
#8019=EDGE_CURVE('',#6099,#6097,#3058,.T.);
#8020=EDGE_CURVE('',#6101,#6102,#3999,.T.);
#8021=EDGE_CURVE('',#6102,#6100,#3059,.T.);
#8022=EDGE_CURVE('',#6101,#6099,#3060,.T.);
#8023=EDGE_CURVE('',#6103,#6104,#4000,.T.);
#8024=EDGE_CURVE('',#6104,#6102,#3061,.T.);
#8025=EDGE_CURVE('',#6103,#6101,#3062,.T.);
#8026=EDGE_CURVE('',#6105,#6106,#4001,.T.);
#8027=EDGE_CURVE('',#6107,#6105,#3063,.T.);
#8028=EDGE_CURVE('',#6108,#6107,#2290,.T.);
#8029=EDGE_CURVE('',#6108,#6106,#3064,.T.);
#8030=EDGE_CURVE('',#6106,#6104,#3065,.T.);
#8031=EDGE_CURVE('',#6105,#6103,#3066,.T.);
#8032=EDGE_CURVE('',#6049,#5990,#3067,.T.);
#8033=EDGE_CURVE('',#6045,#6108,#3068,.T.);
#8034=EDGE_CURVE('',#6041,#6043,#3069,.T.);
#8035=EDGE_CURVE('',#5989,#6050,#3070,.T.);
#8036=EDGE_CURVE('',#6044,#6042,#3071,.T.);
#8037=EDGE_CURVE('',#6107,#6046,#3072,.T.);
#8038=EDGE_CURVE('',#6109,#6110,#4002,.T.);
#8039=EDGE_CURVE('',#6110,#6111,#4003,.T.);
#8040=EDGE_CURVE('',#6112,#6111,#4004,.T.);
#8041=EDGE_CURVE('',#6112,#6113,#4005,.T.);
#8042=EDGE_CURVE('',#6114,#6113,#4006,.T.);
#8043=EDGE_CURVE('',#6115,#6114,#4007,.T.);
#8044=EDGE_CURVE('',#6116,#6115,#4008,.T.);
#8045=EDGE_CURVE('',#6109,#6116,#4009,.T.);
#8046=EDGE_CURVE('',#6117,#6118,#4010,.T.);
#8047=EDGE_CURVE('',#6117,#6119,#4011,.T.);
#8048=EDGE_CURVE('',#6120,#6119,#4012,.T.);
#8049=EDGE_CURVE('',#6118,#6120,#4013,.T.);
#8050=EDGE_CURVE('',#6121,#6122,#4014,.T.);
#8051=EDGE_CURVE('',#6122,#6120,#4015,.T.);
#8052=EDGE_CURVE('',#6119,#6121,#4016,.T.);
#8053=EDGE_CURVE('',#6118,#6114,#4017,.T.);
#8054=EDGE_CURVE('',#6113,#6117,#4018,.T.);
#8055=EDGE_CURVE('',#6123,#6112,#4019,.T.);
#8056=EDGE_CURVE('',#6123,#6121,#4020,.T.);
#8057=EDGE_CURVE('',#6115,#6124,#4021,.T.);
#8058=EDGE_CURVE('',#6124,#6122,#4022,.T.);
#8059=EDGE_CURVE('',#6111,#6125,#4023,.T.);
#8060=EDGE_CURVE('',#6125,#6123,#4024,.T.);
#8061=EDGE_CURVE('',#6124,#6126,#4025,.T.);
#8062=EDGE_CURVE('',#6126,#6116,#4026,.T.);
#8063=EDGE_CURVE('',#6110,#6127,#4027,.T.);
#8064=EDGE_CURVE('',#6127,#6125,#4028,.T.);
#8065=EDGE_CURVE('',#6128,#6109,#4029,.T.);
#8066=EDGE_CURVE('',#6128,#6126,#4030,.T.);
#8067=EDGE_CURVE('',#6127,#6128,#4031,.T.);
#11237=ORIENTED_EDGE('',*,*,#7855,.T.);
#11238=ORIENTED_EDGE('',*,*,#7856,.T.);
#11239=ORIENTED_EDGE('',*,*,#7857,.F.);
#11240=ORIENTED_EDGE('',*,*,#7858,.T.);
#11241=ORIENTED_EDGE('',*,*,#7859,.T.);
#11242=ORIENTED_EDGE('',*,*,#7860,.T.);
#11243=ORIENTED_EDGE('',*,*,#7855,.F.);
#11244=ORIENTED_EDGE('',*,*,#7861,.T.);
#11245=ORIENTED_EDGE('',*,*,#7862,.T.);
#11246=ORIENTED_EDGE('',*,*,#7863,.T.);
#11247=ORIENTED_EDGE('',*,*,#7859,.F.);
#11248=ORIENTED_EDGE('',*,*,#7864,.T.);
#11249=ORIENTED_EDGE('',*,*,#7865,.T.);
#11250=ORIENTED_EDGE('',*,*,#7866,.T.);
#11251=ORIENTED_EDGE('',*,*,#7862,.F.);
#11252=ORIENTED_EDGE('',*,*,#7867,.T.);
#11253=ORIENTED_EDGE('',*,*,#7868,.T.);
#11254=ORIENTED_EDGE('',*,*,#7869,.T.);
#11255=ORIENTED_EDGE('',*,*,#7865,.F.);
#11256=ORIENTED_EDGE('',*,*,#7870,.T.);
#11257=ORIENTED_EDGE('',*,*,#7871,.T.);
#11258=ORIENTED_EDGE('',*,*,#7872,.T.);
#11259=ORIENTED_EDGE('',*,*,#7868,.F.);
#11260=ORIENTED_EDGE('',*,*,#7873,.T.);
#11261=ORIENTED_EDGE('',*,*,#7874,.T.);
#11262=ORIENTED_EDGE('',*,*,#7875,.T.);
#11263=ORIENTED_EDGE('',*,*,#7871,.F.);
#11264=ORIENTED_EDGE('',*,*,#7876,.T.);
#11265=ORIENTED_EDGE('',*,*,#7877,.T.);
#11266=ORIENTED_EDGE('',*,*,#7878,.T.);
#11267=ORIENTED_EDGE('',*,*,#7874,.F.);
#11268=ORIENTED_EDGE('',*,*,#7879,.T.);
#11269=ORIENTED_EDGE('',*,*,#7880,.T.);
#11270=ORIENTED_EDGE('',*,*,#7881,.T.);
#11271=ORIENTED_EDGE('',*,*,#7877,.F.);
#11272=ORIENTED_EDGE('',*,*,#7882,.T.);
#11273=ORIENTED_EDGE('',*,*,#7883,.T.);
#11274=ORIENTED_EDGE('',*,*,#7884,.T.);
#11275=ORIENTED_EDGE('',*,*,#7880,.F.);
#11276=ORIENTED_EDGE('',*,*,#7885,.T.);
#11277=ORIENTED_EDGE('',*,*,#7886,.T.);
#11278=ORIENTED_EDGE('',*,*,#7887,.T.);
#11279=ORIENTED_EDGE('',*,*,#7883,.F.);
#11280=ORIENTED_EDGE('',*,*,#7888,.T.);
#11281=ORIENTED_EDGE('',*,*,#7889,.T.);
#11282=ORIENTED_EDGE('',*,*,#7890,.T.);
#11283=ORIENTED_EDGE('',*,*,#7886,.F.);
#11284=ORIENTED_EDGE('',*,*,#7891,.T.);
#11285=ORIENTED_EDGE('',*,*,#7892,.T.);
#11286=ORIENTED_EDGE('',*,*,#7893,.T.);
#11287=ORIENTED_EDGE('',*,*,#7889,.F.);
#11288=ORIENTED_EDGE('',*,*,#7894,.T.);
#11289=ORIENTED_EDGE('',*,*,#7895,.T.);
#11290=ORIENTED_EDGE('',*,*,#7896,.T.);
#11291=ORIENTED_EDGE('',*,*,#7892,.F.);
#11292=ORIENTED_EDGE('',*,*,#7897,.T.);
#11293=ORIENTED_EDGE('',*,*,#7898,.T.);
#11294=ORIENTED_EDGE('',*,*,#7899,.T.);
#11295=ORIENTED_EDGE('',*,*,#7895,.F.);
#11296=ORIENTED_EDGE('',*,*,#7900,.T.);
#11297=ORIENTED_EDGE('',*,*,#7901,.T.);
#11298=ORIENTED_EDGE('',*,*,#7902,.T.);
#11299=ORIENTED_EDGE('',*,*,#7898,.F.);
#11300=ORIENTED_EDGE('',*,*,#7903,.T.);
#11301=ORIENTED_EDGE('',*,*,#7904,.T.);
#11302=ORIENTED_EDGE('',*,*,#7905,.T.);
#11303=ORIENTED_EDGE('',*,*,#7901,.F.);
#11304=ORIENTED_EDGE('',*,*,#7906,.T.);
#11305=ORIENTED_EDGE('',*,*,#7907,.T.);
#11306=ORIENTED_EDGE('',*,*,#7908,.T.);
#11307=ORIENTED_EDGE('',*,*,#7904,.F.);
#11308=ORIENTED_EDGE('',*,*,#7909,.T.);
#11309=ORIENTED_EDGE('',*,*,#7910,.T.);
#11310=ORIENTED_EDGE('',*,*,#7911,.T.);
#11311=ORIENTED_EDGE('',*,*,#7907,.F.);
#11312=ORIENTED_EDGE('',*,*,#7912,.T.);
#11313=ORIENTED_EDGE('',*,*,#7913,.T.);
#11314=ORIENTED_EDGE('',*,*,#7914,.T.);
#11315=ORIENTED_EDGE('',*,*,#7910,.F.);
#11316=ORIENTED_EDGE('',*,*,#7915,.T.);
#11317=ORIENTED_EDGE('',*,*,#7916,.T.);
#11318=ORIENTED_EDGE('',*,*,#7917,.T.);
#11319=ORIENTED_EDGE('',*,*,#7913,.F.);
#11320=ORIENTED_EDGE('',*,*,#7918,.T.);
#11321=ORIENTED_EDGE('',*,*,#7919,.T.);
#11322=ORIENTED_EDGE('',*,*,#7920,.T.);
#11323=ORIENTED_EDGE('',*,*,#7916,.F.);
#11324=ORIENTED_EDGE('',*,*,#7921,.T.);
#11325=ORIENTED_EDGE('',*,*,#7922,.T.);
#11326=ORIENTED_EDGE('',*,*,#7923,.T.);
#11327=ORIENTED_EDGE('',*,*,#7919,.F.);
#11328=ORIENTED_EDGE('',*,*,#7924,.T.);
#11329=ORIENTED_EDGE('',*,*,#7925,.T.);
#11330=ORIENTED_EDGE('',*,*,#7926,.T.);
#11331=ORIENTED_EDGE('',*,*,#7922,.F.);
#11332=ORIENTED_EDGE('',*,*,#7927,.T.);
#11333=ORIENTED_EDGE('',*,*,#7928,.T.);
#11334=ORIENTED_EDGE('',*,*,#7929,.T.);
#11335=ORIENTED_EDGE('',*,*,#7925,.F.);
#11336=ORIENTED_EDGE('',*,*,#7930,.T.);
#11337=ORIENTED_EDGE('',*,*,#7931,.T.);
#11338=ORIENTED_EDGE('',*,*,#7932,.T.);
#11339=ORIENTED_EDGE('',*,*,#7928,.F.);
#11340=ORIENTED_EDGE('',*,*,#7933,.T.);
#11341=ORIENTED_EDGE('',*,*,#7934,.T.);
#11342=ORIENTED_EDGE('',*,*,#7935,.T.);
#11343=ORIENTED_EDGE('',*,*,#7931,.F.);
#11344=ORIENTED_EDGE('',*,*,#7936,.T.);
#11345=ORIENTED_EDGE('',*,*,#7937,.F.);
#11346=ORIENTED_EDGE('',*,*,#7938,.T.);
#11347=ORIENTED_EDGE('',*,*,#7939,.F.);
#11348=ORIENTED_EDGE('',*,*,#7940,.T.);
#11349=ORIENTED_EDGE('',*,*,#7941,.T.);
#11350=ORIENTED_EDGE('',*,*,#7942,.T.);
#11351=ORIENTED_EDGE('',*,*,#7943,.F.);
#11352=ORIENTED_EDGE('',*,*,#7944,.F.);
#11353=ORIENTED_EDGE('',*,*,#7945,.T.);
#11354=ORIENTED_EDGE('',*,*,#7946,.T.);
#11355=ORIENTED_EDGE('',*,*,#7941,.F.);
#11356=ORIENTED_EDGE('',*,*,#7947,.F.);
#11357=ORIENTED_EDGE('',*,*,#7948,.T.);
#11358=ORIENTED_EDGE('',*,*,#7949,.T.);
#11359=ORIENTED_EDGE('',*,*,#7945,.F.);
#11360=ORIENTED_EDGE('',*,*,#7950,.F.);
#11361=ORIENTED_EDGE('',*,*,#7951,.T.);
#11362=ORIENTED_EDGE('',*,*,#7952,.T.);
#11363=ORIENTED_EDGE('',*,*,#7948,.F.);
#11364=ORIENTED_EDGE('',*,*,#7953,.F.);
#11365=ORIENTED_EDGE('',*,*,#7954,.T.);
#11366=ORIENTED_EDGE('',*,*,#7955,.T.);
#11367=ORIENTED_EDGE('',*,*,#7951,.F.);
#11368=ORIENTED_EDGE('',*,*,#7956,.F.);
#11369=ORIENTED_EDGE('',*,*,#7957,.T.);
#11370=ORIENTED_EDGE('',*,*,#7958,.T.);
#11371=ORIENTED_EDGE('',*,*,#7954,.F.);
#11372=ORIENTED_EDGE('',*,*,#7959,.F.);
#11373=ORIENTED_EDGE('',*,*,#7960,.T.);
#11374=ORIENTED_EDGE('',*,*,#7961,.T.);
#11375=ORIENTED_EDGE('',*,*,#7957,.F.);
#11376=ORIENTED_EDGE('',*,*,#7962,.F.);
#11377=ORIENTED_EDGE('',*,*,#7963,.T.);
#11378=ORIENTED_EDGE('',*,*,#7964,.T.);
#11379=ORIENTED_EDGE('',*,*,#7960,.F.);
#11380=ORIENTED_EDGE('',*,*,#7965,.F.);
#11381=ORIENTED_EDGE('',*,*,#7966,.T.);
#11382=ORIENTED_EDGE('',*,*,#7967,.T.);
#11383=ORIENTED_EDGE('',*,*,#7963,.F.);
#11384=ORIENTED_EDGE('',*,*,#7968,.F.);
#11385=ORIENTED_EDGE('',*,*,#7969,.T.);
#11386=ORIENTED_EDGE('',*,*,#7970,.T.);
#11387=ORIENTED_EDGE('',*,*,#7966,.F.);
#11388=ORIENTED_EDGE('',*,*,#7971,.F.);
#11389=ORIENTED_EDGE('',*,*,#7972,.T.);
#11390=ORIENTED_EDGE('',*,*,#7973,.T.);
#11391=ORIENTED_EDGE('',*,*,#7969,.F.);
#11392=ORIENTED_EDGE('',*,*,#7974,.F.);
#11393=ORIENTED_EDGE('',*,*,#7975,.T.);
#11394=ORIENTED_EDGE('',*,*,#7976,.T.);
#11395=ORIENTED_EDGE('',*,*,#7972,.F.);
#11396=ORIENTED_EDGE('',*,*,#7977,.F.);
#11397=ORIENTED_EDGE('',*,*,#7978,.T.);
#11398=ORIENTED_EDGE('',*,*,#7979,.T.);
#11399=ORIENTED_EDGE('',*,*,#7975,.F.);
#11400=ORIENTED_EDGE('',*,*,#7980,.F.);
#11401=ORIENTED_EDGE('',*,*,#7981,.T.);
#11402=ORIENTED_EDGE('',*,*,#7982,.T.);
#11403=ORIENTED_EDGE('',*,*,#7978,.F.);
#11404=ORIENTED_EDGE('',*,*,#7983,.F.);
#11405=ORIENTED_EDGE('',*,*,#7984,.T.);
#11406=ORIENTED_EDGE('',*,*,#7985,.T.);
#11407=ORIENTED_EDGE('',*,*,#7981,.F.);
#11408=ORIENTED_EDGE('',*,*,#7986,.F.);
#11409=ORIENTED_EDGE('',*,*,#7987,.T.);
#11410=ORIENTED_EDGE('',*,*,#7988,.T.);
#11411=ORIENTED_EDGE('',*,*,#7984,.F.);
#11412=ORIENTED_EDGE('',*,*,#7989,.F.);
#11413=ORIENTED_EDGE('',*,*,#7990,.T.);
#11414=ORIENTED_EDGE('',*,*,#7991,.T.);
#11415=ORIENTED_EDGE('',*,*,#7987,.F.);
#11416=ORIENTED_EDGE('',*,*,#7992,.F.);
#11417=ORIENTED_EDGE('',*,*,#7993,.T.);
#11418=ORIENTED_EDGE('',*,*,#7994,.T.);
#11419=ORIENTED_EDGE('',*,*,#7990,.F.);
#11420=ORIENTED_EDGE('',*,*,#7995,.F.);
#11421=ORIENTED_EDGE('',*,*,#7996,.T.);
#11422=ORIENTED_EDGE('',*,*,#7997,.T.);
#11423=ORIENTED_EDGE('',*,*,#7993,.F.);
#11424=ORIENTED_EDGE('',*,*,#7998,.F.);
#11425=ORIENTED_EDGE('',*,*,#7999,.T.);
#11426=ORIENTED_EDGE('',*,*,#8000,.T.);
#11427=ORIENTED_EDGE('',*,*,#7996,.F.);
#11428=ORIENTED_EDGE('',*,*,#8001,.F.);
#11429=ORIENTED_EDGE('',*,*,#8002,.T.);
#11430=ORIENTED_EDGE('',*,*,#8003,.T.);
#11431=ORIENTED_EDGE('',*,*,#7999,.F.);
#11432=ORIENTED_EDGE('',*,*,#8004,.F.);
#11433=ORIENTED_EDGE('',*,*,#8005,.T.);
#11434=ORIENTED_EDGE('',*,*,#8006,.T.);
#11435=ORIENTED_EDGE('',*,*,#8002,.F.);
#11436=ORIENTED_EDGE('',*,*,#8007,.F.);
#11437=ORIENTED_EDGE('',*,*,#8008,.T.);
#11438=ORIENTED_EDGE('',*,*,#8009,.T.);
#11439=ORIENTED_EDGE('',*,*,#8005,.F.);
#11440=ORIENTED_EDGE('',*,*,#8010,.F.);
#11441=ORIENTED_EDGE('',*,*,#8011,.T.);
#11442=ORIENTED_EDGE('',*,*,#8012,.T.);
#11443=ORIENTED_EDGE('',*,*,#8008,.F.);
#11444=ORIENTED_EDGE('',*,*,#8013,.F.);
#11445=ORIENTED_EDGE('',*,*,#8014,.T.);
#11446=ORIENTED_EDGE('',*,*,#8015,.T.);
#11447=ORIENTED_EDGE('',*,*,#8011,.F.);
#11448=ORIENTED_EDGE('',*,*,#8016,.F.);
#11449=ORIENTED_EDGE('',*,*,#8017,.T.);
#11450=ORIENTED_EDGE('',*,*,#8018,.T.);
#11451=ORIENTED_EDGE('',*,*,#8014,.F.);
#11452=ORIENTED_EDGE('',*,*,#8019,.F.);
#11453=ORIENTED_EDGE('',*,*,#8020,.T.);
#11454=ORIENTED_EDGE('',*,*,#8021,.T.);
#11455=ORIENTED_EDGE('',*,*,#8017,.F.);
#11456=ORIENTED_EDGE('',*,*,#8022,.F.);
#11457=ORIENTED_EDGE('',*,*,#8023,.T.);
#11458=ORIENTED_EDGE('',*,*,#8024,.T.);
#11459=ORIENTED_EDGE('',*,*,#8020,.F.);
#11460=ORIENTED_EDGE('',*,*,#8025,.F.);
#11461=ORIENTED_EDGE('',*,*,#8026,.F.);
#11462=ORIENTED_EDGE('',*,*,#8027,.F.);
#11463=ORIENTED_EDGE('',*,*,#8028,.F.);
#11464=ORIENTED_EDGE('',*,*,#8029,.T.);
#11465=ORIENTED_EDGE('',*,*,#8026,.T.);
#11466=ORIENTED_EDGE('',*,*,#8030,.T.);
#11467=ORIENTED_EDGE('',*,*,#8023,.F.);
#11468=ORIENTED_EDGE('',*,*,#8031,.F.);
#11469=ORIENTED_EDGE('',*,*,#8032,.F.);
#11470=ORIENTED_EDGE('',*,*,#7942,.F.);
#11471=ORIENTED_EDGE('',*,*,#7946,.F.);
#11472=ORIENTED_EDGE('',*,*,#7949,.F.);
#11473=ORIENTED_EDGE('',*,*,#7952,.F.);
#11474=ORIENTED_EDGE('',*,*,#7955,.F.);
#11475=ORIENTED_EDGE('',*,*,#7958,.F.);
#11476=ORIENTED_EDGE('',*,*,#7961,.F.);
#11477=ORIENTED_EDGE('',*,*,#7964,.F.);
#11478=ORIENTED_EDGE('',*,*,#7967,.F.);
#11479=ORIENTED_EDGE('',*,*,#7970,.F.);
#11480=ORIENTED_EDGE('',*,*,#7973,.F.);
#11481=ORIENTED_EDGE('',*,*,#7976,.F.);
#11482=ORIENTED_EDGE('',*,*,#7979,.F.);
#11483=ORIENTED_EDGE('',*,*,#7982,.F.);
#11484=ORIENTED_EDGE('',*,*,#7985,.F.);
#11485=ORIENTED_EDGE('',*,*,#7988,.F.);
#11486=ORIENTED_EDGE('',*,*,#7991,.F.);
#11487=ORIENTED_EDGE('',*,*,#7994,.F.);
#11488=ORIENTED_EDGE('',*,*,#7997,.F.);
#11489=ORIENTED_EDGE('',*,*,#8000,.F.);
#11490=ORIENTED_EDGE('',*,*,#8003,.F.);
#11491=ORIENTED_EDGE('',*,*,#8006,.F.);
#11492=ORIENTED_EDGE('',*,*,#8009,.F.);
#11493=ORIENTED_EDGE('',*,*,#8012,.F.);
#11494=ORIENTED_EDGE('',*,*,#8015,.F.);
#11495=ORIENTED_EDGE('',*,*,#8018,.F.);
#11496=ORIENTED_EDGE('',*,*,#8021,.F.);
#11497=ORIENTED_EDGE('',*,*,#8024,.F.);
#11498=ORIENTED_EDGE('',*,*,#8030,.F.);
#11499=ORIENTED_EDGE('',*,*,#8029,.F.);
#11500=ORIENTED_EDGE('',*,*,#8033,.F.);
#11501=ORIENTED_EDGE('',*,*,#7938,.F.);
#11502=ORIENTED_EDGE('',*,*,#8034,.F.);
#11503=ORIENTED_EDGE('',*,*,#7936,.F.);
#11504=ORIENTED_EDGE('',*,*,#7933,.F.);
#11505=ORIENTED_EDGE('',*,*,#7930,.F.);
#11506=ORIENTED_EDGE('',*,*,#7927,.F.);
#11507=ORIENTED_EDGE('',*,*,#7924,.F.);
#11508=ORIENTED_EDGE('',*,*,#7921,.F.);
#11509=ORIENTED_EDGE('',*,*,#7918,.F.);
#11510=ORIENTED_EDGE('',*,*,#7915,.F.);
#11511=ORIENTED_EDGE('',*,*,#7912,.F.);
#11512=ORIENTED_EDGE('',*,*,#7909,.F.);
#11513=ORIENTED_EDGE('',*,*,#7906,.F.);
#11514=ORIENTED_EDGE('',*,*,#7903,.F.);
#11515=ORIENTED_EDGE('',*,*,#7900,.F.);
#11516=ORIENTED_EDGE('',*,*,#7897,.F.);
#11517=ORIENTED_EDGE('',*,*,#7894,.F.);
#11518=ORIENTED_EDGE('',*,*,#7891,.F.);
#11519=ORIENTED_EDGE('',*,*,#7888,.F.);
#11520=ORIENTED_EDGE('',*,*,#7885,.F.);
#11521=ORIENTED_EDGE('',*,*,#7882,.F.);
#11522=ORIENTED_EDGE('',*,*,#7879,.F.);
#11523=ORIENTED_EDGE('',*,*,#7876,.F.);
#11524=ORIENTED_EDGE('',*,*,#7873,.F.);
#11525=ORIENTED_EDGE('',*,*,#7870,.F.);
#11526=ORIENTED_EDGE('',*,*,#7867,.F.);
#11527=ORIENTED_EDGE('',*,*,#7864,.F.);
#11528=ORIENTED_EDGE('',*,*,#7861,.F.);
#11529=ORIENTED_EDGE('',*,*,#7858,.F.);
#11530=ORIENTED_EDGE('',*,*,#8035,.F.);
#11531=ORIENTED_EDGE('',*,*,#7856,.F.);
#11532=ORIENTED_EDGE('',*,*,#7860,.F.);
#11533=ORIENTED_EDGE('',*,*,#7863,.F.);
#11534=ORIENTED_EDGE('',*,*,#7866,.F.);
#11535=ORIENTED_EDGE('',*,*,#7869,.F.);
#11536=ORIENTED_EDGE('',*,*,#7872,.F.);
#11537=ORIENTED_EDGE('',*,*,#7875,.F.);
#11538=ORIENTED_EDGE('',*,*,#7878,.F.);
#11539=ORIENTED_EDGE('',*,*,#7881,.F.);
#11540=ORIENTED_EDGE('',*,*,#7884,.F.);
#11541=ORIENTED_EDGE('',*,*,#7887,.F.);
#11542=ORIENTED_EDGE('',*,*,#7890,.F.);
#11543=ORIENTED_EDGE('',*,*,#7893,.F.);
#11544=ORIENTED_EDGE('',*,*,#7896,.F.);
#11545=ORIENTED_EDGE('',*,*,#7899,.F.);
#11546=ORIENTED_EDGE('',*,*,#7902,.F.);
#11547=ORIENTED_EDGE('',*,*,#7905,.F.);
#11548=ORIENTED_EDGE('',*,*,#7908,.F.);
#11549=ORIENTED_EDGE('',*,*,#7911,.F.);
#11550=ORIENTED_EDGE('',*,*,#7914,.F.);
#11551=ORIENTED_EDGE('',*,*,#7917,.F.);
#11552=ORIENTED_EDGE('',*,*,#7920,.F.);
#11553=ORIENTED_EDGE('',*,*,#7923,.F.);
#11554=ORIENTED_EDGE('',*,*,#7926,.F.);
#11555=ORIENTED_EDGE('',*,*,#7929,.F.);
#11556=ORIENTED_EDGE('',*,*,#7932,.F.);
#11557=ORIENTED_EDGE('',*,*,#7935,.F.);
#11558=ORIENTED_EDGE('',*,*,#8036,.F.);
#11559=ORIENTED_EDGE('',*,*,#7940,.F.);
#11560=ORIENTED_EDGE('',*,*,#8037,.F.);
#11561=ORIENTED_EDGE('',*,*,#8027,.T.);
#11562=ORIENTED_EDGE('',*,*,#8031,.T.);
#11563=ORIENTED_EDGE('',*,*,#8025,.T.);
#11564=ORIENTED_EDGE('',*,*,#8022,.T.);
#11565=ORIENTED_EDGE('',*,*,#8019,.T.);
#11566=ORIENTED_EDGE('',*,*,#8016,.T.);
#11567=ORIENTED_EDGE('',*,*,#8013,.T.);
#11568=ORIENTED_EDGE('',*,*,#8010,.T.);
#11569=ORIENTED_EDGE('',*,*,#8007,.T.);
#11570=ORIENTED_EDGE('',*,*,#8004,.T.);
#11571=ORIENTED_EDGE('',*,*,#8001,.T.);
#11572=ORIENTED_EDGE('',*,*,#7998,.T.);
#11573=ORIENTED_EDGE('',*,*,#7995,.T.);
#11574=ORIENTED_EDGE('',*,*,#7992,.T.);
#11575=ORIENTED_EDGE('',*,*,#7989,.T.);
#11576=ORIENTED_EDGE('',*,*,#7986,.T.);
#11577=ORIENTED_EDGE('',*,*,#7983,.T.);
#11578=ORIENTED_EDGE('',*,*,#7980,.T.);
#11579=ORIENTED_EDGE('',*,*,#7977,.T.);
#11580=ORIENTED_EDGE('',*,*,#7974,.T.);
#11581=ORIENTED_EDGE('',*,*,#7971,.T.);
#11582=ORIENTED_EDGE('',*,*,#7968,.T.);
#11583=ORIENTED_EDGE('',*,*,#7965,.T.);
#11584=ORIENTED_EDGE('',*,*,#7962,.T.);
#11585=ORIENTED_EDGE('',*,*,#7959,.T.);
#11586=ORIENTED_EDGE('',*,*,#7956,.T.);
#11587=ORIENTED_EDGE('',*,*,#7953,.T.);
#11588=ORIENTED_EDGE('',*,*,#7950,.T.);
#11589=ORIENTED_EDGE('',*,*,#7947,.T.);
#11590=ORIENTED_EDGE('',*,*,#7944,.T.);
#11591=ORIENTED_EDGE('',*,*,#8038,.T.);
#11592=ORIENTED_EDGE('',*,*,#8039,.T.);
#11593=ORIENTED_EDGE('',*,*,#8040,.F.);
#11594=ORIENTED_EDGE('',*,*,#8041,.T.);
#11595=ORIENTED_EDGE('',*,*,#8042,.F.);
#11596=ORIENTED_EDGE('',*,*,#8043,.F.);
#11597=ORIENTED_EDGE('',*,*,#8044,.F.);
#11598=ORIENTED_EDGE('',*,*,#8045,.F.);
#11599=ORIENTED_EDGE('',*,*,#8033,.T.);
#11600=ORIENTED_EDGE('',*,*,#8028,.T.);
#11601=ORIENTED_EDGE('',*,*,#8037,.T.);
#11602=ORIENTED_EDGE('',*,*,#7939,.T.);
#11603=ORIENTED_EDGE('',*,*,#7937,.T.);
#11604=ORIENTED_EDGE('',*,*,#8036,.T.);
#11605=ORIENTED_EDGE('',*,*,#7934,.F.);
#11606=ORIENTED_EDGE('',*,*,#8034,.T.);
#11607=ORIENTED_EDGE('',*,*,#8046,.F.);
#11608=ORIENTED_EDGE('',*,*,#8047,.T.);
#11609=ORIENTED_EDGE('',*,*,#8048,.F.);
#11610=ORIENTED_EDGE('',*,*,#8049,.F.);
#11611=ORIENTED_EDGE('',*,*,#8050,.T.);
#11612=ORIENTED_EDGE('',*,*,#8051,.T.);
#11613=ORIENTED_EDGE('',*,*,#8048,.T.);
#11614=ORIENTED_EDGE('',*,*,#8052,.T.);
#11615=ORIENTED_EDGE('',*,*,#8046,.T.);
#11616=ORIENTED_EDGE('',*,*,#8053,.T.);
#11617=ORIENTED_EDGE('',*,*,#8042,.T.);
#11618=ORIENTED_EDGE('',*,*,#8054,.T.);
#11619=ORIENTED_EDGE('',*,*,#8055,.F.);
#11620=ORIENTED_EDGE('',*,*,#8056,.T.);
#11621=ORIENTED_EDGE('',*,*,#8052,.F.);
#11622=ORIENTED_EDGE('',*,*,#8047,.F.);
#11623=ORIENTED_EDGE('',*,*,#8054,.F.);
#11624=ORIENTED_EDGE('',*,*,#8041,.F.);
#11625=ORIENTED_EDGE('',*,*,#8057,.F.);
#11626=ORIENTED_EDGE('',*,*,#8043,.T.);
#11627=ORIENTED_EDGE('',*,*,#8053,.F.);
#11628=ORIENTED_EDGE('',*,*,#8049,.T.);
#11629=ORIENTED_EDGE('',*,*,#8051,.F.);
#11630=ORIENTED_EDGE('',*,*,#8058,.F.);
#11631=ORIENTED_EDGE('',*,*,#8055,.T.);
#11632=ORIENTED_EDGE('',*,*,#8040,.T.);
#11633=ORIENTED_EDGE('',*,*,#8059,.T.);
#11634=ORIENTED_EDGE('',*,*,#8060,.T.);
#11635=ORIENTED_EDGE('',*,*,#8057,.T.);
#11636=ORIENTED_EDGE('',*,*,#8061,.T.);
#11637=ORIENTED_EDGE('',*,*,#8062,.T.);
#11638=ORIENTED_EDGE('',*,*,#8044,.T.);
#11639=ORIENTED_EDGE('',*,*,#8063,.T.);
#11640=ORIENTED_EDGE('',*,*,#8064,.T.);
#11641=ORIENTED_EDGE('',*,*,#8059,.F.);
#11642=ORIENTED_EDGE('',*,*,#8039,.F.);
#11643=ORIENTED_EDGE('',*,*,#8065,.T.);
#11644=ORIENTED_EDGE('',*,*,#8045,.T.);
#11645=ORIENTED_EDGE('',*,*,#8062,.F.);
#11646=ORIENTED_EDGE('',*,*,#8066,.F.);
#11647=ORIENTED_EDGE('',*,*,#8067,.T.);
#11648=ORIENTED_EDGE('',*,*,#8066,.T.);
#11649=ORIENTED_EDGE('',*,*,#8061,.F.);
#11650=ORIENTED_EDGE('',*,*,#8058,.T.);
#11651=ORIENTED_EDGE('',*,*,#8050,.F.);
#11652=ORIENTED_EDGE('',*,*,#8056,.F.);
#11653=ORIENTED_EDGE('',*,*,#8060,.F.);
#11654=ORIENTED_EDGE('',*,*,#8064,.F.);
#11655=ORIENTED_EDGE('',*,*,#8032,.T.);
#11656=ORIENTED_EDGE('',*,*,#7857,.T.);
#11657=ORIENTED_EDGE('',*,*,#8035,.T.);
#11658=ORIENTED_EDGE('',*,*,#7943,.T.);
#11659=ORIENTED_EDGE('',*,*,#8067,.F.);
#11660=ORIENTED_EDGE('',*,*,#8063,.F.);
#11661=ORIENTED_EDGE('',*,*,#8038,.F.);
#11662=ORIENTED_EDGE('',*,*,#8065,.F.);
#13651=CYLINDRICAL_SURFACE('',#15371,5.13675);
#13652=CYLINDRICAL_SURFACE('',#15373,5.13675);
#13653=CYLINDRICAL_SURFACE('',#15374,5.13675);
#13654=CYLINDRICAL_SURFACE('',#15375,5.13675);
#13655=CYLINDRICAL_SURFACE('',#15376,5.13675);
#13656=CYLINDRICAL_SURFACE('',#15377,5.13675);
#13657=CYLINDRICAL_SURFACE('',#15378,5.13675);
#13658=CYLINDRICAL_SURFACE('',#15379,5.13675);
#13659=CYLINDRICAL_SURFACE('',#15380,5.13675);
#13660=CYLINDRICAL_SURFACE('',#15381,5.13675);
#13661=CYLINDRICAL_SURFACE('',#15382,5.13675);
#13662=CYLINDRICAL_SURFACE('',#15383,5.13675);
#13663=CYLINDRICAL_SURFACE('',#15384,5.13675);
#13664=CYLINDRICAL_SURFACE('',#15385,5.13675);
#13665=CYLINDRICAL_SURFACE('',#15386,5.13675);
#13666=CYLINDRICAL_SURFACE('',#15387,5.13675);
#13667=CYLINDRICAL_SURFACE('',#15388,5.13675);
#13668=CYLINDRICAL_SURFACE('',#15389,5.13675);
#13669=CYLINDRICAL_SURFACE('',#15390,5.13675);
#13670=CYLINDRICAL_SURFACE('',#15391,5.13675);
#13671=CYLINDRICAL_SURFACE('',#15392,5.13675);
#13672=CYLINDRICAL_SURFACE('',#15393,5.13675);
#13673=CYLINDRICAL_SURFACE('',#15394,5.13675);
#13674=CYLINDRICAL_SURFACE('',#15395,5.13675);
#13675=CYLINDRICAL_SURFACE('',#15396,5.13675);
#13676=CYLINDRICAL_SURFACE('',#15397,5.13675);
#13677=CYLINDRICAL_SURFACE('',#15398,5.13675);
#13678=CYLINDRICAL_SURFACE('',#15399,5.13675);
#13679=CYLINDRICAL_SURFACE('',#15401,6.11325);
#13680=CYLINDRICAL_SURFACE('',#15403,6.11325);
#13681=CYLINDRICAL_SURFACE('',#15404,6.11325);
#13682=CYLINDRICAL_SURFACE('',#15405,6.11325);
#13683=CYLINDRICAL_SURFACE('',#15406,6.11325);
#13684=CYLINDRICAL_SURFACE('',#15407,6.11325);
#13685=CYLINDRICAL_SURFACE('',#15408,6.11325);
#13686=CYLINDRICAL_SURFACE('',#15409,6.11325);
#13687=CYLINDRICAL_SURFACE('',#15410,6.11325);
#13688=CYLINDRICAL_SURFACE('',#15411,6.11325);
#13689=CYLINDRICAL_SURFACE('',#15412,6.11325);
#13690=CYLINDRICAL_SURFACE('',#15413,6.11325);
#13691=CYLINDRICAL_SURFACE('',#15414,6.11325);
#13692=CYLINDRICAL_SURFACE('',#15415,6.11325);
#13693=CYLINDRICAL_SURFACE('',#15416,6.11325);
#13694=CYLINDRICAL_SURFACE('',#15417,6.11325);
#13695=CYLINDRICAL_SURFACE('',#15418,6.11325);
#13696=CYLINDRICAL_SURFACE('',#15419,6.11325);
#13697=CYLINDRICAL_SURFACE('',#15420,6.11325);
#13698=CYLINDRICAL_SURFACE('',#15421,6.11325);
#13699=CYLINDRICAL_SURFACE('',#15422,6.11325);
#13700=CYLINDRICAL_SURFACE('',#15423,6.11325);
#13701=CYLINDRICAL_SURFACE('',#15424,6.11325);
#13702=CYLINDRICAL_SURFACE('',#15425,6.11325);
#13703=CYLINDRICAL_SURFACE('',#15426,6.11325);
#13704=CYLINDRICAL_SURFACE('',#15427,6.11325);
#13705=CYLINDRICAL_SURFACE('',#15428,6.11325);
#13706=CYLINDRICAL_SURFACE('',#15429,6.11325);
#13707=CYLINDRICAL_SURFACE('',#15430,6.11325);
#13708=CYLINDRICAL_SURFACE('',#15432,6.11325);
#13709=CYLINDRICAL_SURFACE('',#15434,5.13675);
#14349=ADVANCED_FACE('',(#921),#13651,.F.);
#14350=ADVANCED_FACE('',(#922),#13652,.F.);
#14351=ADVANCED_FACE('',(#923),#13653,.F.);
#14352=ADVANCED_FACE('',(#924),#13654,.F.);
#14353=ADVANCED_FACE('',(#925),#13655,.F.);
#14354=ADVANCED_FACE('',(#926),#13656,.F.);
#14355=ADVANCED_FACE('',(#927),#13657,.F.);
#14356=ADVANCED_FACE('',(#928),#13658,.F.);
#14357=ADVANCED_FACE('',(#929),#13659,.F.);
#14358=ADVANCED_FACE('',(#930),#13660,.F.);
#14359=ADVANCED_FACE('',(#931),#13661,.F.);
#14360=ADVANCED_FACE('',(#932),#13662,.F.);
#14361=ADVANCED_FACE('',(#933),#13663,.F.);
#14362=ADVANCED_FACE('',(#934),#13664,.F.);
#14363=ADVANCED_FACE('',(#935),#13665,.F.);
#14364=ADVANCED_FACE('',(#936),#13666,.F.);
#14365=ADVANCED_FACE('',(#937),#13667,.F.);
#14366=ADVANCED_FACE('',(#938),#13668,.F.);
#14367=ADVANCED_FACE('',(#939),#13669,.F.);
#14368=ADVANCED_FACE('',(#940),#13670,.F.);
#14369=ADVANCED_FACE('',(#941),#13671,.F.);
#14370=ADVANCED_FACE('',(#942),#13672,.F.);
#14371=ADVANCED_FACE('',(#943),#13673,.F.);
#14372=ADVANCED_FACE('',(#944),#13674,.F.);
#14373=ADVANCED_FACE('',(#945),#13675,.F.);
#14374=ADVANCED_FACE('',(#946),#13676,.F.);
#14375=ADVANCED_FACE('',(#947),#13677,.F.);
#14376=ADVANCED_FACE('',(#948),#13678,.F.);
#14377=ADVANCED_FACE('',(#949),#13679,.F.);
#14378=ADVANCED_FACE('',(#950),#13680,.F.);
#14379=ADVANCED_FACE('',(#951),#13681,.F.);
#14380=ADVANCED_FACE('',(#952),#13682,.F.);
#14381=ADVANCED_FACE('',(#953),#13683,.F.);
#14382=ADVANCED_FACE('',(#954),#13684,.F.);
#14383=ADVANCED_FACE('',(#955),#13685,.F.);
#14384=ADVANCED_FACE('',(#956),#13686,.F.);
#14385=ADVANCED_FACE('',(#957),#13687,.F.);
#14386=ADVANCED_FACE('',(#958),#13688,.F.);
#14387=ADVANCED_FACE('',(#959),#13689,.F.);
#14388=ADVANCED_FACE('',(#960),#13690,.F.);
#14389=ADVANCED_FACE('',(#961),#13691,.F.);
#14390=ADVANCED_FACE('',(#962),#13692,.F.);
#14391=ADVANCED_FACE('',(#963),#13693,.F.);
#14392=ADVANCED_FACE('',(#964),#13694,.F.);
#14393=ADVANCED_FACE('',(#965),#13695,.F.);
#14394=ADVANCED_FACE('',(#966),#13696,.F.);
#14395=ADVANCED_FACE('',(#967),#13697,.F.);
#14396=ADVANCED_FACE('',(#968),#13698,.F.);
#14397=ADVANCED_FACE('',(#969),#13699,.F.);
#14398=ADVANCED_FACE('',(#970),#13700,.F.);
#14399=ADVANCED_FACE('',(#971),#13701,.F.);
#14400=ADVANCED_FACE('',(#972),#13702,.F.);
#14401=ADVANCED_FACE('',(#973),#13703,.F.);
#14402=ADVANCED_FACE('',(#974),#13704,.F.);
#14403=ADVANCED_FACE('',(#975),#13705,.F.);
#14404=ADVANCED_FACE('',(#976),#13706,.F.);
#14405=ADVANCED_FACE('',(#977),#13707,.F.);
#14406=ADVANCED_FACE('',(#978),#13708,.F.);
#14407=ADVANCED_FACE('',(#979),#290,.F.);
#14408=ADVANCED_FACE('',(#980),#291,.F.);
#14409=ADVANCED_FACE('',(#981,#343),#450,.T.);
#14410=ADVANCED_FACE('',(#982),#13709,.F.);
#14411=ADVANCED_FACE('',(#983),#451,.T.);
#14412=ADVANCED_FACE('',(#984),#452,.T.);
#14413=ADVANCED_FACE('',(#985),#453,.T.);
#14414=ADVANCED_FACE('',(#986),#454,.T.);
#14415=ADVANCED_FACE('',(#987),#455,.T.);
#14416=ADVANCED_FACE('',(#988),#456,.T.);
#14417=ADVANCED_FACE('',(#989),#457,.T.);
#14418=ADVANCED_FACE('',(#990),#458,.T.);
#14419=ADVANCED_FACE('',(#991),#459,.T.);
#14420=ADVANCED_FACE('',(#992,#344),#460,.T.);
#14421=ADVANCED_FACE('',(#993),#461,.F.);
#14733=CLOSED_SHELL('',(#14349,#14350,#14351,#14352,#14353,#14354,#14355,
#14356,#14357,#14358,#14359,#14360,#14361,#14362,#14363,#14364,#14365,#14366,
#14367,#14368,#14369,#14370,#14371,#14372,#14373,#14374,#14375,#14376,#14377,
#14378,#14379,#14380,#14381,#14382,#14383,#14384,#14385,#14386,#14387,#14388,
#14389,#14390,#14391,#14392,#14393,#14394,#14395,#14396,#14397,#14398,#14399,
#14400,#14401,#14402,#14403,#14404,#14405,#14406,#14407,#14408,#14409,#14410,
#14411,#14412,#14413,#14414,#14415,#14416,#14417,#14418,#14419,#14420,#14421));
#15370=AXIS2_PLACEMENT_3D('',#43265,#17293,#17294);
#15371=AXIS2_PLACEMENT_3D('',#43266,#17295,#17296);
#15372=AXIS2_PLACEMENT_3D('',#43300,#17298,#17299);
#15373=AXIS2_PLACEMENT_3D('',#43341,#17300,#17301);
#15374=AXIS2_PLACEMENT_3D('',#43428,#17303,#17304);
#15375=AXIS2_PLACEMENT_3D('',#43515,#17306,#17307);
#15376=AXIS2_PLACEMENT_3D('',#43602,#17309,#17310);
#15377=AXIS2_PLACEMENT_3D('',#43692,#17312,#17313);
#15378=AXIS2_PLACEMENT_3D('',#43779,#17315,#17316);
#15379=AXIS2_PLACEMENT_3D('',#43866,#17318,#17319);
#15380=AXIS2_PLACEMENT_3D('',#43953,#17321,#17322);
#15381=AXIS2_PLACEMENT_3D('',#44040,#17324,#17325);
#15382=AXIS2_PLACEMENT_3D('',#44130,#17327,#17328);
#15383=AXIS2_PLACEMENT_3D('',#44217,#17330,#17331);
#15384=AXIS2_PLACEMENT_3D('',#44304,#17333,#17334);
#15385=AXIS2_PLACEMENT_3D('',#44391,#17336,#17337);
#15386=AXIS2_PLACEMENT_3D('',#44478,#17339,#17340);
#15387=AXIS2_PLACEMENT_3D('',#44565,#17342,#17343);
#15388=AXIS2_PLACEMENT_3D('',#44652,#17345,#17346);
#15389=AXIS2_PLACEMENT_3D('',#44739,#17348,#17349);
#15390=AXIS2_PLACEMENT_3D('',#44826,#17351,#17352);
#15391=AXIS2_PLACEMENT_3D('',#44913,#17354,#17355);
#15392=AXIS2_PLACEMENT_3D('',#45000,#17357,#17358);
#15393=AXIS2_PLACEMENT_3D('',#45090,#17360,#17361);
#15394=AXIS2_PLACEMENT_3D('',#45177,#17363,#17364);
#15395=AXIS2_PLACEMENT_3D('',#45264,#17366,#17367);
#15396=AXIS2_PLACEMENT_3D('',#45351,#17369,#17370);
#15397=AXIS2_PLACEMENT_3D('',#45438,#17372,#17373);
#15398=AXIS2_PLACEMENT_3D('',#45528,#17375,#17376);
#15399=AXIS2_PLACEMENT_3D('',#45615,#17378,#17379);
#15400=AXIS2_PLACEMENT_3D('',#45646,#17381,#17382);
#15401=AXIS2_PLACEMENT_3D('',#45684,#17383,#17384);
#15402=AXIS2_PLACEMENT_3D('',#45697,#17386,#17387);
#15403=AXIS2_PLACEMENT_3D('',#45706,#17388,#17389);
#15404=AXIS2_PLACEMENT_3D('',#45744,#17391,#17392);
#15405=AXIS2_PLACEMENT_3D('',#45780,#17394,#17395);
#15406=AXIS2_PLACEMENT_3D('',#45818,#17397,#17398);
#15407=AXIS2_PLACEMENT_3D('',#45855,#17400,#17401);
#15408=AXIS2_PLACEMENT_3D('',#45892,#17403,#17404);
#15409=AXIS2_PLACEMENT_3D('',#45930,#17406,#17407);
#15410=AXIS2_PLACEMENT_3D('',#45966,#17409,#17410);
#15411=AXIS2_PLACEMENT_3D('',#46004,#17412,#17413);
#15412=AXIS2_PLACEMENT_3D('',#46041,#17415,#17416);
#15413=AXIS2_PLACEMENT_3D('',#46078,#17418,#17419);
#15414=AXIS2_PLACEMENT_3D('',#46116,#17421,#17422);
#15415=AXIS2_PLACEMENT_3D('',#46152,#17424,#17425);
#15416=AXIS2_PLACEMENT_3D('',#46190,#17427,#17428);
#15417=AXIS2_PLACEMENT_3D('',#46227,#17430,#17431);
#15418=AXIS2_PLACEMENT_3D('',#46264,#17433,#17434);
#15419=AXIS2_PLACEMENT_3D('',#46302,#17436,#17437);
#15420=AXIS2_PLACEMENT_3D('',#46338,#17439,#17440);
#15421=AXIS2_PLACEMENT_3D('',#46376,#17442,#17443);
#15422=AXIS2_PLACEMENT_3D('',#46412,#17445,#17446);
#15423=AXIS2_PLACEMENT_3D('',#46450,#17448,#17449);
#15424=AXIS2_PLACEMENT_3D('',#46488,#17451,#17452);
#15425=AXIS2_PLACEMENT_3D('',#46524,#17454,#17455);
#15426=AXIS2_PLACEMENT_3D('',#46562,#17457,#17458);
#15427=AXIS2_PLACEMENT_3D('',#46598,#17460,#17461);
#15428=AXIS2_PLACEMENT_3D('',#46636,#17463,#17464);
#15429=AXIS2_PLACEMENT_3D('',#46674,#17466,#17467);
#15430=AXIS2_PLACEMENT_3D('',#46710,#17469,#17470);
#15431=AXIS2_PLACEMENT_3D('',#46722,#17472,#17473);
#15432=AXIS2_PLACEMENT_3D('',#46730,#17474,#17475);
#15433=AXIS2_PLACEMENT_3D('',#50232,#17476,#17477);
#15434=AXIS2_PLACEMENT_3D('',#50249,#17486,#17487);
#15435=AXIS2_PLACEMENT_3D('',#50250,#17488,#17489);
#15436=AXIS2_PLACEMENT_3D('',#50259,#17494,#17495);
#15437=AXIS2_PLACEMENT_3D('',#50265,#17499,#17500);
#15438=AXIS2_PLACEMENT_3D('',#50268,#17503,#17504);
#15439=AXIS2_PLACEMENT_3D('',#50272,#17507,#17508);
#15440=AXIS2_PLACEMENT_3D('',#50276,#17511,#17512);
#15441=AXIS2_PLACEMENT_3D('',#50280,#17515,#17516);
#15442=AXIS2_PLACEMENT_3D('',#50284,#17519,#17520);
#15443=AXIS2_PLACEMENT_3D('',#50288,#17523,#17524);
#15444=AXIS2_PLACEMENT_3D('',#50292,#17527,#17528);
#15445=AXIS2_PLACEMENT_3D('',#50294,#17530,#17531);
#17293=DIRECTION('axis',(0.,0.,1.));
#17294=DIRECTION('refdir',(1.,0.,0.));
#17295=DIRECTION('center_axis',(-1.,0.,0.));
#17296=DIRECTION('ref_axis',(0.,0.991178642906414,0.13253262936424));
#17297=DIRECTION('',(-1.,0.,0.));
#17298=DIRECTION('center_axis',(1.,0.,0.));
#17299=DIRECTION('ref_axis',(0.,1.,0.));
#17300=DIRECTION('center_axis',(-1.,0.,0.));
#17301=DIRECTION('ref_axis',(0.,1.,0.));
#17302=DIRECTION('',(-1.,0.,0.));
#17303=DIRECTION('center_axis',(-1.,0.,0.));
#17304=DIRECTION('ref_axis',(0.,1.,0.));
#17305=DIRECTION('',(-1.,0.,0.));
#17306=DIRECTION('center_axis',(-1.,0.,0.));
#17307=DIRECTION('ref_axis',(0.,1.,0.));
#17308=DIRECTION('',(-1.,0.,0.));
#17309=DIRECTION('center_axis',(-1.,0.,0.));
#17310=DIRECTION('ref_axis',(0.,1.,0.));
#17311=DIRECTION('',(-1.,0.,0.));
#17312=DIRECTION('center_axis',(-1.,0.,0.));
#17313=DIRECTION('ref_axis',(0.,1.,0.));
#17314=DIRECTION('',(-1.,0.,0.));
#17315=DIRECTION('center_axis',(-1.,0.,0.));
#17316=DIRECTION('ref_axis',(0.,1.,0.));
#17317=DIRECTION('',(-1.,0.,0.));
#17318=DIRECTION('center_axis',(-1.,0.,0.));
#17319=DIRECTION('ref_axis',(0.,1.,0.));
#17320=DIRECTION('',(-1.,0.,0.));
#17321=DIRECTION('center_axis',(-1.,0.,0.));
#17322=DIRECTION('ref_axis',(0.,1.,0.));
#17323=DIRECTION('',(-1.,0.,0.));
#17324=DIRECTION('center_axis',(-1.,0.,0.));
#17325=DIRECTION('ref_axis',(0.,1.,0.));
#17326=DIRECTION('',(-1.,0.,0.));
#17327=DIRECTION('center_axis',(-1.,0.,0.));
#17328=DIRECTION('ref_axis',(0.,1.,0.));
#17329=DIRECTION('',(-1.,0.,0.));
#17330=DIRECTION('center_axis',(-1.,0.,0.));
#17331=DIRECTION('ref_axis',(0.,1.,0.));
#17332=DIRECTION('',(-1.,0.,0.));
#17333=DIRECTION('center_axis',(-1.,0.,0.));
#17334=DIRECTION('ref_axis',(0.,1.,0.));
#17335=DIRECTION('',(-1.,0.,0.));
#17336=DIRECTION('center_axis',(-1.,0.,0.));
#17337=DIRECTION('ref_axis',(0.,1.,0.));
#17338=DIRECTION('',(-1.,0.,0.));
#17339=DIRECTION('center_axis',(-1.,0.,0.));
#17340=DIRECTION('ref_axis',(0.,1.,0.));
#17341=DIRECTION('',(-1.,0.,0.));
#17342=DIRECTION('center_axis',(-1.,0.,0.));
#17343=DIRECTION('ref_axis',(0.,1.,0.));
#17344=DIRECTION('',(-1.,0.,0.));
#17345=DIRECTION('center_axis',(-1.,0.,0.));
#17346=DIRECTION('ref_axis',(0.,1.,0.));
#17347=DIRECTION('',(-1.,0.,0.));
#17348=DIRECTION('center_axis',(-1.,0.,0.));
#17349=DIRECTION('ref_axis',(0.,1.,0.));
#17350=DIRECTION('',(-1.,0.,0.));
#17351=DIRECTION('center_axis',(-1.,0.,0.));
#17352=DIRECTION('ref_axis',(0.,1.,0.));
#17353=DIRECTION('',(-1.,0.,0.));
#17354=DIRECTION('center_axis',(-1.,0.,0.));
#17355=DIRECTION('ref_axis',(0.,1.,0.));
#17356=DIRECTION('',(-1.,0.,0.));
#17357=DIRECTION('center_axis',(-1.,0.,0.));
#17358=DIRECTION('ref_axis',(0.,1.,0.));
#17359=DIRECTION('',(-1.,0.,0.));
#17360=DIRECTION('center_axis',(-1.,0.,0.));
#17361=DIRECTION('ref_axis',(0.,1.,0.));
#17362=DIRECTION('',(-1.,0.,0.));
#17363=DIRECTION('center_axis',(-1.,0.,0.));
#17364=DIRECTION('ref_axis',(0.,1.,0.));
#17365=DIRECTION('',(-1.,0.,0.));
#17366=DIRECTION('center_axis',(-1.,0.,0.));
#17367=DIRECTION('ref_axis',(0.,1.,0.));
#17368=DIRECTION('',(-1.,0.,0.));
#17369=DIRECTION('center_axis',(-1.,0.,0.));
#17370=DIRECTION('ref_axis',(0.,1.,0.));
#17371=DIRECTION('',(-1.,0.,0.));
#17372=DIRECTION('center_axis',(-1.,0.,0.));
#17373=DIRECTION('ref_axis',(0.,1.,0.));
#17374=DIRECTION('',(-1.,0.,0.));
#17375=DIRECTION('center_axis',(-1.,0.,0.));
#17376=DIRECTION('ref_axis',(0.,1.,0.));
#17377=DIRECTION('',(-1.,0.,0.));
#17378=DIRECTION('center_axis',(-1.,0.,0.));
#17379=DIRECTION('ref_axis',(0.,0.936835173124404,-0.349771151464737));
#17380=DIRECTION('',(-1.,0.,0.));
#17381=DIRECTION('center_axis',(-1.,0.,0.));
#17382=DIRECTION('ref_axis',(0.,1.,0.));
#17383=DIRECTION('center_axis',(-1.,0.,0.));
#17384=DIRECTION('ref_axis',(0.,-0.417222372432346,0.908804429974857));
#17385=DIRECTION('',(-1.,1.22464679914735E-16,1.19060305846873E-29));
#17386=DIRECTION('center_axis',(1.,0.,0.));
#17387=DIRECTION('ref_axis',(0.,1.,9.73425822924114E-14));
#17388=DIRECTION('center_axis',(-1.,0.,0.));
#17389=DIRECTION('ref_axis',(0.,1.,9.73425822924114E-14));
#17390=DIRECTION('',(-1.,1.22464679914735E-16,1.19060305846873E-29));
#17391=DIRECTION('center_axis',(-1.,0.,0.));
#17392=DIRECTION('ref_axis',(0.,1.,9.73425822924114E-14));
#17393=DIRECTION('',(-1.,1.22464679914735E-16,1.19060305846873E-29));
#17394=DIRECTION('center_axis',(-1.,0.,0.));
#17395=DIRECTION('ref_axis',(0.,1.,9.73425822924114E-14));
#17396=DIRECTION('',(-1.,1.22464679914735E-16,1.19060305846873E-29));
#17397=DIRECTION('center_axis',(-1.,0.,0.));
#17398=DIRECTION('ref_axis',(0.,1.,9.73425822924114E-14));
#17399=DIRECTION('',(-1.,1.22464679914735E-16,1.19060305846873E-29));
#17400=DIRECTION('center_axis',(-1.,0.,0.));
#17401=DIRECTION('ref_axis',(0.,1.,9.73425822924114E-14));
#17402=DIRECTION('',(-1.,1.22464679914735E-16,1.19060305846873E-29));
#17403=DIRECTION('center_axis',(-1.,0.,0.));
#17404=DIRECTION('ref_axis',(0.,1.,9.73425822924114E-14));
#17405=DIRECTION('',(-1.,1.22464679914735E-16,1.19060305846873E-29));
#17406=DIRECTION('center_axis',(-1.,0.,0.));
#17407=DIRECTION('ref_axis',(0.,1.,9.73425822924114E-14));
#17408=DIRECTION('',(-1.,1.22464679914735E-16,1.19060305846873E-29));
#17409=DIRECTION('center_axis',(-1.,0.,0.));
#17410=DIRECTION('ref_axis',(0.,1.,9.73425822924114E-14));
#17411=DIRECTION('',(-1.,1.22464679914735E-16,1.19060305846873E-29));
#17412=DIRECTION('center_axis',(-1.,0.,0.));
#17413=DIRECTION('ref_axis',(0.,1.,9.73425822924114E-14));
#17414=DIRECTION('',(-1.,1.22464679914735E-16,1.19060305846873E-29));
#17415=DIRECTION('center_axis',(-1.,0.,0.));
#17416=DIRECTION('ref_axis',(0.,1.,9.73425822924114E-14));
#17417=DIRECTION('',(-1.,1.22464679914735E-16,1.19060305846873E-29));
#17418=DIRECTION('center_axis',(-1.,0.,0.));
#17419=DIRECTION('ref_axis',(0.,1.,9.73425822924114E-14));
#17420=DIRECTION('',(-1.,1.22464679914735E-16,1.19060305846873E-29));
#17421=DIRECTION('center_axis',(-1.,0.,0.));
#17422=DIRECTION('ref_axis',(0.,1.,9.73425822924114E-14));
#17423=DIRECTION('',(-1.,1.22464679914735E-16,1.19060305846873E-29));
#17424=DIRECTION('center_axis',(-1.,0.,0.));
#17425=DIRECTION('ref_axis',(0.,1.,9.73425822924114E-14));
#17426=DIRECTION('',(-1.,1.22464679914735E-16,1.19060305846873E-29));
#17427=DIRECTION('center_axis',(-1.,0.,0.));
#17428=DIRECTION('ref_axis',(0.,1.,9.73425822924114E-14));
#17429=DIRECTION('',(-1.,1.22464679914735E-16,1.19060305846873E-29));
#17430=DIRECTION('center_axis',(-1.,0.,0.));
#17431=DIRECTION('ref_axis',(0.,1.,9.73425822924114E-14));
#17432=DIRECTION('',(-1.,1.22464679914735E-16,1.19060305846873E-29));
#17433=DIRECTION('center_axis',(-1.,0.,0.));
#17434=DIRECTION('ref_axis',(0.,1.,9.73425822924114E-14));
#17435=DIRECTION('',(-1.,1.22464679914735E-16,1.19060305846873E-29));
#17436=DIRECTION('center_axis',(-1.,0.,0.));
#17437=DIRECTION('ref_axis',(0.,1.,9.73425822924114E-14));
#17438=DIRECTION('',(-1.,1.22464679914735E-16,1.19060305846873E-29));
#17439=DIRECTION('center_axis',(-1.,0.,0.));
#17440=DIRECTION('ref_axis',(0.,1.,9.73425822924114E-14));
#17441=DIRECTION('',(-1.,1.22464679914735E-16,1.19060305846873E-29));
#17442=DIRECTION('center_axis',(-1.,0.,0.));
#17443=DIRECTION('ref_axis',(0.,1.,9.73425822924114E-14));
#17444=DIRECTION('',(-1.,1.22464679914735E-16,1.19060305846873E-29));
#17445=DIRECTION('center_axis',(-1.,0.,0.));
#17446=DIRECTION('ref_axis',(0.,1.,9.73425822924114E-14));
#17447=DIRECTION('',(-1.,1.22464679914735E-16,1.19060305846873E-29));
#17448=DIRECTION('center_axis',(-1.,0.,0.));
#17449=DIRECTION('ref_axis',(0.,1.,9.73425822924114E-14));
#17450=DIRECTION('',(-1.,1.22464679914735E-16,1.19060305846873E-29));
#17451=DIRECTION('center_axis',(-1.,0.,0.));
#17452=DIRECTION('ref_axis',(0.,1.,9.73425822924114E-14));
#17453=DIRECTION('',(-1.,1.22464679914735E-16,1.19060305846873E-29));
#17454=DIRECTION('center_axis',(-1.,0.,0.));
#17455=DIRECTION('ref_axis',(0.,1.,9.73425822924114E-14));
#17456=DIRECTION('',(-1.,1.22464679914735E-16,1.19060305846873E-29));
#17457=DIRECTION('center_axis',(-1.,0.,0.));
#17458=DIRECTION('ref_axis',(0.,1.,9.73425822924114E-14));
#17459=DIRECTION('',(-1.,1.22464679914735E-16,1.19060305846873E-29));
#17460=DIRECTION('center_axis',(-1.,0.,0.));
#17461=DIRECTION('ref_axis',(0.,1.,9.73425822924114E-14));
#17462=DIRECTION('',(-1.,1.22464679914735E-16,1.19060305846873E-29));
#17463=DIRECTION('center_axis',(-1.,0.,0.));
#17464=DIRECTION('ref_axis',(0.,1.,9.73425822924114E-14));
#17465=DIRECTION('',(-1.,1.22464679914735E-16,1.19060305846873E-29));
#17466=DIRECTION('center_axis',(-1.,0.,0.));
#17467=DIRECTION('ref_axis',(0.,1.,9.73425822924114E-14));
#17468=DIRECTION('',(-1.,1.22464679914735E-16,1.19060305846873E-29));
#17469=DIRECTION('center_axis',(-1.,0.,0.));
#17470=DIRECTION('ref_axis',(0.,-0.608992615770512,-0.79317589092016));
#17471=DIRECTION('',(-1.,1.22464679914735E-16,1.19060305846873E-29));
#17472=DIRECTION('center_axis',(-1.,0.,0.));
#17473=DIRECTION('ref_axis',(0.,1.,9.73425822924114E-14));
#17474=DIRECTION('center_axis',(-1.,0.,0.));
#17475=DIRECTION('ref_axis',(0.,1.,9.73425822924114E-14));
#17476=DIRECTION('center_axis',(1.,0.,0.));
#17477=DIRECTION('ref_axis',(0.,1.,0.));
#17478=DIRECTION('',(0.,1.,0.));
#17479=DIRECTION('',(0.,0.,1.));
#17480=DIRECTION('',(0.,1.,0.));
#17481=DIRECTION('',(0.,0.,1.));
#17482=DIRECTION('',(0.,1.,0.));
#17483=DIRECTION('',(0.,0.,1.));
#17484=DIRECTION('',(0.,1.,0.));
#17485=DIRECTION('',(0.,0.,1.));
#17486=DIRECTION('center_axis',(-1.,0.,0.));
#17487=DIRECTION('ref_axis',(0.,1.,0.));
#17488=DIRECTION('center_axis',(1.,0.,0.));
#17489=DIRECTION('ref_axis',(0.,1.,0.));
#17490=DIRECTION('',(0.,-1.,0.));
#17491=DIRECTION('',(0.,0.,1.));
#17492=DIRECTION('',(0.,1.,0.));
#17493=DIRECTION('',(0.,0.,1.));
#17494=DIRECTION('center_axis',(0.,0.,1.));
#17495=DIRECTION('ref_axis',(1.,0.,0.));
#17496=DIRECTION('',(0.,-1.,0.));
#17497=DIRECTION('',(1.,0.,0.));
#17498=DIRECTION('',(-1.,0.,0.));
#17499=DIRECTION('center_axis',(0.,0.,1.));
#17500=DIRECTION('ref_axis',(1.,0.,0.));
#17501=DIRECTION('',(1.,0.,0.));
#17502=DIRECTION('',(-1.,0.,0.));
#17503=DIRECTION('center_axis',(0.,1.,0.));
#17504=DIRECTION('ref_axis',(-1.,0.,0.));
#17505=DIRECTION('',(1.,0.,0.));
#17506=DIRECTION('',(0.,0.,1.));
#17507=DIRECTION('center_axis',(0.,-1.,0.));
#17508=DIRECTION('ref_axis',(1.,0.,0.));
#17509=DIRECTION('',(-1.,0.,0.));
#17510=DIRECTION('',(0.,0.,1.));
#17511=DIRECTION('center_axis',(0.,0.,1.));
#17512=DIRECTION('ref_axis',(1.,0.,0.));
#17513=DIRECTION('',(-1.,0.,0.));
#17514=DIRECTION('',(0.,-1.,0.));
#17515=DIRECTION('center_axis',(0.,0.,1.));
#17516=DIRECTION('ref_axis',(1.,0.,0.));
#17517=DIRECTION('',(0.,-1.,0.));
#17518=DIRECTION('',(1.,0.,0.));
#17519=DIRECTION('center_axis',(0.,1.,0.));
#17520=DIRECTION('ref_axis',(-1.,0.,0.));
#17521=DIRECTION('',(-1.,0.,0.));
#17522=DIRECTION('',(0.,0.,1.));
#17523=DIRECTION('center_axis',(0.,-1.,0.));
#17524=DIRECTION('ref_axis',(1.,0.,0.));
#17525=DIRECTION('',(1.,0.,0.));
#17526=DIRECTION('',(0.,0.,1.));
#17527=DIRECTION('center_axis',(-1.,0.,0.));
#17528=DIRECTION('ref_axis',(0.,-1.,0.));
#17529=DIRECTION('',(0.,-1.,0.));
#17530=DIRECTION('center_axis',(0.,0.,1.));
#17531=DIRECTION('ref_axis',(1.,0.,0.));
#43265=CARTESIAN_POINT('',(0.,0.,0.));
#43266=CARTESIAN_POINT('Origin',(25.,0.,20.));
#43267=CARTESIAN_POINT('',(1.67595849469688,-5.1370281214151,20.0000980417081));
#43268=CARTESIAN_POINT('',(1.19904150530312,-5.13642988889554,19.9999056069319));
#43269=CARTESIAN_POINT('',(25.,-5.13675,20.));
#43270=CARTESIAN_POINT('',(0.,2.03511426366965,15.2835913560943));
#43271=CARTESIAN_POINT('Ctrl Pts',(1.19904150530312,-5.13642988889554,19.9999056069319));
#43272=CARTESIAN_POINT('Ctrl Pts',(1.16979164483845,-5.13607337989701,20.5394453457191));
#43273=CARTESIAN_POINT('Ctrl Pts',(1.14054178437377,-5.05144972646588,21.0790942532312));
#43274=CARTESIAN_POINT('Ctrl Pts',(1.1112919239091,-4.88433464596569,21.591857523604));
#43275=CARTESIAN_POINT('Ctrl Pts',(1.06498809374622,-4.61978404017791,22.4035845885512));
#43276=CARTESIAN_POINT('Ctrl Pts',(1.01868426358334,-4.14850745767332,23.147935444906));
#43277=CARTESIAN_POINT('Ctrl Pts',(0.972380433420454,-3.5279135019224,23.7342406241061));
#43278=CARTESIAN_POINT('Ctrl Pts',(0.926076603257575,-2.90731954617152,
24.3205458033061));
#43279=CARTESIAN_POINT('Ctrl Pts',(0.879772773094695,-2.13740821717434,
24.7488053053514));
#43280=CARTESIAN_POINT('Ctrl Pts',(0.833468942931815,-1.31196997330618,
24.9668393096929));
#43281=CARTESIAN_POINT('Ctrl Pts',(0.787165112768935,-0.486531729438019,
25.1848733140344));
#43282=CARTESIAN_POINT('Ctrl Pts',(0.740861282606054,0.394433429301118,
25.1926818206721));
#43283=CARTESIAN_POINT('Ctrl Pts',(0.694557452443174,1.22361266905245,24.9893341571924));
#43284=CARTESIAN_POINT('Ctrl Pts',(0.648253622280297,2.05279190880373,24.7859864937127));
#43285=CARTESIAN_POINT('Ctrl Pts',(0.60194979211742,2.83018522956722,24.3714826601157));
#43286=CARTESIAN_POINT('Ctrl Pts',(0.555645961954543,3.4610850284195,23.7962758976919));
#43287=CARTESIAN_POINT('Ctrl Pts',(0.509342131791666,4.09198482727179,23.2210691352681));
#43288=CARTESIAN_POINT('Ctrl Pts',(0.463038301628789,4.57639110421287,22.4851594440176));
#43289=CARTESIAN_POINT('Ctrl Pts',(0.416734471465911,4.85530994747718,21.6782733986309));
#43290=CARTESIAN_POINT('Ctrl Pts',(0.370430641303029,5.13422879074152,20.8713873532441));
#43291=CARTESIAN_POINT('Ctrl Pts',(0.324126811140146,5.20766020032903,19.993524953721));
#43292=CARTESIAN_POINT('Ctrl Pts',(0.277822980977266,5.06662947414752,19.1514626743736));
#43293=CARTESIAN_POINT('Ctrl Pts',(0.23151915081439,4.92559874796603,18.3094003950264));
#43294=CARTESIAN_POINT('Ctrl Pts',(0.185215320651517,4.57010588601557,17.5031382358548));
#43295=CARTESIAN_POINT('Ctrl Pts',(0.138911490488641,4.04350918221108,16.8312698444277));
#43296=CARTESIAN_POINT('Ctrl Pts',(0.0926076603257671,3.51691247840663,
16.1594014530006));
#43297=CARTESIAN_POINT('Ctrl Pts',(0.0463038301628913,2.81921193274818,
15.621926829318));
#43298=CARTESIAN_POINT('Ctrl Pts',(1.67921232474555E-14,2.03511426366992,
15.2835913560944));
#43299=CARTESIAN_POINT('',(8.67361737988404E-17,-4.95671627827806,18.6504206457069));
#43300=CARTESIAN_POINT('Origin',(0.,0.,20.));
#43301=CARTESIAN_POINT('Ctrl Pts',(8.67361737988404E-17,-4.95671627827806,
18.6504206457069));
#43302=CARTESIAN_POINT('Ctrl Pts',(0.0435916381931696,-4.74515587227111,
17.8749982094656));
#43303=CARTESIAN_POINT('Ctrl Pts',(0.087183276386337,-4.34884798055575,
17.1496924532122));
#43304=CARTESIAN_POINT('Ctrl Pts',(0.130774914579507,-3.80964413227746,
16.5536547957343));
#43305=CARTESIAN_POINT('Ctrl Pts',(0.177078744742386,-3.23689200712882,
15.9205327657653));
#43306=CARTESIAN_POINT('Ctrl Pts',(0.223382574905267,-2.50290931084975,
15.4332648935754));
#43307=CARTESIAN_POINT('Ctrl Pts',(0.269686405068148,-1.69709307475199,
15.1512235477709));
#43308=CARTESIAN_POINT('Ctrl Pts',(0.315990235231029,-0.891276838654234,
14.8691822019664));
#43309=CARTESIAN_POINT('Ctrl Pts',(0.362294065393908,-0.0136270627378211,
14.7923673825474));
#43310=CARTESIAN_POINT('Ctrl Pts',(0.408597895556788,0.828935910813523,
14.9301289758831));
#43311=CARTESIAN_POINT('Ctrl Pts',(0.454901725719665,1.67149888436482,15.0678905692187));
#43312=CARTESIAN_POINT('Ctrl Pts',(0.501205555882542,2.47897505555102,15.4202285753089));
#43313=CARTESIAN_POINT('Ctrl Pts',(0.54750938604542,3.15300369865065,15.944225949857));
#43314=CARTESIAN_POINT('Ctrl Pts',(0.593813216208297,3.82703234175028,16.4682233244052));
#43315=CARTESIAN_POINT('Ctrl Pts',(0.640117046371173,4.36761345676332,17.1638800674114));
#43316=CARTESIAN_POINT('Ctrl Pts',(0.686420876534051,4.70889301949145,17.9464512664084));
#43317=CARTESIAN_POINT('Ctrl Pts',(0.732724706696928,5.05017258221958,18.7290224654053));
#43318=CARTESIAN_POINT('Ctrl Pts',(0.779028536859813,5.19215059266281,19.5985081203932));
#43319=CARTESIAN_POINT('Ctrl Pts',(0.825332367022691,5.11753265898529,20.448990868539));
#43320=CARTESIAN_POINT('Ctrl Pts',(0.871636197185571,5.04291472530777,21.2994736166849));
#43321=CARTESIAN_POINT('Ctrl Pts',(0.917940027348451,4.75170084750951,22.1309534579889));
#43322=CARTESIAN_POINT('Ctrl Pts',(0.964243857511331,4.27936539996342,22.8421413166637));
#43323=CARTESIAN_POINT('Ctrl Pts',(1.01054768767421,3.80702995241733,23.5533291753386));
#43324=CARTESIAN_POINT('Ctrl Pts',(1.05685151783709,3.15357293512343,24.1442250513843));
#43325=CARTESIAN_POINT('Ctrl Pts',(1.10315534799997,2.3985969297664,24.5428478929248));
#43326=CARTESIAN_POINT('Ctrl Pts',(1.14945917816285,1.64362092440936,24.9414707344653));
#43327=CARTESIAN_POINT('Ctrl Pts',(1.19576300832573,0.787125930989224,25.1478205415004));
#43328=CARTESIAN_POINT('Ctrl Pts',(1.24206683848861,-0.0665523229436308,
25.1367602221083));
#43329=CARTESIAN_POINT('Ctrl Pts',(1.28837066865149,-0.920230576876437,
25.1256999027162));
#43330=CARTESIAN_POINT('Ctrl Pts',(1.33467449881437,-1.77109209132193,24.8972294568967));
#43331=CARTESIAN_POINT('Ctrl Pts',(1.38097832897724,-2.51548720074908,24.4791805886385));
#43332=CARTESIAN_POINT('Ctrl Pts',(1.42728215914012,-3.25988231017623,24.0611317203803));
#43333=CARTESIAN_POINT('Ctrl Pts',(1.473585989303,-3.89781101458502,23.4535044296833));
#43334=CARTESIAN_POINT('Ctrl Pts',(1.51988981946587,-4.35156263339055,22.7303181625132));
#43335=CARTESIAN_POINT('Ctrl Pts',(1.56619364962876,-4.80531425219613,22.007131895343));
#43336=CARTESIAN_POINT('Ctrl Pts',(1.61249747979164,-5.07488878539839,21.1683866516996));
#43337=CARTESIAN_POINT('Ctrl Pts',(1.65880130995452,-5.12744739087817,20.316256078288));
#43338=CARTESIAN_POINT('Ctrl Pts',(1.66452037153531,-5.13393898995932,20.2110080414178));
#43339=CARTESIAN_POINT('Ctrl Pts',(1.6702394331161,-5.13711998437662,20.1055558096961));
#43340=CARTESIAN_POINT('Ctrl Pts',(1.67595849469688,-5.1370281214151,20.0000980417081));
#43341=CARTESIAN_POINT('Origin',(25.,0.,20.));
#43342=CARTESIAN_POINT('',(3.42595849469688,-5.13662475218558,19.9998702837641));
#43343=CARTESIAN_POINT('',(2.94904150530311,-5.13675306620054,20.0001330755183));
#43344=CARTESIAN_POINT('',(25.,-5.13675,20.));
#43345=CARTESIAN_POINT('Ctrl Pts',(2.94904150530311,-5.13675306620054,20.0001330755183));
#43346=CARTESIAN_POINT('Ctrl Pts',(2.93840810362253,-5.1369545100676,20.1962400809989));
#43347=CARTESIAN_POINT('Ctrl Pts',(2.92777470194195,-5.12593941290559,20.3923245889008));
#43348=CARTESIAN_POINT('Ctrl Pts',(2.91714130026136,-5.10353305157791,20.5870986720596));
#43349=CARTESIAN_POINT('Ctrl Pts',(2.87083747009849,-5.00596311294013,21.4352549194799));
#43350=CARTESIAN_POINT('Ctrl Pts',(2.82453363993561,-4.69238941147243,22.2585625924748));
#43351=CARTESIAN_POINT('Ctrl Pts',(2.77822980977273,-4.2010106299116,22.956728622548));
#43352=CARTESIAN_POINT('Ctrl Pts',(2.73192597960986,-3.70963184835079,23.6548946526213));
#43353=CARTESIAN_POINT('Ctrl Pts',(2.68562214944698,-3.0404479866969,24.2279190397728));
#43354=CARTESIAN_POINT('Ctrl Pts',(2.6393183192841,-2.27497717516906,24.6059975367511));
#43355=CARTESIAN_POINT('Ctrl Pts',(2.59301448912122,-1.50950636364119,24.9840760337294));
#43356=CARTESIAN_POINT('Ctrl Pts',(2.54671065895834,-0.647748602239379,
25.1672086405343));
#43357=CARTESIAN_POINT('Ctrl Pts',(2.50040682879546,0.205319157132801,25.1330866455296));
#43358=CARTESIAN_POINT('Ctrl Pts',(2.45410299863258,1.05838691650498,25.0989646505249));
#43359=CARTESIAN_POINT('Ctrl Pts',(2.4077991684697,1.9027646738475,24.8475880537104));
#43360=CARTESIAN_POINT('Ctrl Pts',(2.36149533830682,2.6355926631063,24.4095788641542));
#43361=CARTESIAN_POINT('Ctrl Pts',(2.31519150814394,3.36842065236505,23.971569674598));
#43362=CARTESIAN_POINT('Ctrl Pts',(2.26888767798107,3.98969887354006,23.3469278923001));
#43363=CARTESIAN_POINT('Ctrl Pts',(2.22258384781819,4.42374492670835,22.6117456427229));
#43364=CARTESIAN_POINT('Ctrl Pts',(2.17628001765531,4.85779097987664,21.8765633931457));
#43365=CARTESIAN_POINT('Ctrl Pts',(2.12997618749244,5.10460486503819,21.0308406762892));
#43366=CARTESIAN_POINT('Ctrl Pts',(2.08367235732956,5.13412040058503,20.1776011220843));
#43367=CARTESIAN_POINT('Ctrl Pts',(2.03736852716668,5.16363593613188,19.3243615678793));
#43368=CARTESIAN_POINT('Ctrl Pts',(1.99106469700379,4.97585312206397,18.4636051763258));
#43369=CARTESIAN_POINT('Ctrl Pts',(1.94476086684092,4.593647133555,17.7001868684259));
#43370=CARTESIAN_POINT('Ctrl Pts',(1.89845703667804,4.21144114504601,16.936768560526));
#43371=CARTESIAN_POINT('Ctrl Pts',(1.85215320651516,3.63481198209594,16.2706883362796));
#43372=CARTESIAN_POINT('Ctrl Pts',(1.80584937635228,2.93400303467477,15.7830863406323));
#43373=CARTESIAN_POINT('Ctrl Pts',(1.75954554618939,2.23319408725357,15.2954843449849));
#43374=CARTESIAN_POINT('Ctrl Pts',(1.71324171602651,1.40820535536131,14.9863605779366));
#43375=CARTESIAN_POINT('Ctrl Pts',(1.66693788586363,0.559534654553702,14.8933714642486));
#43376=CARTESIAN_POINT('Ctrl Pts',(1.62063405570075,-0.289136046253805,
14.8003823505606));
#43377=CARTESIAN_POINT('Ctrl Pts',(1.57433022553787,-1.16148871597661,14.9235278902329));
#43378=CARTESIAN_POINT('Ctrl Pts',(1.528026395375,-1.95125569367861,15.2478071862158));
#43379=CARTESIAN_POINT('Ctrl Pts',(1.48172256521212,-2.74102267138062,15.5720864821987));
#43380=CARTESIAN_POINT('Ctrl Pts',(1.43541873504924,-3.4482039570618,16.0974995344921));
#43381=CARTESIAN_POINT('Ctrl Pts',(1.38911490488637,-3.98665281109446,16.7600412814375));
#43382=CARTESIAN_POINT('Ctrl Pts',(1.34281107472349,-4.52510166512713,17.422583028383));
#43383=CARTESIAN_POINT('Ctrl Pts',(1.29650724456061,-4.89481808751126,18.2222534699804));
#43384=CARTESIAN_POINT('Ctrl Pts',(1.25020341439773,-5.05076398416784,19.0616403275488));
#43385=CARTESIAN_POINT('Ctrl Pts',(1.23314944469953,-5.10819976403283,19.3707913844634));
#43386=CARTESIAN_POINT('Ctrl Pts',(1.21609547500132,-5.13663774949937,19.6853299402422));
#43387=CARTESIAN_POINT('Ctrl Pts',(1.19904150530312,-5.13642988889554,19.9999056069319));
#43388=CARTESIAN_POINT('Ctrl Pts',(1.67595849469688,-5.1370281214151,20.0000980417081));
#43389=CARTESIAN_POINT('Ctrl Pts',(1.71654326327897,-5.13637622477403,19.25172716853));
#43390=CARTESIAN_POINT('Ctrl Pts',(1.75712803186106,-4.9709066914377,18.5030774948426));
#43391=CARTESIAN_POINT('Ctrl Pts',(1.79771280044315,-4.65410916960248,17.8251431180106));
#43392=CARTESIAN_POINT('Ctrl Pts',(1.84401663060603,-4.29266966508966,17.0516766343244));
#43393=CARTESIAN_POINT('Ctrl Pts',(1.89032046076891,-3.73424797830663,16.3702595701316));
#43394=CARTESIAN_POINT('Ctrl Pts',(1.93662429093179,-3.04686949311008,15.8639002752298));
#43395=CARTESIAN_POINT('Ctrl Pts',(1.98292812109466,-2.35949100791349,15.3575409803279));
#43396=CARTESIAN_POINT('Ctrl Pts',(2.02923195125755,-1.54315572430333,15.026239454717));
#43397=CARTESIAN_POINT('Ctrl Pts',(2.07553578142043,-0.697307354947416,
14.9103539333822));
#43398=CARTESIAN_POINT('Ctrl Pts',(2.12183961158331,0.148541014408493,14.7944684120474));
#43399=CARTESIAN_POINT('Ctrl Pts',(2.16814344174618,1.02390246951018,14.8939988949887));
#43400=CARTESIAN_POINT('Ctrl Pts',(2.21444727190906,1.82214289574261,15.1968208546759));
#43401=CARTESIAN_POINT('Ctrl Pts',(2.26075110207194,2.62038332197499,15.4996428143631));
#43402=CARTESIAN_POINT('Ctrl Pts',(2.30705493223482,3.34150271933815,16.0057562507961));
#43403=CARTESIAN_POINT('Ctrl Pts',(2.3533587623977,3.89765631317662,16.6535078218819));
#43404=CARTESIAN_POINT('Ctrl Pts',(2.39966259256058,4.45380990701512,17.3012593929677));
#43405=CARTESIAN_POINT('Ctrl Pts',(2.44596642272346,4.84499769732893,18.0906490987062));
#43406=CARTESIAN_POINT('Ctrl Pts',(2.49227025288633,5.02356626779578,18.9255156648107));
#43407=CARTESIAN_POINT('Ctrl Pts',(2.53857408304922,5.20213483826264,19.7603822309153));
#43408=CARTESIAN_POINT('Ctrl Pts',(2.58487791321209,5.16808418888255,20.6407256573858));
#43409=CARTESIAN_POINT('Ctrl Pts',(2.63118174337498,4.92556227560906,21.459304938352));
#43410=CARTESIAN_POINT('Ctrl Pts',(2.67748557353785,4.68304036233561,22.2778842193182));
#43411=CARTESIAN_POINT('Ctrl Pts',(2.72378940370073,4.23204718516878,23.0346993547799));
#43412=CARTESIAN_POINT('Ctrl Pts',(2.77009323386361,3.62752148790459,23.6375572144555));
#43413=CARTESIAN_POINT('Ctrl Pts',(2.81639706402649,3.0229957906404,24.240415074131));
#43414=CARTESIAN_POINT('Ctrl Pts',(2.86270089418936,2.26493757327881,24.6893156580203));
#43415=CARTESIAN_POINT('Ctrl Pts',(2.90900472435224,1.44569139494332,24.9295751362994));
#43416=CARTESIAN_POINT('Ctrl Pts',(2.95530855451512,0.626445216607834,25.1698346145785));
#43417=CARTESIAN_POINT('Ctrl Pts',(3.001612384678,-0.253988922701738,25.2014529872475));
#43418=CARTESIAN_POINT('Ctrl Pts',(3.04791621484087,-1.08835896685382,25.0205785914601));
#43419=CARTESIAN_POINT('Ctrl Pts',(3.09422004500375,-1.92272901100601,24.8397041956727));
#43420=CARTESIAN_POINT('Ctrl Pts',(3.14052387516663,-2.71103496000072,24.4463370314289));
#43421=CARTESIAN_POINT('Ctrl Pts',(3.18682770532951,-3.35724755952852,23.8883960006432));
#43422=CARTESIAN_POINT('Ctrl Pts',(3.23313153549239,-4.00346015905632,23.3304549698574));
#43423=CARTESIAN_POINT('Ctrl Pts',(3.27943536565528,-4.50757940911709,22.6079400725296));
#43424=CARTESIAN_POINT('Ctrl Pts',(3.32573919581816,-4.80819489445646,21.8088660787087));
#43425=CARTESIAN_POINT('Ctrl Pts',(3.35914562877773,-5.02507740767993,21.2323649186445));
#43426=CARTESIAN_POINT('Ctrl Pts',(3.3925520617373,-5.13603483479161,20.6160142309818));
#43427=CARTESIAN_POINT('Ctrl Pts',(3.42595849469688,-5.13662475218558,19.9998702837641));
#43428=CARTESIAN_POINT('Origin',(25.,0.,20.));
#43429=CARTESIAN_POINT('',(5.17595849469686,-5.13652742584517,20.0001179802973));
#43430=CARTESIAN_POINT('',(4.6990415053031,-5.13690701511421,19.999878736315));
#43431=CARTESIAN_POINT('',(25.,-5.13675,20.));
#43432=CARTESIAN_POINT('Ctrl Pts',(4.6990415053031,-5.13690701511421,19.999878736315));
#43433=CARTESIAN_POINT('Ctrl Pts',(4.66072073224373,-5.13619931580811,20.7065503462862));
#43434=CARTESIAN_POINT('Ctrl Pts',(4.62239995918437,-4.98918393518755,21.4135072640234));
#43435=CARTESIAN_POINT('Ctrl Pts',(4.584079186125,-4.70575595787938,22.0607268921647));
#43436=CARTESIAN_POINT('Ctrl Pts',(4.53777535596212,-4.36328371953613,22.8427765573191));
#43437=CARTESIAN_POINT('Ctrl Pts',(4.49147152579924,-3.821643378755,23.5376072786038));
#43438=CARTESIAN_POINT('Ctrl Pts',(4.44516769563637,-3.14681606646729,24.0605766958687));
#43439=CARTESIAN_POINT('Ctrl Pts',(4.39886386547349,-2.47198875417958,24.5835461131336));
#43440=CARTESIAN_POINT('Ctrl Pts',(4.35256003531062,-1.66397447038526,24.9346542263786));
#43441=CARTESIAN_POINT('Ctrl Pts',(4.30625620514774,-0.821203284337316,
25.0711300146023));
#43442=CARTESIAN_POINT('Ctrl Pts',(4.25995237498486,0.0215679017106736,
25.2076058028261));
#43443=CARTESIAN_POINT('Ctrl Pts',(4.21364854482198,0.899095990012317,25.1294492660285));
#43444=CARTESIAN_POINT('Ctrl Pts',(4.1673447146591,1.70448293156581,24.8461812177436));
#43445=CARTESIAN_POINT('Ctrl Pts',(4.12104088449621,2.50986987311931,24.5629131694588));
#43446=CARTESIAN_POINT('Ctrl Pts',(4.07473705433334,3.2431156679247,24.0745336096866));
#43447=CARTESIAN_POINT('Ctrl Pts',(4.02843322417046,3.81489833763396,23.4405355880622));
#43448=CARTESIAN_POINT('Ctrl Pts',(3.98212939400758,4.38668100734326,22.8065375664377));
#43449=CARTESIAN_POINT('Ctrl Pts',(3.93582556384469,4.79700055195643,22.026921082961));
#43450=CARTESIAN_POINT('Ctrl Pts',(3.88952173368181,4.99587297737494,21.1966568652486));
#43451=CARTESIAN_POINT('Ctrl Pts',(3.84321790351893,5.19474540279343,20.3663926475364));
#43452=CARTESIAN_POINT('Ctrl Pts',(3.79691407335605,5.18217070901731,19.4854806955885));
#43453=CARTESIAN_POINT('Ctrl Pts',(3.75061024319318,4.95968071052699,18.6612312713407));
#43454=CARTESIAN_POINT('Ctrl Pts',(3.7043064130303,4.73719071203664,17.8369818470928));
#43455=CARTESIAN_POINT('Ctrl Pts',(3.65800258286743,4.30478540883215,17.069394950545));
#43456=CARTESIAN_POINT('Ctrl Pts',(3.61169875270455,3.71513922114496,16.4519758982357));
#43457=CARTESIAN_POINT('Ctrl Pts',(3.56539492254167,3.1254930334578,15.8345568459265));
#43458=CARTESIAN_POINT('Ctrl Pts',(3.51909109237879,2.37860596128802,15.3673056378559));
#43459=CARTESIAN_POINT('Ctrl Pts',(3.47278726221591,1.56546172573618,15.1071415262117));
#43460=CARTESIAN_POINT('Ctrl Pts',(3.42648343205303,0.752317490184298,14.8469774145675));
#43461=CARTESIAN_POINT('Ctrl Pts',(3.38017960189015,-0.12708390874967,14.7939003993497));
#43462=CARTESIAN_POINT('Ctrl Pts',(3.33387577172727,-0.965616220544838,
14.9543761759623));
#43463=CARTESIAN_POINT('Ctrl Pts',(3.28757194156439,-1.80414853234001,15.1148519525748));
#43464=CARTESIAN_POINT('Ctrl Pts',(3.24126811140151,-2.6018117569964,15.4888805210176));
#43465=CARTESIAN_POINT('Ctrl Pts',(3.19496428123863,-3.2614367626877,16.0308987538203));
#43466=CARTESIAN_POINT('Ctrl Pts',(3.14866045107576,-3.92106176837896,16.572916986623));
#43467=CARTESIAN_POINT('Ctrl Pts',(3.10235662091288,-4.44264855510516,17.2829248837855));
#43468=CARTESIAN_POINT('Ctrl Pts',(3.05605279075,-4.76265886056433,18.0744312432895));
#43469=CARTESIAN_POINT('Ctrl Pts',(3.02038236226771,-5.00918068552627,18.6841728324984));
#43470=CARTESIAN_POINT('Ctrl Pts',(2.98471193378541,-5.13607730981806,19.3422795377697));
#43471=CARTESIAN_POINT('Ctrl Pts',(2.94904150530311,-5.13675306620054,20.0001330755183));
#43472=CARTESIAN_POINT('Ctrl Pts',(3.42595849469688,-5.13662475218558,19.9998702837641));
#43473=CARTESIAN_POINT('Ctrl Pts',(3.43885589190018,-5.13685250469529,19.7619923507535));
#43474=CARTESIAN_POINT('Ctrl Pts',(3.45175328910349,-5.12062952689274,19.5241452332548));
#43475=CARTESIAN_POINT('Ctrl Pts',(3.46465068630679,-5.08770017461725,19.2886340133428));
#43476=CARTESIAN_POINT('Ctrl Pts',(3.51095451646967,-4.9694782488207,18.4431090321117));
#43477=CARTESIAN_POINT('Ctrl Pts',(3.55725834663255,-4.63592267660959,17.6276921599634));
#43478=CARTESIAN_POINT('Ctrl Pts',(3.60356217679543,-4.12766627689558,16.9417152290282));
#43479=CARTESIAN_POINT('Ctrl Pts',(3.6498660069583,-3.61940987718164,16.2557382980931));
#43480=CARTESIAN_POINT('Ctrl Pts',(3.69616983712118,-2.93645264996485,15.6992013083712));
#43481=CARTESIAN_POINT('Ctrl Pts',(3.74247366728406,-2.16199055912924,15.3399000594395));
#43482=CARTESIAN_POINT('Ctrl Pts',(3.78877749744694,-1.3875284682935,14.9805988105078));
#43483=CARTESIAN_POINT('Ctrl Pts',(3.83508132760981,-0.521561513839056,
14.8185333023666));
#43484=CARTESIAN_POINT('Ctrl Pts',(3.88138515777269,0.330420600639911,14.8734459077808));
#43485=CARTESIAN_POINT('Ctrl Pts',(3.92768898793557,1.18240271511878,14.9283585131949));
#43486=CARTESIAN_POINT('Ctrl Pts',(3.97399281809846,2.02039998962215,15.2002492321646));
#43487=CARTESIAN_POINT('Ctrl Pts',(4.02029664826134,2.74232990974664,15.6559970879515));
#43488=CARTESIAN_POINT('Ctrl Pts',(4.06660047842422,3.46425982987117,16.1117449437385));
#43489=CARTESIAN_POINT('Ctrl Pts',(4.11290430858709,4.07012239561694,16.7513499363429));
#43490=CARTESIAN_POINT('Ctrl Pts',(4.15920813874997,4.48611310191496,17.4968971514132));
#43491=CARTESIAN_POINT('Ctrl Pts',(4.20551196891285,4.90210380821297,18.2424443664834));
#43492=CARTESIAN_POINT('Ctrl Pts',(4.25181579907574,5.12822265506323,19.0939338040197));
#43493=CARTESIAN_POINT('Ctrl Pts',(4.29811962923862,5.13692446882051,19.9476393715678));
#43494=CARTESIAN_POINT('Ctrl Pts',(4.34442345940149,5.14562628257779,20.8013449391159));
#43495=CARTESIAN_POINT('Ctrl Pts',(4.39072728956437,4.93691106324213,21.657266636676));
#43496=CARTESIAN_POINT('Ctrl Pts',(4.43703111972725,4.53620392260352,22.4111384461148));
#43497=CARTESIAN_POINT('Ctrl Pts',(4.48333494989012,4.13549678196491,23.1650102555536));
#43498=CARTESIAN_POINT('Ctrl Pts',(4.529638780053,3.54279772002336,23.8168321768712));
#43499=CARTESIAN_POINT('Ctrl Pts',(4.57594261021588,2.83030770015685,24.2872010631891));
#43500=CARTESIAN_POINT('Ctrl Pts',(4.62224644037876,2.1178176802903,24.757569949507));
#43501=CARTESIAN_POINT('Ctrl Pts',(4.66855027054164,1.28553670249876,25.0464858008252));
#43502=CARTESIAN_POINT('Ctrl Pts',(4.71485410070452,0.434850937701575,25.1187536857869));
#43503=CARTESIAN_POINT('Ctrl Pts',(4.7611579308674,-0.415834827095611,25.1910215707485));
#43504=CARTESIAN_POINT('Ctrl Pts',(4.80746176103028,-1.28492537889845,25.0466414893536));
#43505=CARTESIAN_POINT('Ctrl Pts',(4.85376559119316,-2.06655050610693,24.7032014245071));
#43506=CARTESIAN_POINT('Ctrl Pts',(4.90006942135603,-2.84817563331536,24.3597613596607));
#43507=CARTESIAN_POINT('Ctrl Pts',(4.94637325151891,-3.54233533592946,23.8172613113628));
#43508=CARTESIAN_POINT('Ctrl Pts',(4.99267708168179,-4.06446899544116,23.1417871377409));
#43509=CARTESIAN_POINT('Ctrl Pts',(5.03898091184467,-4.5866026549529,22.4663129641189));
#43510=CARTESIAN_POINT('Ctrl Pts',(5.08528474200755,-4.93671027136222,21.6578646651729));
#43511=CARTESIAN_POINT('Ctrl Pts',(5.13158857217043,-5.07214270142953,20.8149251806834));
#43512=CARTESIAN_POINT('Ctrl Pts',(5.14637854634591,-5.11540137217387,20.5456806459821));
#43513=CARTESIAN_POINT('Ctrl Pts',(5.16116852052139,-5.1367580897038,20.2729171934918));
#43514=CARTESIAN_POINT('Ctrl Pts',(5.17595849469686,-5.13652742584517,20.0001179802973));
#43515=CARTESIAN_POINT('Origin',(25.,0.,20.));
#43516=CARTESIAN_POINT('',(6.92595849469687,-5.13711149676084,19.9999295065412));
#43517=CARTESIAN_POINT('',(6.4490415053031,-5.13634995705138,20.0000574179808));
#43518=CARTESIAN_POINT('',(25.,-5.13675,20.));
#43519=CARTESIAN_POINT('Ctrl Pts',(6.4490415053031,-5.13634995705138,20.0000574179808));
#43520=CARTESIAN_POINT('Ctrl Pts',(6.42933719102783,-5.13649271790615,20.3635369867805));
#43521=CARTESIAN_POINT('Ctrl Pts',(6.40963287675255,-5.09845241040451,20.7269871071621));
#43522=CARTESIAN_POINT('Ctrl Pts',(6.38992856247728,-5.02192199172085,21.0821432290962));
#43523=CARTESIAN_POINT('Ctrl Pts',(6.3436247323144,-4.8420805895022,21.9167365329586));
#43524=CARTESIAN_POINT('Ctrl Pts',(6.29732090215152,-4.44968956026618,22.7055288187839));
#43525=CARTESIAN_POINT('Ctrl Pts',(6.25101707198864,-3.89254889586517,23.3524315880428));
#43526=CARTESIAN_POINT('Ctrl Pts',(6.20471324182576,-3.33540823146419,23.9993343573016));
#43527=CARTESIAN_POINT('Ctrl Pts',(6.15840941166288,-2.61351793189824,24.504347609994));
#43528=CARTESIAN_POINT('Ctrl Pts',(6.11210558150001,-1.81481668043628,24.8059520259381));
#43529=CARTESIAN_POINT('Ctrl Pts',(6.06580175133713,-1.01611542897428,25.1075564418822));
#43530=CARTESIAN_POINT('Ctrl Pts',(6.01949792117425,-0.140603225616253,
25.2057520210781));
#43531=CARTESIAN_POINT('Ctrl Pts',(5.97319409101137,0.70506745017449,25.0885768491704));
#43532=CARTESIAN_POINT('Ctrl Pts',(5.92689026084849,1.55073812596523,24.9714016772627));
#43533=CARTESIAN_POINT('Ctrl Pts',(5.88058643068561,2.3665672741887,24.6388557542514));
#43534=CARTESIAN_POINT('Ctrl Pts',(5.83428260052273,3.05317284038265,24.1314489063715));
#43535=CARTESIAN_POINT('Ctrl Pts',(5.78797877035985,3.73977840657657,23.6240420584916));
#43536=CARTESIAN_POINT('Ctrl Pts',(5.74167494019697,4.297160390741,22.941774285743));
#43537=CARTESIAN_POINT('Ctrl Pts',(5.6953711100341,4.65742005840793,22.1677575645694));
#43538=CARTESIAN_POINT('Ctrl Pts',(5.64906727987122,5.01767972607487,21.3937408433957));
#43539=CARTESIAN_POINT('Ctrl Pts',(5.60276344970835,5.1808170772443,20.527975173797));
#43540=CARTESIAN_POINT('Ctrl Pts',(5.55645961954547,5.12695917019303,19.6759257394025));
#43541=CARTESIAN_POINT('Ctrl Pts',(5.51015578938259,5.07310126314176,18.8238763050079));
#43542=CARTESIAN_POINT('Ctrl Pts',(5.4638519592197,4.80224809786972,17.9855431058176));
#43543=CARTESIAN_POINT('Ctrl Pts',(5.41754812905682,4.34739425918792,17.2630495776525));
#43544=CARTESIAN_POINT('Ctrl Pts',(5.37124429889395,3.89254042050617,16.5405560494875));
#43545=CARTESIAN_POINT('Ctrl Pts',(5.32494046873107,3.25368590841469,15.9339021923476));
#43546=CARTESIAN_POINT('Ctrl Pts',(5.27863663856819,2.50865421580088,15.5169889042349));
#43547=CARTESIAN_POINT('Ctrl Pts',(5.23233280840532,1.76362252318708,15.1000756161223));
#43548=CARTESIAN_POINT('Ctrl Pts',(5.18602897824244,0.912413650050945,14.8729028970369));
#43549=CARTESIAN_POINT('Ctrl Pts',(5.13972514807956,0.0587195112657737,
14.86314430043));
#43550=CARTESIAN_POINT('Ctrl Pts',(5.09342131791668,-0.794974627519446,
14.8533857038231));
#43551=CARTESIAN_POINT('Ctrl Pts',(5.0471174877538,-1.6511540319537,15.0610412296947));
#43552=CARTESIAN_POINT('Ctrl Pts',(5.00081365759092,-2.40552129076381,15.4608148551871));
#43553=CARTESIAN_POINT('Ctrl Pts',(4.95450982742804,-3.15988854957393,15.8605884806794));
#43554=CARTESIAN_POINT('Ctrl Pts',(4.90820599726516,-3.81244366275989,16.4524802057925));
#43555=CARTESIAN_POINT('Ctrl Pts',(4.86190216710228,-4.28369416803413,17.1643874146917));
#43556=CARTESIAN_POINT('Ctrl Pts',(4.8155983369394,-4.75494467330841,17.8762946235911));
#43557=CARTESIAN_POINT('Ctrl Pts',(4.76929450677652,-5.04489057067094,18.7082173162766));
#43558=CARTESIAN_POINT('Ctrl Pts',(4.72299067661363,-5.11821145139949,19.5588129671315));
#43559=CARTESIAN_POINT('Ctrl Pts',(4.71500761951012,-5.13085240951628,19.7054607418163));
#43560=CARTESIAN_POINT('Ctrl Pts',(4.70702456240661,-5.13705444439399,19.8526635481691));
#43561=CARTESIAN_POINT('Ctrl Pts',(4.6990415053031,-5.13690701511421,19.999878736315));
#43562=CARTESIAN_POINT('Ctrl Pts',(5.17595849469686,-5.13652742584517,20.0001179802973));
#43563=CARTESIAN_POINT('Ctrl Pts',(5.20747235068426,-5.13603593698008,19.4188488708258));
#43564=CARTESIAN_POINT('Ctrl Pts',(5.23898620667166,-5.03753493650671,18.8374174031187));
#43565=CARTESIAN_POINT('Ctrl Pts',(5.27050006265906,-4.84406756639821,18.2895193523615));
#43566=CARTESIAN_POINT('Ctrl Pts',(5.31680389282194,-4.55980275757426,17.4844836785621));
#43567=CARTESIAN_POINT('Ctrl Pts',(5.36310772298482,-4.07051589620105,16.7518430009963));
#43568=CARTESIAN_POINT('Ctrl Pts',(5.4094115531477,-3.43581055688794,16.1808455843009));
#43569=CARTESIAN_POINT('Ctrl Pts',(5.45571538331058,-2.80110521757488,15.6098481676055));
#43570=CARTESIAN_POINT('Ctrl Pts',(5.50201921347345,-2.02098140032195,15.2004940117805));
#43571=CARTESIAN_POINT('Ctrl Pts',(5.54832304363632,-1.19047163474926,15.0026495099269));
#43572=CARTESIAN_POINT('Ctrl Pts',(5.5946268737992,-0.35996186917647,14.8048050080732));
#43573=CARTESIAN_POINT('Ctrl Pts',(5.64093070396209,0.520933844716072,14.818470160191));
#43574=CARTESIAN_POINT('Ctrl Pts',(5.68723453412497,1.34490722307478,15.0419803151764));
#43575=CARTESIAN_POINT('Ctrl Pts',(5.73353836428785,2.16888060143339,15.2654904701619));
#43576=CARTESIAN_POINT('Ctrl Pts',(5.77984219445072,2.93593164425815,15.698845628015));
#43577=CARTESIAN_POINT('Ctrl Pts',(5.8261460246136,3.55262031121797,16.2892556598307));
#43578=CARTESIAN_POINT('Ctrl Pts',(5.87244985477648,4.16930897817779,16.8796656916465));
#43579=CARTESIAN_POINT('Ctrl Pts',(5.91875368493936,4.63563526927263,17.6271305974248));
#43580=CARTESIAN_POINT('Ctrl Pts',(5.96505751510224,4.89479260317398,18.4405962659754));
#43581=CARTESIAN_POINT('Ctrl Pts',(6.01136134526512,5.15394993707534,19.254061934526));
#43582=CARTESIAN_POINT('Ctrl Pts',(6.057665175428,5.20593831378318,20.133528365849));
#43583=CARTESIAN_POINT('Ctrl Pts',(6.10396900559087,5.04442465277859,20.9718613873471));
#43584=CARTESIAN_POINT('Ctrl Pts',(6.15027283575375,4.88291099177398,21.8101944088453));
#43585=CARTESIAN_POINT('Ctrl Pts',(6.19657666591664,4.50789529305694,22.6073940205188));
#43586=CARTESIAN_POINT('Ctrl Pts',(6.24288049607952,3.96506093368653,23.2663475666147));
#43587=CARTESIAN_POINT('Ctrl Pts',(6.2891843262424,3.42222657431609,23.9253011127106));
#43588=CARTESIAN_POINT('Ctrl Pts',(6.33548815640528,2.71157355429229,24.4460085932289));
#43589=CARTESIAN_POINT('Ctrl Pts',(6.38179198656816,1.91967166251458,24.7650388604832));
#43590=CARTESIAN_POINT('Ctrl Pts',(6.42809581673104,1.12776977073697,25.0840691277375));
#43591=CARTESIAN_POINT('Ctrl Pts',(6.47439964689391,0.254619007205502,25.2014221817279));
#43592=CARTESIAN_POINT('Ctrl Pts',(6.52070347705679,-0.593415812696665,
25.1028023974105));
#43593=CARTESIAN_POINT('Ctrl Pts',(6.56700730721967,-1.44145063259883,25.004182613093));
#43594=CARTESIAN_POINT('Ctrl Pts',(6.61331113738255,-2.26436950887167,24.6895899904676));
#43595=CARTESIAN_POINT('Ctrl Pts',(6.65961496754543,-2.96192673595563,24.1973473342824));
#43596=CARTESIAN_POINT('Ctrl Pts',(6.70591879770831,-3.65948396303959,23.7051046780972));
#43597=CARTESIAN_POINT('Ctrl Pts',(6.75222262787118,-4.23167954093465,23.0352119883522));
#43598=CARTESIAN_POINT('Ctrl Pts',(6.79852645803406,-4.60881018408253,22.2692737430451));
#43599=CARTESIAN_POINT('Ctrl Pts',(6.84100380358832,-4.95477527145751,21.566631577058));
#43600=CARTESIAN_POINT('Ctrl Pts',(6.8834811491426,-5.1365830919474,20.7831620910917));
#43601=CARTESIAN_POINT('Ctrl Pts',(6.92595849469687,-5.13711149676084,19.9999295065412));
#43602=CARTESIAN_POINT('Origin',(25.,0.,20.));
#43603=CARTESIAN_POINT('',(8.67595849469684,-5.13631265723153,19.9999878238786));
#43604=CARTESIAN_POINT('',(8.19904150530309,-5.13718402169266,20.000021201249));
#43605=CARTESIAN_POINT('',(25.,-5.13675,20.));
#43606=CARTESIAN_POINT('Ctrl Pts',(8.19904150530309,-5.13718402169266,20.000021201249));
#43607=CARTESIAN_POINT('Ctrl Pts',(8.19795364981191,-5.13718867916289,20.0200791611231));
#43608=CARTESIAN_POINT('Ctrl Pts',(8.19686579432073,-5.13707366050557,20.0401370673822));
#43609=CARTESIAN_POINT('Ctrl Pts',(8.19577793882955,-5.13683863807768,20.0601935674349));
#43610=CARTESIAN_POINT('Ctrl Pts',(8.14947410866668,-5.12683506805018,20.9138848707705));
#43611=CARTESIAN_POINT('Ctrl Pts',(8.1031702785038,-4.89941809766086,21.7650285199751));
#43612=CARTESIAN_POINT('Ctrl Pts',(8.05686644834092,-4.48229103438051,22.5099405455748));
#43613=CARTESIAN_POINT('Ctrl Pts',(8.01056261817804,-4.06516397110018,23.2548525711745));
#43614=CARTESIAN_POINT('Ctrl Pts',(7.96425878801516,-3.45832681492884,23.8935329731693));
#43615=CARTESIAN_POINT('Ctrl Pts',(7.91795495785228,-2.73570279285051,24.348179468283));
#43616=CARTESIAN_POINT('Ctrl Pts',(7.87165112768941,-2.01307877077215,24.8028259633968));
#43617=CARTESIAN_POINT('Ctrl Pts',(7.82534729752653,-1.17466788278679,25.0734385516296));
#43618=CARTESIAN_POINT('Ctrl Pts',(7.77904346736365,-0.322603028549861,
25.1270519546011));
#43619=CARTESIAN_POINT('Ctrl Pts',(7.73273963720077,0.529461825687064,25.1806653575726));
#43620=CARTESIAN_POINT('Ctrl Pts',(7.68643580703788,1.39518064617555,25.0172795752827));
#43621=CARTESIAN_POINT('Ctrl Pts',(7.640131976875,2.1690939563155,24.6567978126481));
#43622=CARTESIAN_POINT('Ctrl Pts',(7.59382814671212,2.9430072664554,24.2963160500134));
#43623=CARTESIAN_POINT('Ctrl Pts',(7.54752431654925,3.62511506624678,23.7387383070339));
#43624=CARTESIAN_POINT('Ctrl Pts',(7.50122048638637,4.13232486671005,23.051987164976));
#43625=CARTESIAN_POINT('Ctrl Pts',(7.4549166562235,4.63953466717333,22.365236022918));
#43626=CARTESIAN_POINT('Ctrl Pts',(7.40861282606061,4.97184646830851,21.5493114817816));
#43627=CARTESIAN_POINT('Ctrl Pts',(7.36230899589774,5.08877896396127,20.7036072165303));
#43628=CARTESIAN_POINT('Ctrl Pts',(7.31600516573486,5.20571145961404,19.8579029512789));
#43629=CARTESIAN_POINT('Ctrl Pts',(7.26970133557198,5.10726464978438,18.9824189619126));
#43630=CARTESIAN_POINT('Ctrl Pts',(7.22339750540911,4.80543105304975,18.183804290944));
#43631=CARTESIAN_POINT('Ctrl Pts',(7.17709367524623,4.50359745631513,17.3851896199754));
#43632=CARTESIAN_POINT('Ctrl Pts',(7.13078984508334,3.99837707267555,16.6634442674047));
#43633=CARTESIAN_POINT('Ctrl Pts',(7.08448601492046,3.35131445443296,16.1064892594579));
#43634=CARTESIAN_POINT('Ctrl Pts',(7.03818218475758,2.70425183619038,15.5495342515111));
#43635=CARTESIAN_POINT('Ctrl Pts',(6.9918783545947,1.91534698334479,15.1573695881882));
#43636=CARTESIAN_POINT('Ctrl Pts',(6.94557452443182,1.08070210702917,14.9777676860712));
#43637=CARTESIAN_POINT('Ctrl Pts',(6.89927069426894,0.24605723071356,14.7981657839541));
#43638=CARTESIAN_POINT('Ctrl Pts',(6.85296686410606,-0.63432766907208,14.8311266430428));
#43639=CARTESIAN_POINT('Ctrl Pts',(6.80666303394318,-1.45320653443837,15.0726350624828));
#43640=CARTESIAN_POINT('Ctrl Pts',(6.7603592037803,-2.27208539980461,15.3141434819228));
#43641=CARTESIAN_POINT('Ctrl Pts',(6.71405537361743,-3.0294582307515,15.764199461714));
#43642=CARTESIAN_POINT('Ctrl Pts',(6.66775154345455,-3.63306395999889,16.3679784249312));
#43643=CARTESIAN_POINT('Ctrl Pts',(6.62144771329168,-4.23666968924627,16.9717573881484));
#43644=CARTESIAN_POINT('Ctrl Pts',(6.57514388312879,-4.68650831679415,17.7292593347915));
#43645=CARTESIAN_POINT('Ctrl Pts',(6.52884005296591,-4.92778174296745,18.5482074690628));
#43646=CARTESIAN_POINT('Ctrl Pts',(6.50224053707831,-5.06638272500672,19.0186571884932));
#43647=CARTESIAN_POINT('Ctrl Pts',(6.4756410211907,-5.13615723937687,19.5093841354682));
#43648=CARTESIAN_POINT('Ctrl Pts',(6.4490415053031,-5.13634995705138,20.0000574179808));
#43649=CARTESIAN_POINT('Ctrl Pts',(6.92595849469687,-5.13711149676084,19.9999295065412));
#43650=CARTESIAN_POINT('Ctrl Pts',(6.92978497930548,-5.13715909702539,19.9293736045506));
#43651=CARTESIAN_POINT('Ctrl Pts',(6.93361146391409,-5.13573562608275,19.8588196250004));
#43652=CARTESIAN_POINT('Ctrl Pts',(6.9374379485227,-5.13282856734164,19.788326827259));
#43653=CARTESIAN_POINT('Ctrl Pts',(6.98374177868558,-5.09765059905217,18.9353019576494));
#43654=CARTESIAN_POINT('Ctrl Pts',(7.03004560884846,-4.84522895407254,18.0912360192996));
#43655=CARTESIAN_POINT('Ctrl Pts',(7.07634943901133,-4.40631294029821,17.3589507944877));
#43656=CARTESIAN_POINT('Ctrl Pts',(7.12265326917421,-3.96739692652388,16.6266655696758));
#43657=CARTESIAN_POINT('Ctrl Pts',(7.1689570993371,-3.34198654395484,16.0061610584017));
#43658=CARTESIAN_POINT('Ctrl Pts',(7.21526092949998,-2.60626755873719,15.5730254071148));
#43659=CARTESIAN_POINT('Ctrl Pts',(7.26156475966286,-1.87054857351955,15.139889755828));
#43660=CARTESIAN_POINT('Ctrl Pts',(7.30786858982574,-1.02452098565328,14.8941229645282));
#43661=CARTESIAN_POINT('Ctrl Pts',(7.35417241998862,-0.171245540144829,
14.8656636652088));
#43662=CARTESIAN_POINT('Ctrl Pts',(7.40047625015149,0.68202990536357,14.8372043658894));
#43663=CARTESIAN_POINT('Ctrl Pts',(7.44678008031437,1.54255320851417,15.0260525585502));
#43664=CARTESIAN_POINT('Ctrl Pts',(7.49308391047725,2.30549779628496,15.4092032777412));
#43665=CARTESIAN_POINT('Ctrl Pts',(7.53938774064013,3.06844238405575,15.7923539969322));
#43666=CARTESIAN_POINT('Ctrl Pts',(7.58569157080301,3.73380825644674,16.3698072426534));
#43667=CARTESIAN_POINT('Ctrl Pts',(7.63199540096588,4.22054237985248,17.0712192547673));
#43668=CARTESIAN_POINT('Ctrl Pts',(7.67829923112877,4.70727650325828,17.7726312668813));
#43669=CARTESIAN_POINT('Ctrl Pts',(7.72460306129164,5.0153788776788,18.5980020453883));
#43670=CARTESIAN_POINT('Ctrl Pts',(7.77090689145452,5.10731732248371,19.4467872007676));
#43671=CARTESIAN_POINT('Ctrl Pts',(7.8172107216174,5.19925576728861,20.2955723561469));
#43672=CARTESIAN_POINT('Ctrl Pts',(7.86351455178028,5.07503028247796,21.1677718883985));
#43673=CARTESIAN_POINT('Ctrl Pts',(7.90981838194316,4.74977367364457,21.9571368585078));
#43674=CARTESIAN_POINT('Ctrl Pts',(7.95612221210604,4.42451706481121,22.746501828617));
#43675=CARTESIAN_POINT('Ctrl Pts',(8.00242604226892,3.89822933195513,23.4530322365837));
#43676=CARTESIAN_POINT('Ctrl Pts',(8.04872987243179,3.23502139369626,23.9906604987275));
#43677=CARTESIAN_POINT('Ctrl Pts',(8.09503370259467,2.57181345543735,24.5282887608713));
#43678=CARTESIAN_POINT('Ctrl Pts',(8.14133753275755,1.7716853117756,24.8970148771921));
#43679=CARTESIAN_POINT('Ctrl Pts',(8.18764136292043,0.932106364145535,25.0519216501937));
#43680=CARTESIAN_POINT('Ctrl Pts',(8.23394519308331,0.0925274165154677,
25.2068284231954));
#43681=CARTESIAN_POINT('Ctrl Pts',(8.28024902324619,-0.786502335082951,
25.1479158528779));
#43682=CARTESIAN_POINT('Ctrl Pts',(8.32655285340907,-1.59790191317113,24.8823605059091));
#43683=CARTESIAN_POINT('Ctrl Pts',(8.37285668357194,-2.40930149125927,24.6168051589403));
#43684=CARTESIAN_POINT('Ctrl Pts',(8.41916051373481,-3.15307089583721,24.1446070353203));
#43685=CARTESIAN_POINT('Ctrl Pts',(8.46546434389769,-3.73860619146813,23.5232880068046));
#43686=CARTESIAN_POINT('Ctrl Pts',(8.51176817406057,-4.32414148709909,22.9019689782888));
#43687=CARTESIAN_POINT('Ctrl Pts',(8.55807200422345,-4.75144267378303,22.1315290448773));
#43688=CARTESIAN_POINT('Ctrl Pts',(8.60437583438634,-4.96845710066864,21.3058210721964));
#43689=CARTESIAN_POINT('Ctrl Pts',(8.6282367211565,-5.08028708642134,20.8803244259781));
#43690=CARTESIAN_POINT('Ctrl Pts',(8.65209760792667,-5.13627632047532,20.4401515877795));
#43691=CARTESIAN_POINT('Ctrl Pts',(8.67595849469684,-5.13631265723153,19.9999878238786));
#43692=CARTESIAN_POINT('Origin',(25.,0.,20.));
#43693=CARTESIAN_POINT('',(10.4259584946969,-5.13705094320386,20.000091771118));
#43694=CARTESIAN_POINT('',(9.94904150530308,-5.13641270033522,19.9999113248429));
#43695=CARTESIAN_POINT('',(25.,-5.13675,20.));
#43696=CARTESIAN_POINT('Ctrl Pts',(9.94904150530308,-5.13641270033522,19.9999113248429));
#43697=CARTESIAN_POINT('Ctrl Pts',(9.92026627843311,-5.13608567565037,20.530700733121));
#43698=CARTESIAN_POINT('Ctrl Pts',(9.89149105156315,-5.05423141803617,21.061588697543));
#43699=CARTESIAN_POINT('Ctrl Pts',(9.86271582469318,-4.89240905155667,21.5668657030692));
#43700=CARTESIAN_POINT('Ctrl Pts',(9.81641199453031,-4.63201161288895,22.3799352491347));
#43701=CARTESIAN_POINT('Ctrl Pts',(9.77010816436743,-4.16454609932103,23.1266882093746));
#43702=CARTESIAN_POINT('Ctrl Pts',(9.72380433420456,-3.54695786911788,23.7161571998384));
#43703=CARTESIAN_POINT('Ctrl Pts',(9.67750050404168,-2.92936963891474,24.3056261903022));
#43704=CARTESIAN_POINT('Ctrl Pts',(9.6311966738788,-2.16165869207638,24.73781121099));
#43705=CARTESIAN_POINT('Ctrl Pts',(9.58489284371592,-1.33734545661897,24.9600646758756));
#43706=CARTESIAN_POINT('Ctrl Pts',(9.53858901355304,-0.51303222116157,25.1823181407612));
#43707=CARTESIAN_POINT('Ctrl Pts',(9.49228518339017,0.367883302914878,25.1946400498445));
#43708=CARTESIAN_POINT('Ctrl Pts',(9.44598135322729,1.19809041853487,24.99552938218));
#43709=CARTESIAN_POINT('Ctrl Pts',(9.39967752306441,2.02829753415495,24.7964187145154));
#43710=CARTESIAN_POINT('Ctrl Pts',(9.35337369290152,2.80779624131857,24.3858754701028));
#43711=CARTESIAN_POINT('Ctrl Pts',(9.30706986273864,3.44163015959083,23.8139108935321));
#43712=CARTESIAN_POINT('Ctrl Pts',(9.26076603257576,4.07546407786306,23.2419463169615));
#43713=CARTESIAN_POINT('Ctrl Pts',(9.21446220241288,4.56363320724394,22.5085604082327));
#43714=CARTESIAN_POINT('Ctrl Pts',(9.16815837225,4.84667013214954,21.7030922139854));
#43715=CARTESIAN_POINT('Ctrl Pts',(9.12185454208712,5.12970705705514,20.8976240197382));
#43716=CARTESIAN_POINT('Ctrl Pts',(9.07555071192424,5.20761177748545,20.0200735399724));
#43717=CARTESIAN_POINT('Ctrl Pts',(9.02924688176136,5.07089415548018,19.1773415513561));
#43718=CARTESIAN_POINT('Ctrl Pts',(8.98294305159848,4.93417653347491,18.3346095627398));
#43719=CARTESIAN_POINT('Ctrl Pts',(8.93663922143561,4.58283656903409,17.526696065273));
#43720=CARTESIAN_POINT('Ctrl Pts',(8.89033539127273,4.05967352663219,16.8520188506965));
#43721=CARTESIAN_POINT('Ctrl Pts',(8.84403156110985,3.5365104842303,16.1773416361201));
#43722=CARTESIAN_POINT('Ctrl Pts',(8.79772773094698,2.84152436386732,15.6359007044339));
#43723=CARTESIAN_POINT('Ctrl Pts',(8.7514239007841,2.05937645597988,15.2936528951039));
#43724=CARTESIAN_POINT('Ctrl Pts',(8.70512007062122,1.27722854809239,14.9514050857739));
#43725=CARTESIAN_POINT('Ctrl Pts',(8.65881624045834,0.407918852680429,14.8083503988));
#43726=CARTESIAN_POINT('Ctrl Pts',(8.61251241029546,-0.442655723186566,
14.8819153611983));
#43727=CARTESIAN_POINT('Ctrl Pts',(8.56620858013258,-1.29323029905356,14.9554803235965));
#43728=CARTESIAN_POINT('Ctrl Pts',(8.5199047499697,-2.12506975537558,15.2456649353669));
#43729=CARTESIAN_POINT('Ctrl Pts',(8.47360091980682,-2.83684170615976,15.717119708257));
#43730=CARTESIAN_POINT('Ctrl Pts',(8.42729708964395,-3.54861365694389,16.1885744811471));
#43731=CARTESIAN_POINT('Ctrl Pts',(8.38099325948107,-4.14031810219019,16.8412994151569));
#43732=CARTESIAN_POINT('Ctrl Pts',(8.33468942931819,-4.5398752399805,17.5957813608949));
#43733=CARTESIAN_POINT('Ctrl Pts',(8.28947345464649,-4.93004524014409,18.3325376168839));
#43734=CARTESIAN_POINT('Ctrl Pts',(8.24425747997479,-5.13699043710604,19.1663257214849));
#43735=CARTESIAN_POINT('Ctrl Pts',(8.19904150530309,-5.13718402169266,20.000021201249));
#43736=CARTESIAN_POINT('Ctrl Pts',(8.67595849469684,-5.13631265723153,19.9999878238786));
#43737=CARTESIAN_POINT('Ctrl Pts',(8.69840143808955,-5.13634683466049,19.5859809794599));
#43738=CARTESIAN_POINT('Ctrl Pts',(8.72084438148226,-5.08688057336706,19.1719821628957));
#43739=CARTESIAN_POINT('Ctrl Pts',(8.74328732487497,-4.98782055609996,18.7702111018865));
#43740=CARTESIAN_POINT('Ctrl Pts',(8.78959115503785,-4.78344191755838,17.9412851162078));
#43741=CARTESIAN_POINT('Ctrl Pts',(8.83589498520072,-4.36795697338792,17.164409156801));
#43742=CARTESIAN_POINT('Ctrl Pts',(8.8821988153636,-3.79197895239965,16.5342201082102));
#43743=CARTESIAN_POINT('Ctrl Pts',(8.92850264552648,-3.21600093141144,15.9040310596194));
#43744=CARTESIAN_POINT('Ctrl Pts',(8.97480647568936,-2.47952983360547,15.4205289218445));
#43745=CARTESIAN_POINT('Ctrl Pts',(9.02111030585223,-1.67228053483701,15.1426125904369));
#43746=CARTESIAN_POINT('Ctrl Pts',(9.06741413601512,-0.86503123606842,14.8646962590293));
#43747=CARTESIAN_POINT('Ctrl Pts',(9.113717966178,0.0129962636626844,14.7923657339889));
#43748=CARTESIAN_POINT('Ctrl Pts',(9.16002179634088,0.854843078433148,14.9344321201832));
#43749=CARTESIAN_POINT('Ctrl Pts',(9.20632562650376,1.69668989320356,15.0764985063775));
#43750=CARTESIAN_POINT('Ctrl Pts',(9.25262945666664,2.50235602301334,15.4329618038064));
#43751=CARTESIAN_POINT('Ctrl Pts',(9.29893328682952,3.17369744424494,15.9603986377156));
#43752=CARTESIAN_POINT('Ctrl Pts',(9.3452371169924,3.84503886547653,16.4878354716248));
#43753=CARTESIAN_POINT('Ctrl Pts',(9.39154094715527,4.38205557812995,17.1862458420142));
#43754=CARTESIAN_POINT('Ctrl Pts',(9.43784477731815,4.71932968888737,17.9705513257629));
#43755=CARTESIAN_POINT('Ctrl Pts',(9.48414860748104,5.05660379964479,18.7548568095115));
#43756=CARTESIAN_POINT('Ctrl Pts',(9.53045243764392,5.19413530850622,19.6250574066194));
#43757=CARTESIAN_POINT('Ctrl Pts',(9.5767562678068,5.11517050676475,20.475147682832));
#43758=CARTESIAN_POINT('Ctrl Pts',(9.62306009796968,5.03620570502329,21.3252379590446));
#43759=CARTESIAN_POINT('Ctrl Pts',(9.66936392813255,4.74074459267895,22.1552179143621));
#43760=CARTESIAN_POINT('Ctrl Pts',(9.71566775829543,4.26477942671644,22.86398168207));
#43761=CARTESIAN_POINT('Ctrl Pts',(9.76197158845831,3.78881426075394,23.572745449778));
#43762=CARTESIAN_POINT('Ctrl Pts',(9.80827541862118,3.13234504117326,24.1602930298765));
#43763=CARTESIAN_POINT('Ctrl Pts',(9.85457924878406,2.37534103589674,24.5550509982833));
#43764=CARTESIAN_POINT('Ctrl Pts',(9.90088307894694,1.61833703062018,24.9498089666901));
#43765=CARTESIAN_POINT('Ctrl Pts',(9.94718690910982,0.76079823964778,25.1517773234051));
#43766=CARTESIAN_POINT('Ctrl Pts',(9.9934907392727,-0.092812329032254,25.1363528408158));
#43767=CARTESIAN_POINT('Ctrl Pts',(10.0397945694356,-0.946422897712288,
25.1209283582265));
#43768=CARTESIAN_POINT('Ctrl Pts',(10.0860983995985,-1.79610524409995,24.8881110363328));
#43769=CARTESIAN_POINT('Ctrl Pts',(10.1324022297613,-2.53835341059595,24.4662620385164));
#43770=CARTESIAN_POINT('Ctrl Pts',(10.1787060599242,-3.28060157709191,24.0444130407));
#43771=CARTESIAN_POINT('Ctrl Pts',(10.2250098900871,-3.91541556369621,23.4335323669608));
#43772=CARTESIAN_POINT('Ctrl Pts',(10.27131372025,-4.36546408318106,22.7080358144295));
#43773=CARTESIAN_POINT('Ctrl Pts',(10.3176175504128,-4.81551260266596,21.9825392618981));
#43774=CARTESIAN_POINT('Ctrl Pts',(10.3639213805757,-5.08079565503136,21.1424268305745));
#43775=CARTESIAN_POINT('Ctrl Pts',(10.4102252107386,-5.12899719124236,20.290038697426));
#43776=CARTESIAN_POINT('Ctrl Pts',(10.4154696387247,-5.13445655571799,20.1934961832375));
#43777=CARTESIAN_POINT('Ctrl Pts',(10.4207140667108,-5.13713117626548,20.0967961950884));
#43778=CARTESIAN_POINT('Ctrl Pts',(10.4259584946969,-5.13705094320386,20.000091771118));
#43779=CARTESIAN_POINT('Origin',(25.,0.,20.));
#43780=CARTESIAN_POINT('',(12.1759584946968,-5.13659925691256,19.9998724976161));
#43781=CARTESIAN_POINT('',(11.6990415053031,-5.13678078662753,20.0001322193276));
#43782=CARTESIAN_POINT('',(25.,-5.13675,20.));
#43783=CARTESIAN_POINT('Ctrl Pts',(11.6990415053031,-5.13678078662753,20.0001322193276));
#43784=CARTESIAN_POINT('Ctrl Pts',(11.6888827372172,-5.13697407873776,20.1874828625214));
#43785=CARTESIAN_POINT('Ctrl Pts',(11.6787239691313,-5.12692244990169,20.3748128764519));
#43786=CARTESIAN_POINT('Ctrl Pts',(11.6685652010455,-5.10646780565129,20.5610000080705));
#43787=CARTESIAN_POINT('Ctrl Pts',(11.6222613708826,-5.01323520447304,21.4096439822325));
#43788=CARTESIAN_POINT('Ctrl Pts',(11.5759575407197,-4.70387462893425,22.234543990903));
#43789=CARTESIAN_POINT('Ctrl Pts',(11.5296537105568,-4.21607153025175,22.9352129924435));
#43790=CARTESIAN_POINT('Ctrl Pts',(11.483349880394,-3.72826843156924,23.6358819939839));
#43791=CARTESIAN_POINT('Ctrl Pts',(11.4370460502311,-3.062022809743,24.2123199883943));
#43792=CARTESIAN_POINT('Ctrl Pts',(11.3907422200682,-2.29849486702586,24.5943068906489));
#43793=CARTESIAN_POINT('Ctrl Pts',(11.3444383899053,-1.53496692430872,24.9762937929036));
#43794=CARTESIAN_POINT('Ctrl Pts',(11.2981345597424,-0.674156660700671,
25.1638296030025));
#43795=CARTESIAN_POINT('Ctrl Pts',(11.2518307295796,0.179074394045612,25.134069226316));
#43796=CARTESIAN_POINT('Ctrl Pts',(11.2055268994167,1.0323054487919,25.1043088496296));
#43797=CARTESIAN_POINT('Ctrl Pts',(11.1592230692538,1.87795729467641,24.8572522861577));
#43798=CARTESIAN_POINT('Ctrl Pts',(11.1129192390909,2.61301495854358,24.4229952843787));
#43799=CARTESIAN_POINT('Ctrl Pts',(11.066615408928,3.34807262241072,23.9887382825997));
#43800=CARTESIAN_POINT('Ctrl Pts',(11.0203115787652,3.97253610426052,23.3672808425136));
#43801=CARTESIAN_POINT('Ctrl Pts',(10.9740077486023,4.41033498677829,22.6343271937266));
#43802=CARTESIAN_POINT('Ctrl Pts',(10.9277039184394,4.84813386929609,21.9013735449396));
#43803=CARTESIAN_POINT('Ctrl Pts',(10.8814000882765,5.09926815248184,21.0569236874518));
#43804=CARTESIAN_POINT('Ctrl Pts',(10.8350962581136,5.1331453512996,20.2038461715107));
#43805=CARTESIAN_POINT('Ctrl Pts',(10.7887924279508,5.16702255011737,19.3507686555696));
#43806=CARTESIAN_POINT('Ctrl Pts',(10.7424885977879,4.98364266456715,18.4890634811753));
#43807=CARTESIAN_POINT('Ctrl Pts',(10.696184767625,4.60534452602403,17.7237011936416));
#43808=CARTESIAN_POINT('Ctrl Pts',(10.6498809374621,4.22704638748092,16.9583389061079));
#43809=CARTESIAN_POINT('Ctrl Pts',(10.6035771072993,3.65382999594493,16.289319505435));
#43810=CARTESIAN_POINT('Ctrl Pts',(10.5572732771364,2.95552298967378,15.7981410879567));
#43811=CARTESIAN_POINT('Ctrl Pts',(10.5109694469735,2.25721598340259,15.3069626704783));
#43812=CARTESIAN_POINT('Ctrl Pts',(10.4646656168106,1.43381836239623,14.9936252361946));
#43813=CARTESIAN_POINT('Ctrl Pts',(10.4183617866477,0.58563415157598,14.8962986862752));
#43814=CARTESIAN_POINT('Ctrl Pts',(10.3720579564849,-0.262550059244267,
14.7989721363558));
#43815=CARTESIAN_POINT('Ctrl Pts',(10.325754126322,-1.1355208598784,14.9176564708008));
#43816=CARTESIAN_POINT('Ctrl Pts',(10.2794502961591,-1.92693535752653,15.2378938916565));
#43817=CARTESIAN_POINT('Ctrl Pts',(10.2331464659962,-2.71834985517461,15.5581313125122));
#43818=CARTESIAN_POINT('Ctrl Pts',(10.1868426358333,-3.4282080498367,16.0799218197787));
#43819=CARTESIAN_POINT('Ctrl Pts',(10.1405388056705,-3.9700369760445,16.7397023344413));
#43820=CARTESIAN_POINT('Ctrl Pts',(10.0942349755076,-4.51186590225237,17.3994828491039));
#43821=CARTESIAN_POINT('Ctrl Pts',(10.0479311453447,-4.88566556000591,18.1972533711626));
#43822=CARTESIAN_POINT('Ctrl Pts',(10.0016273151818,-5.04590070699891,19.0358316981376));
#43823=CARTESIAN_POINT('Ctrl Pts',(9.9840987118889,-5.10655871985318,19.3532807465613));
#43824=CARTESIAN_POINT('Ctrl Pts',(9.96657010859599,-5.1366119093977,19.6765777500346));
#43825=CARTESIAN_POINT('Ctrl Pts',(9.94904150530308,-5.13641270033522,19.9999113248429));
#43826=CARTESIAN_POINT('Ctrl Pts',(10.4259584946969,-5.13705094320386,20.000091771118));
#43827=CARTESIAN_POINT('Ctrl Pts',(10.4670178968737,-5.1364227867007,19.2429785365343));
#43828=CARTESIAN_POINT('Ctrl Pts',(10.5080772990505,-4.96693434567107,18.4855934058136));
#43829=CARTESIAN_POINT('Ctrl Pts',(10.5491367012273,-4.6429297443183,17.8013781536833));
#43830=CARTESIAN_POINT('Ctrl Pts',(10.5954405313901,-4.27754074112656,17.0297695780623));
#43831=CARTESIAN_POINT('Ctrl Pts',(10.641744361553,-3.71564271468642,16.3512162617936));
#43832=CARTESIAN_POINT('Ctrl Pts',(10.6880481917159,-3.02568453126784,15.8483776964874));
#43833=CARTESIAN_POINT('Ctrl Pts',(10.7343520218788,-2.3357263478493,15.3455391311813));
#43834=CARTESIAN_POINT('Ctrl Pts',(10.7806558520416,-1.51770800745234,15.0184153168377));
#43835=CARTESIAN_POINT('Ctrl Pts',(10.8269596822045,-0.671278245885745,
14.9068555733833));
#43836=CARTESIAN_POINT('Ctrl Pts',(10.8732635123674,0.175151515680903,14.7952958299288));
#43837=CARTESIAN_POINT('Ctrl Pts',(10.9195673425303,1.0499926984172,14.8993001573634));
#43838=CARTESIAN_POINT('Ctrl Pts',(10.9658711726932,1.84667456473939,15.2061990356585));
#43839=CARTESIAN_POINT('Ctrl Pts',(11.012175002856,2.64335643106154,15.5130979139536));
#43840=CARTESIAN_POINT('Ctrl Pts',(11.0584788330189,3.3618789809696,16.0228913431091));
#43841=CARTESIAN_POINT('Ctrl Pts',(11.1047826631818,3.91471378116012,16.6734776950437));
#43842=CARTESIAN_POINT('Ctrl Pts',(11.1510864933447,4.46754858135067,17.3240640469784));
#43843=CARTESIAN_POINT('Ctrl Pts',(11.1973903235076,4.85469563182366,18.1154433216923));
#43844=CARTESIAN_POINT('Ctrl Pts',(11.2436941536704,5.02899374774183,18.9512118808118));
#43845=CARTESIAN_POINT('Ctrl Pts',(11.2899979838333,5.20329186365999,19.7869804399314));
#43846=CARTESIAN_POINT('Ctrl Pts',(11.3363018139962,5.16474104502332,20.6671382834566));
#43847=CARTESIAN_POINT('Ctrl Pts',(11.3826056441591,4.91803744612548,21.484467012865));
#43848=CARTESIAN_POINT('Ctrl Pts',(11.4289094743219,4.67133384722765,22.3017957422732));
#43849=CARTESIAN_POINT('Ctrl Pts',(11.4752133044848,4.21647746806867,23.0562953575646));
#43850=CARTESIAN_POINT('Ctrl Pts',(11.5215171346477,3.60887765697164,23.6560547986576));
#43851=CARTESIAN_POINT('Ctrl Pts',(11.5678209648106,3.00127784587458,24.2558142397507));
#43852=CARTESIAN_POINT('Ctrl Pts',(11.6141247949735,2.24093460283946,24.7008335066453));
#43853=CARTESIAN_POINT('Ctrl Pts',(11.6604286251363,1.42047084254621,24.9369015808757));
#43854=CARTESIAN_POINT('Ctrl Pts',(11.7067324552992,0.600007082252954,25.1729696551061));
#43855=CARTESIAN_POINT('Ctrl Pts',(11.7530362854621,-0.280577195298433,
25.2000865366723));
#43856=CARTESIAN_POINT('Ctrl Pts',(11.799340115625,-1.1140116445696,25.0149489219273));
#43857=CARTESIAN_POINT('Ctrl Pts',(11.8456439457879,-1.94744609384073,24.8298113071824));
#43858=CARTESIAN_POINT('Ctrl Pts',(11.8919477759507,-2.73373071483164,24.4324191961262));
#43859=CARTESIAN_POINT('Ctrl Pts',(11.9382516061136,-3.37708248581986,23.8711817985914));
#43860=CARTESIAN_POINT('Ctrl Pts',(11.9845554362765,-4.02043425680805,23.3099444010566));
#43861=CARTESIAN_POINT('Ctrl Pts',(12.0308592664394,-4.52085317779356,22.5848617170433));
#43862=CARTESIAN_POINT('Ctrl Pts',(12.0771630966022,-4.81737959739892,21.7842613172799));
#43863=CARTESIAN_POINT('Ctrl Pts',(12.1100948959671,-5.02827248730623,21.2148654024344));
#43864=CARTESIAN_POINT('Ctrl Pts',(12.143026695332,-5.13603221298305,20.6072710206123));
#43865=CARTESIAN_POINT('Ctrl Pts',(12.1759584946968,-5.13659925691256,19.9998724976161));
#43866=CARTESIAN_POINT('Origin',(25.,0.,20.));
#43867=CARTESIAN_POINT('',(13.9259584946968,-5.13655067277195,20.0001216380244));
#43868=CARTESIAN_POINT('',(13.4490415053031,-5.13687989532564,19.9998753684823));
#43869=CARTESIAN_POINT('',(25.,-5.13675,20.));
#43870=CARTESIAN_POINT('Ctrl Pts',(13.4490415053031,-5.13687989532564,19.9998753684823));
#43871=CARTESIAN_POINT('Ctrl Pts',(13.4111953658384,-5.13617111687111,20.6978049124174));
#43872=CARTESIAN_POINT('Ctrl Pts',(13.3733492263738,-4.99287560925193,21.3960165694796));
#43873=CARTESIAN_POINT('Ctrl Pts',(13.3355030869091,-4.71622959740109,22.0366425419808));
#43874=CARTESIAN_POINT('Ctrl Pts',(13.2891992567462,-4.37775993763722,22.820432821471));
#43875=CARTESIAN_POINT('Ctrl Pts',(13.2428954265833,-3.83967888536099,23.5180235117641));
#43876=CARTESIAN_POINT('Ctrl Pts',(13.1965915964205,-3.16753398880461,24.0444360409056));
#43877=CARTESIAN_POINT('Ctrl Pts',(13.1502877662576,-2.49538909224818,24.570848570047));
#43878=CARTESIAN_POINT('Ctrl Pts',(13.1039839360947,-1.68918035141157,24.9260829380368));
#43879=CARTESIAN_POINT('Ctrl Pts',(13.0576801059318,-0.847117889289556,
25.0668654749119));
#43880=CARTESIAN_POINT('Ctrl Pts',(13.0113762757689,-0.00505542716753793,
25.2076480117869));
#43881=CARTESIAN_POINT('Ctrl Pts',(12.9650724456061,0.872860756239892,25.1339787175473));
#43882=CARTESIAN_POINT('Ctrl Pts',(12.9187686154432,1.67968533525682,24.854831782228));
#43883=CARTESIAN_POINT('Ctrl Pts',(12.8724647852803,2.4865099142737,24.5756848469088));
#43884=CARTESIAN_POINT('Ctrl Pts',(12.8261609551174,3.22224288890008,24.0910602705099));
#43885=CARTESIAN_POINT('Ctrl Pts',(12.7798571249545,3.79725929940857,23.4599936809571));
#43886=CARTESIAN_POINT('Ctrl Pts',(12.7335532947917,4.37227570991707,22.8289270914043));
#43887=CARTESIAN_POINT('Ctrl Pts',(12.6872494646288,4.78657555630767,22.0514184886975));
#43888=CARTESIAN_POINT('Ctrl Pts',(12.6409456344659,4.98968997510898,21.2221818242411));
#43889=CARTESIAN_POINT('Ctrl Pts',(12.594641804303,5.1928043939103,20.3929451597845));
#43890=CARTESIAN_POINT('Ctrl Pts',(12.5483379741402,5.18473338512231,19.5119804335783));
#43891=CARTESIAN_POINT('Ctrl Pts',(12.5020341439773,4.96646013675279,18.6866043363656));
#43892=CARTESIAN_POINT('Ctrl Pts',(12.4557303138144,4.74818688838326,17.8612282391528));
#43893=CARTESIAN_POINT('Ctrl Pts',(12.4094264836515,4.31971140043221,17.0914407709334));
#43894=CARTESIAN_POINT('Ctrl Pts',(12.3631226534886,3.73322937388923,16.4710153158254));
#43895=CARTESIAN_POINT('Ctrl Pts',(12.3168188233258,3.14674734734626,15.8505898607174));
#43896=CARTESIAN_POINT('Ctrl Pts',(12.2705149931629,2.40225878221136,15.3795264187206));
#43897=CARTESIAN_POINT('Ctrl Pts',(12.224211163,1.5904552200749,15.1152086378081));
#43898=CARTESIAN_POINT('Ctrl Pts',(12.1779073328371,0.778651657938445,14.8508908568955));
#43899=CARTESIAN_POINT('Ctrl Pts',(12.1316035026742,-0.100466901199574,
14.7933187370672));
#43900=CARTESIAN_POINT('Ctrl Pts',(12.0852996725114,-0.939808661571305,
14.9495055550131));
#43901=CARTESIAN_POINT('Ctrl Pts',(12.0389958423485,-1.77915042194299,15.1056923729589));
#43902=CARTESIAN_POINT('Ctrl Pts',(11.9926920121856,-2.57871538354839,15.475638128679));
#43903=CARTESIAN_POINT('Ctrl Pts',(11.9463881820227,-3.24110275023627,16.0142770515728));
#43904=CARTESIAN_POINT('Ctrl Pts',(11.9000843518599,-3.90349011692416,16.5529159744666));
#43905=CARTESIAN_POINT('Ctrl Pts',(11.853780521697,-4.42869988869453,17.2602480645341));
#43906=CARTESIAN_POINT('Ctrl Pts',(11.8074766915341,-4.75275246117088,18.0501080793945));
#43907=CARTESIAN_POINT('Ctrl Pts',(11.7713316294571,-5.00570994454042,18.6666777922856));
#43908=CARTESIAN_POINT('Ctrl Pts',(11.7351865673801,-5.13609305015553,19.3335355836762));
#43909=CARTESIAN_POINT('Ctrl Pts',(11.6990415053031,-5.13678078662753,20.0001322193276));
#43910=CARTESIAN_POINT('Ctrl Pts',(12.1759584946968,-5.13659925691256,19.9998724976161));
#43911=CARTESIAN_POINT('Ctrl Pts',(12.1893305254949,-5.13682950636858,19.7532369686496));
#43912=CARTESIAN_POINT('Ctrl Pts',(12.2027025562929,-5.11938599591789,19.5066337325767));
#43913=CARTESIAN_POINT('Ctrl Pts',(12.2160745870909,-5.08399694390373,19.2626332607487));
#43914=CARTESIAN_POINT('Ctrl Pts',(12.2623784172538,-4.96145395257798,18.4177237194945));
#43915=CARTESIAN_POINT('Ctrl Pts',(12.3086822474166,-4.62373405170133,17.6040227524996));
#43916=CARTESIAN_POINT('Ctrl Pts',(12.3549860775795,-4.1119773472077,16.9206531650645));
#43917=CARTESIAN_POINT('Ctrl Pts',(12.4012899077424,-3.60022064271406,16.2372835776294));
#43918=CARTESIAN_POINT('Ctrl Pts',(12.4475937379053,-2.91442713460346,15.6842453697541));
#43919=CARTESIAN_POINT('Ctrl Pts',(12.4938975680682,-2.13813829466724,15.3289081290715));
#43920=CARTESIAN_POINT('Ctrl Pts',(12.540201398231,-1.36184945473103,14.973570888389));
#43921=CARTESIAN_POINT('Ctrl Pts',(12.5865052283939,-0.495065282969215,
14.8159346148992));
#43922=CARTESIAN_POINT('Ctrl Pts',(12.6328090585568,0.35662496586725,14.87520212423));
#43923=CARTESIAN_POINT('Ctrl Pts',(12.6791128887197,1.20831521470367,14.9344696335608));
#43924=CARTESIAN_POINT('Ctrl Pts',(12.7254167188826,2.04491154061474,15.2106409257122));
#43925=CARTESIAN_POINT('Ctrl Pts',(12.7717205490454,2.76450208888721,15.6700735763393));
#43926=CARTESIAN_POINT('Ctrl Pts',(12.8180243792083,3.48409263715968,16.1295062269664));
#43927=CARTESIAN_POINT('Ctrl Pts',(12.8643282093712,4.08667740779355,16.7722002360692));
#43928=CARTESIAN_POINT('Ctrl Pts',(12.9106320395341,4.49885118767081,17.5198643938346));
#43929=CARTESIAN_POINT('Ctrl Pts',(12.9569358696969,4.91102496754808,18.2675285515999));
#43930=CARTESIAN_POINT('Ctrl Pts',(13.0032396998598,5.13278775666873,19.1201628580279));
#43931=CARTESIAN_POINT('Ctrl Pts',(13.0495435300227,5.13712502431383,19.973901755897));
#43932=CARTESIAN_POINT('Ctrl Pts',(13.0958473601856,5.14146229195894,20.8276406537662));
#43933=CARTESIAN_POINT('Ctrl Pts',(13.1421511903485,4.92837403812845,21.6824841430764));
#43934=CARTESIAN_POINT('Ctrl Pts',(13.1884550205113,4.52381808560127,22.4342975500467));
#43935=CARTESIAN_POINT('Ctrl Pts',(13.2347588506742,4.11926213307414,23.1861109570169));
#43936=CARTESIAN_POINT('Ctrl Pts',(13.2810626808371,3.52323848185035,23.8348942816473));
#43937=CARTESIAN_POINT('Ctrl Pts',(13.327366511,2.8083530875956,24.3016145305186));
#43938=CARTESIAN_POINT('Ctrl Pts',(13.3736703411629,2.09346769334081,24.76833477939));
#43939=CARTESIAN_POINT('Ctrl Pts',(13.4199741713257,1.25972055605504,25.0529919525024));
#43940=CARTESIAN_POINT('Ctrl Pts',(13.4662780014886,0.408676450159372,25.1209098989205));
#43941=CARTESIAN_POINT('Ctrl Pts',(13.5125818316515,-0.442367655736295,
25.1888278453385));
#43942=CARTESIAN_POINT('Ctrl Pts',(13.5588856618144,-1.31070873024186,25.0400065650622));
#43943=CARTESIAN_POINT('Ctrl Pts',(13.6051894919772,-2.09056786101249,24.6925750555829));
#43944=CARTESIAN_POINT('Ctrl Pts',(13.6514933221401,-2.87042699178307,24.3451435461035));
#43945=CARTESIAN_POINT('Ctrl Pts',(13.697797152303,-3.56180417881871,23.7991018074213));
#43946=CARTESIAN_POINT('Ctrl Pts',(13.7441009824659,-4.08047776197707,23.120967136608));
#43947=CARTESIAN_POINT('Ctrl Pts',(13.7904048126288,-4.59915134513546,22.4428324657947));
#43948=CARTESIAN_POINT('Ctrl Pts',(13.8367086427916,-4.94512132441653,21.6326048628505));
#43949=CARTESIAN_POINT('Ctrl Pts',(13.8830124729545,-5.07624259211229,20.7889840174565));
#43950=CARTESIAN_POINT('Ctrl Pts',(13.8973278135353,-5.11678018042506,20.5281693142155));
#43951=CARTESIAN_POINT('Ctrl Pts',(13.9116431541161,-5.13678241017023,20.2641628664098));
#43952=CARTESIAN_POINT('Ctrl Pts',(13.9259584946968,-5.13655067277195,20.0001216380244));
#43953=CARTESIAN_POINT('Origin',(25.,0.,20.));
#43954=CARTESIAN_POINT('',(15.6759584946968,-5.13709264059427,19.9999219868719));
#43955=CARTESIAN_POINT('',(15.1990415053031,-5.1363612583734,20.0000647015142));
#43956=CARTESIAN_POINT('',(25.,-5.13675,20.));
#43957=CARTESIAN_POINT('Ctrl Pts',(15.1990415053031,-5.1363612583734,20.0000647015142));
#43958=CARTESIAN_POINT('Ctrl Pts',(15.1798118246225,-5.13651868439003,20.3547866133449));
#43959=CARTESIAN_POINT('Ctrl Pts',(15.1605821439419,-5.10030269833592,20.7094768313789));
#43960=CARTESIAN_POINT('Ctrl Pts',(15.1413524632614,-5.02738864798306,21.0564553191401));
#43961=CARTESIAN_POINT('Ctrl Pts',(15.0950486330985,-4.85181631997047,21.8919571267025));
#43962=CARTESIAN_POINT('Ctrl Pts',(15.0487448029356,-4.46346299222078,22.6827451405394));
#43963=CARTESIAN_POINT('Ctrl Pts',(15.0024409727727,-3.90963679493877,23.3324877480449));
#43964=CARTESIAN_POINT('Ctrl Pts',(14.9561371426099,-3.35581059765675,23.9822303555503));
#43965=CARTESIAN_POINT('Ctrl Pts',(14.909833312447,-2.63651153084241,24.4909275567245));
#43966=CARTESIAN_POINT('Ctrl Pts',(14.8635294822841,-1.83936262094488,24.7966112629521));
#43967=CARTESIAN_POINT('Ctrl Pts',(14.8172256521212,-1.04221371104731,25.1022949691798));
#43968=CARTESIAN_POINT('Ctrl Pts',(14.7709218219583,-0.167214958066531,
25.204965180461));
#43969=CARTESIAN_POINT('Ctrl Pts',(14.7246179917955,0.679043705641541,25.0921148951135));
#43970=CARTESIAN_POINT('Ctrl Pts',(14.6783141616326,1.52530236934961,24.979264609766));
#43971=CARTESIAN_POINT('Ctrl Pts',(14.6320103314697,2.34282094378498,24.6508938277899));
#43972=CARTESIAN_POINT('Ctrl Pts',(14.5857065013068,3.03201157324853,24.1470037712661));
#43973=CARTESIAN_POINT('Ctrl Pts',(14.5394026711439,3.72120220271208,23.6431137147422));
#43974=CARTESIAN_POINT('Ctrl Pts',(14.4930988409811,4.2820648872038,22.9637043836706));
#43975=CARTESIAN_POINT('Ctrl Pts',(14.4467950108182,4.64627688295148,22.1915395470214));
#43976=CARTESIAN_POINT('Ctrl Pts',(14.4004911806553,5.01048887869915,21.4193747103723));
#43977=CARTESIAN_POINT('Ctrl Pts',(14.3541873504924,5.17805018570278,20.5544543681455));
#43978=CARTESIAN_POINT('Ctrl Pts',(14.3078835203295,5.12854894815326,19.7021407285239));
#43979=CARTESIAN_POINT('Ctrl Pts',(14.2615796901667,5.07904771060375,18.8498270889023));
#43980=CARTESIAN_POINT('Ctrl Pts',(14.2152758600038,4.81248392850112,18.0101201518859));
#43981=CARTESIAN_POINT('Ctrl Pts',(14.1689720298409,4.36132966584095,17.2853106982448));
#43982=CARTESIAN_POINT('Ctrl Pts',(14.122668199678,3.91017540318078,16.5605012446038));
#43983=CARTESIAN_POINT('Ctrl Pts',(14.0763643695151,3.27443065996308,15.9505892743381));
#43984=CARTESIAN_POINT('Ctrl Pts',(14.0300605393523,2.53154010561662,15.5298725797956));
#43985=CARTESIAN_POINT('Ctrl Pts',(13.9837567091894,1.78864955127012,15.1091558852532));
#43986=CARTESIAN_POINT('Ctrl Pts',(13.9374528790265,0.938613185794851,14.8776344664341));
#43987=CARTESIAN_POINT('Ctrl Pts',(13.8911490488637,0.0849800924179688,
14.863511623385));
#43988=CARTESIAN_POINT('Ctrl Pts',(13.8448452187008,-0.768653000958913,
14.849388780336));
#43989=CARTESIAN_POINT('Ctrl Pts',(13.7985413885379,-1.62588282223741,15.052664513057));
#43990=CARTESIAN_POINT('Ctrl Pts',(13.752237558375,-2.38228400126439,15.448576333));
#43991=CARTESIAN_POINT('Ctrl Pts',(13.7059337282121,-3.13868518029134,15.8444881529429));
#43992=CARTESIAN_POINT('Ctrl Pts',(13.6596298980493,-3.79425771706679,16.4330360601078));
#43993=CARTESIAN_POINT('Ctrl Pts',(13.6133260678864,-4.26914157509214,17.1425247733308));
#43994=CARTESIAN_POINT('Ctrl Pts',(13.5670222377235,-4.74402543311751,17.8520134865539));
#43995=CARTESIAN_POINT('Ctrl Pts',(13.5207184075606,-5.03822061239277,18.6824430058351));
#43996=CARTESIAN_POINT('Ctrl Pts',(13.4744145773977,-5.11588906840463,19.5326526998193));
#43997=CARTESIAN_POINT('Ctrl Pts',(13.4659568866995,-5.13007570859501,19.6879489376263));
#43998=CARTESIAN_POINT('Ctrl Pts',(13.4574991960013,-5.137038290053,19.8439051084966));
#43999=CARTESIAN_POINT('Ctrl Pts',(13.4490415053031,-5.13687989532564,19.9998753684823));
#44000=CARTESIAN_POINT('Ctrl Pts',(13.9259584946968,-5.13655067277195,20.0001216380244));
#44001=CARTESIAN_POINT('Ctrl Pts',(13.9579469842789,-5.13603284161668,19.4101056313638));
#44002=CARTESIAN_POINT('Ctrl Pts',(13.989935473861,-5.03448157070668,18.8199159562585));
#44003=CARTESIAN_POINT('Ctrl Pts',(14.0219239634432,-4.83525970650011,18.2647771888103));
#44004=CARTESIAN_POINT('Ctrl Pts',(14.068227793606,-4.54688299708175,17.4612052934018));
#44005=CARTESIAN_POINT('Ctrl Pts',(14.1145316237689,-4.05385702213458,16.7310755904285));
#44006=CARTESIAN_POINT('Ctrl Pts',(14.1608354539318,-3.41624084476046,16.1633304645348));
#44007=CARTESIAN_POINT('Ctrl Pts',(14.2071392840947,-2.77862466738633,15.595585338641));
#44008=CARTESIAN_POINT('Ctrl Pts',(14.2534431142576,-1.99641828758527,15.1902247898268));
#44009=CARTESIAN_POINT('Ctrl Pts',(14.2997469444204,-1.16490792699735,14.9966287210127));
#44010=CARTESIAN_POINT('Ctrl Pts',(14.3460507745833,-0.333397566409359,
14.8030326521985));
#44011=CARTESIAN_POINT('Ctrl Pts',(14.3923546047462,0.54741677496555,14.8212010633846));
#44012=CARTESIAN_POINT('Ctrl Pts',(14.4386584349091,1.37023672584908,15.0489207288803));
#44013=CARTESIAN_POINT('Ctrl Pts',(14.4849622650719,2.19305667673255,15.276640394376));
#44014=CARTESIAN_POINT('Ctrl Pts',(14.5312660952348,2.95788223712471,15.7139113141812));
#44015=CARTESIAN_POINT('Ctrl Pts',(14.5775699253977,3.57154446882019,16.3074663520807));
#44016=CARTESIAN_POINT('Ctrl Pts',(14.6238737555606,4.18520670051574,16.9010213899802));
#44017=CARTESIAN_POINT('Ctrl Pts',(14.6701775857235,4.64770560351457,17.650860545974));
#44018=CARTESIAN_POINT('Ctrl Pts',(14.7164814158864,4.90270083833917,18.4656404842655));
#44019=CARTESIAN_POINT('Ctrl Pts',(14.7627852460492,5.15769607316375,19.2804204225568));
#44020=CARTESIAN_POINT('Ctrl Pts',(14.8090890762121,5.20518763981414,20.1601411431458));
#44021=CARTESIAN_POINT('Ctrl Pts',(14.855392906375,5.03939024675767,20.9976374966191));
#44022=CARTESIAN_POINT('Ctrl Pts',(14.9016967365379,4.87359285370119,21.8351338500923));
#44023=CARTESIAN_POINT('Ctrl Pts',(14.9480005667007,4.49450650093785,22.6304058364498));
#44024=CARTESIAN_POINT('Ctrl Pts',(14.9943043968636,3.94831044136419,23.2865756179329));
#44025=CARTESIAN_POINT('Ctrl Pts',(15.0406082270265,3.40211438179051,23.942745399416));
#44026=CARTESIAN_POINT('Ctrl Pts',(15.0869120571894,2.68880861540652,24.4598129760247));
#44027=CARTESIAN_POINT('Ctrl Pts',(15.1332158873523,1.89528608134946,24.7747906031176));
#44028=CARTESIAN_POINT('Ctrl Pts',(15.1795197175151,1.10176354729244,25.0897682302105));
#44029=CARTESIAN_POINT('Ctrl Pts',(15.225823547678,0.228024245562298,25.2026559077876));
#44030=CARTESIAN_POINT('Ctrl Pts',(15.2721273778409,-0.619495314359142,
25.0997019706316));
#44031=CARTESIAN_POINT('Ctrl Pts',(15.3184312080038,-1.46701487428056,24.9967480334755));
#44032=CARTESIAN_POINT('Ctrl Pts',(15.3647350381666,-2.28831469239333,24.6779524815862));
#44033=CARTESIAN_POINT('Ctrl Pts',(15.4110388683295,-2.98334629233299,24.1821501089511));
#44034=CARTESIAN_POINT('Ctrl Pts',(15.4573426984924,-3.6783778922727,23.6863477363159));
#44035=CARTESIAN_POINT('Ctrl Pts',(15.5036465286553,-4.24714127403926,23.0135385429349));
#44036=CARTESIAN_POINT('Ctrl Pts',(15.5499503588182,-4.62035125273102,22.2456822872266));
#44037=CARTESIAN_POINT('Ctrl Pts',(15.5919530707777,-4.95889411582207,21.5491514598327));
#44038=CARTESIAN_POINT('Ctrl Pts',(15.6339557827373,-5.13652580276168,20.7744111288028));
#44039=CARTESIAN_POINT('Ctrl Pts',(15.6759584946968,-5.13709264059427,19.9999219868719));
#44040=CARTESIAN_POINT('Origin',(25.,0.,20.));
#44041=CARTESIAN_POINT('',(17.4259584946968,-5.13631117261779,19.999995970574));
#44042=CARTESIAN_POINT('',(16.9490415053031,-5.13718894078376,20.0000119941014));
#44043=CARTESIAN_POINT('',(25.,-5.13675,20.));
#44044=CARTESIAN_POINT('Ctrl Pts',(16.9490415053031,-5.13718894078376,20.0000119941014));
#44045=CARTESIAN_POINT('Ctrl Pts',(16.9484282834066,-5.1371904673118,20.0113185931481));
#44046=CARTESIAN_POINT('Ctrl Pts',(16.9478150615101,-5.13715392013654,20.0226251822843));
#44047=CARTESIAN_POINT('Ctrl Pts',(16.9472018396137,-5.13707923933338,20.0339315195396));
#44048=CARTESIAN_POINT('Ctrl Pts',(16.9008980094508,-5.1314401595061,20.8876628084021));
#44049=CARTESIAN_POINT('Ctrl Pts',(16.8545941792879,-4.90837749602317,21.7399579674652));
#44050=CARTESIAN_POINT('Ctrl Pts',(16.808290349125,-4.49506412670956,22.4869927535031));
#44051=CARTESIAN_POINT('Ctrl Pts',(16.7619865189621,-4.08175075739599,23.234027539541));
#44052=CARTESIAN_POINT('Ctrl Pts',(16.7156826887993,-3.47818668225178,23.8758019525536));
#44053=CARTESIAN_POINT('Ctrl Pts',(16.6693788586364,-2.7578964105667,24.3341368053848));
#44054=CARTESIAN_POINT('Ctrl Pts',(16.6230750284735,-2.03760613888161,24.792471658216));
#44055=CARTESIAN_POINT('Ctrl Pts',(16.5767711983106,-1.20058967065567,25.0673669508658));
#44056=CARTESIAN_POINT('Ctrl Pts',(16.5304673681477,-0.348810041178962,
25.1253356977257));
#44057=CARTESIAN_POINT('Ctrl Pts',(16.4841635379848,0.502969588297676,25.1833044445855));
#44058=CARTESIAN_POINT('Ctrl Pts',(16.437859707822,1.36951237902513,25.0243466456554));
#44059=CARTESIAN_POINT('Ctrl Pts',(16.3915558776591,2.14525848062353,24.667826101144));
#44060=CARTESIAN_POINT('Ctrl Pts',(16.3452520474962,2.92100458222195,24.3113055566325));
#44061=CARTESIAN_POINT('Ctrl Pts',(16.2989482173333,3.60595399469137,23.7572222665397));
#44062=CARTESIAN_POINT('Ctrl Pts',(16.2526443871705,4.11666807164104,23.0730731275288));
#44063=CARTESIAN_POINT('Ctrl Pts',(16.2063405570076,4.62738214859073,22.3889239885178));
#44064=CARTESIAN_POINT('Ctrl Pts',(16.1600367268447,4.96386089002065,21.5747090005889));
#44065=CARTESIAN_POINT('Ctrl Pts',(16.1137328966818,5.08511538461402,20.7296135856535));
#44066=CARTESIAN_POINT('Ctrl Pts',(16.067429066519,5.20636987920738,19.884518170718));
#44067=CARTESIAN_POINT('Ctrl Pts',(16.0211252363561,5.1124001269642,19.0085423287761));
#44068=CARTESIAN_POINT('Ctrl Pts',(15.9748214061932,4.81465326366721,18.2083950184634));
#44069=CARTESIAN_POINT('Ctrl Pts',(15.9285175760303,4.51690640037024,17.4082477081506));
#44070=CARTESIAN_POINT('Ctrl Pts',(15.8822137458674,4.01538242601949,16.683928929467));
#44071=CARTESIAN_POINT('Ctrl Pts',(15.8359099157046,3.37117560654253,16.1236731963029));
#44072=CARTESIAN_POINT('Ctrl Pts',(15.7896060855417,2.72696878706553,15.5634174631387));
#44073=CARTESIAN_POINT('Ctrl Pts',(15.7433022553788,1.94007912246231,15.1672247754941));
#44074=CARTESIAN_POINT('Ctrl Pts',(15.6969984252159,1.10636333919777,14.983358232753));
#44075=CARTESIAN_POINT('Ctrl Pts',(15.650694595053,0.272647555933252,14.7994916900119));
#44076=CARTESIAN_POINT('Ctrl Pts',(15.6043907648902,-0.607894345992638,
14.8279512921742));
#44077=CARTESIAN_POINT('Ctrl Pts',(15.5580869347273,-1.42799718312314,15.0652701690771));
#44078=CARTESIAN_POINT('Ctrl Pts',(15.5117831045644,-2.24810002025363,15.3025890459799));
#44079=CARTESIAN_POINT('Ctrl Pts',(15.4654792744015,-3.00776379258878,15.7487671976232));
#44080=CARTESIAN_POINT('Ctrl Pts',(15.4191754442386,-3.61444835669347,16.3494524334007));
#44081=CARTESIAN_POINT('Ctrl Pts',(15.3728716140758,-4.22113292079819,16.9501376691782));
#44082=CARTESIAN_POINT('Ctrl Pts',(15.3265677839129,-4.67483827667241,17.7053299890898));
#44083=CARTESIAN_POINT('Ctrl Pts',(15.28026395375,-4.92029529047178,18.5230339496896));
#44084=CARTESIAN_POINT('Ctrl Pts',(15.2531898042677,-5.06381559666912,19.001150753066));
#44085=CARTESIAN_POINT('Ctrl Pts',(15.2261156547854,-5.13613961270089,19.5006391403159));
#44086=CARTESIAN_POINT('Ctrl Pts',(15.1990415053031,-5.1363612583734,20.0000647015142));
#44087=CARTESIAN_POINT('Ctrl Pts',(15.6759584946968,-5.13709264059427,19.9999219868719));
#44088=CARTESIAN_POINT('Ctrl Pts',(15.6802596129002,-5.13715068533487,19.9206135519823));
#44089=CARTESIAN_POINT('Ctrl Pts',(15.6845607311035,-5.13535203559877,19.8413077510508));
#44090=CARTESIAN_POINT('Ctrl Pts',(15.6888618493068,-5.13167934602173,19.7620888329847));
#44091=CARTESIAN_POINT('Ctrl Pts',(15.7351656794697,-5.09214088500373,18.9092549524864));
#44092=CARTESIAN_POINT('Ctrl Pts',(15.7814695096325,-4.83540738735081,18.0664905095254));
#44093=CARTESIAN_POINT('Ctrl Pts',(15.8277733397954,-4.39275341894673,17.3364587418047));
#44094=CARTESIAN_POINT('Ctrl Pts',(15.8740771699583,-3.95009945054265,16.606426974084));
#44095=CARTESIAN_POINT('Ctrl Pts',(15.9203810001212,-3.32152501138741,15.9891278816036));
#44096=CARTESIAN_POINT('Ctrl Pts',(15.9666848302841,-2.58360130426497,15.5597591355449));
#44097=CARTESIAN_POINT('Ctrl Pts',(16.012988660447,-1.8456775971425,15.1303903894862));
#44098=CARTESIAN_POINT('Ctrl Pts',(16.0592924906098,-0.9984046220528,14.8889519898493));
#44099=CARTESIAN_POINT('Ctrl Pts',(16.1055963207727,-0.144994833635566,
14.8648552959049));
#44100=CARTESIAN_POINT('Ctrl Pts',(16.1519001509356,0.708414954781668,14.8407586019606));
#44101=CARTESIAN_POINT('Ctrl Pts',(16.1982039810985,1.56796155652645,15.0340036137088));
#44102=CARTESIAN_POINT('Ctrl Pts',(16.2445078112613,2.32893737764552,15.4210497573371));
#44103=CARTESIAN_POINT('Ctrl Pts',(16.2908116414242,3.08991319876458,15.8080959009655));
#44104=CARTESIAN_POINT('Ctrl Pts',(16.3371154715871,3.75231823925793,16.3889431764739));
#44105=CARTESIAN_POINT('Ctrl Pts',(16.38341930175,4.2354601458875,17.0928343723869));
#44106=CARTESIAN_POINT('Ctrl Pts',(16.4297231319129,4.71860205251706,17.7967255682998));
#44107=CARTESIAN_POINT('Ctrl Pts',(16.4760269620757,5.02248082528284,18.6236606846172));
#44108=CARTESIAN_POINT('Ctrl Pts',(16.5223307922386,5.1100787910474,19.4729047685055));
#44109=CARTESIAN_POINT('Ctrl Pts',(16.5686346224015,5.19767675681196,20.3221488523938));
#44110=CARTESIAN_POINT('Ctrl Pts',(16.6149384525644,5.06899391557534,21.193701903853));
#44111=CARTESIAN_POINT('Ctrl Pts',(16.6612422827273,4.73970605578413,21.9813937363734));
#44112=CARTESIAN_POINT('Ctrl Pts',(16.7075461128901,4.41041819599293,22.7690855688939));
#44113=CARTESIAN_POINT('Ctrl Pts',(16.753849943053,3.88052531764715,23.4729161824757));
#44114=CARTESIAN_POINT('Ctrl Pts',(16.8001537732159,3.21457750823702,24.0071468749365));
#44115=CARTESIAN_POINT('Ctrl Pts',(16.8464576033788,2.54862969882685,24.5413775673973));
#44116=CARTESIAN_POINT('Ctrl Pts',(16.8927614335417,1.74662695835231,24.9060083387372));
#44117=CARTESIAN_POINT('Ctrl Pts',(16.9390652637045,0.90626704645616,25.056620875079));
#44118=CARTESIAN_POINT('Ctrl Pts',(16.9853690938674,0.0659071345600125,
25.2072334114207));
#44119=CARTESIAN_POINT('Ctrl Pts',(17.0316729240303,-0.812809948757753,
25.1438277127643));
#44120=CARTESIAN_POINT('Ctrl Pts',(17.0779767541932,-1.62284131440529,24.8741276862671));
#44121=CARTESIAN_POINT('Ctrl Pts',(17.124280584356,-2.43287268005278,24.60442765977));
#44122=CARTESIAN_POINT('Ctrl Pts',(17.1705844145189,-3.17421832803005,24.128433305432));
#44123=CARTESIAN_POINT('Ctrl Pts',(17.2168882446818,-3.7565695782378,23.504128941354));
#44124=CARTESIAN_POINT('Ctrl Pts',(17.2631920748447,-4.33892082844559,22.879824577276));
#44125=CARTESIAN_POINT('Ctrl Pts',(17.3094959050076,-4.76227768088384,22.1072102034581));
#44126=CARTESIAN_POINT('Ctrl Pts',(17.3557997351704,-4.97506797260937,21.2804035698533));
#44127=CARTESIAN_POINT('Ctrl Pts',(17.3791859883459,-5.08254002444763,20.8628158845016));
#44128=CARTESIAN_POINT('Ctrl Pts',(17.4025722415214,-5.13629939103057,20.4314044857201));
#44129=CARTESIAN_POINT('Ctrl Pts',(17.4259584946968,-5.13631117261779,19.999995970574));
#44130=CARTESIAN_POINT('Origin',(25.,0.,20.));
#44131=CARTESIAN_POINT('',(19.1759584946968,-5.13707257898892,20.0000850551338));
#44132=CARTESIAN_POINT('',(18.6990415053031,-5.13639668367057,19.9999176386971));
#44133=CARTESIAN_POINT('',(25.,-5.13675,20.));
#44134=CARTESIAN_POINT('Ctrl Pts',(18.6990415053031,-5.13639668367057,19.9999176386971));
#44135=CARTESIAN_POINT('Ctrl Pts',(18.6707409120278,-5.13609916331192,20.5219565910637));
#44136=CARTESIAN_POINT('Ctrl Pts',(18.6424403187525,-5.05696603051791,21.0440837186712));
#44137=CARTESIAN_POINT('Ctrl Pts',(18.6141397254773,-4.90035546598673,21.54183357279));
#44138=CARTESIAN_POINT('Ctrl Pts',(18.5678358953144,-4.64411811748906,22.356223733609));
#44139=CARTESIAN_POINT('Ctrl Pts',(18.5215320651515,-4.18047636719759,23.1053567774596));
#44140=CARTESIAN_POINT('Ctrl Pts',(18.4752282349886,-3.56590977309181,23.6979753851772));
#44141=CARTESIAN_POINT('Ctrl Pts',(18.4289244048258,-2.95134317898598,24.2905939928948));
#44142=CARTESIAN_POINT('Ctrl Pts',(18.3826205746629,-2.18585174106585,24.7266981644793));
#44143=CARTESIAN_POINT('Ctrl Pts',(18.3363167445,-1.36268551289881,24.9531628937623));
#44144=CARTESIAN_POINT('Ctrl Pts',(18.2900129143371,-0.539519284731791,
25.1796276230454));
#44145=CARTESIAN_POINT('Ctrl Pts',(18.2437090841742,0.341321733682111,25.196452910027));
#44146=CARTESIAN_POINT('Ctrl Pts',(18.1974052540114,1.17253592134146,25.0015891446991));
#44147=CARTESIAN_POINT('Ctrl Pts',(18.1511014238485,2.00375010900077,24.8067253793712));
#44148=CARTESIAN_POINT('Ctrl Pts',(18.1047975936856,2.78533746590556,24.4001725617338));
#44149=CARTESIAN_POINT('Ctrl Pts',(18.0584937635227,3.4220871780759,23.8314558336038));
#44150=CARTESIAN_POINT('Ctrl Pts',(18.0121899333599,4.05883689024629,23.2627391054738));
#44151=CARTESIAN_POINT('Ctrl Pts',(17.965886103197,4.55074895768223,22.5318584668512));
#44152=CARTESIAN_POINT('Ctrl Pts',(17.9195822730341,4.83790001041956,21.7278477792881));
#44153=CARTESIAN_POINT('Ctrl Pts',(17.8732784428712,5.12505106315689,20.9238370917249));
#44154=CARTESIAN_POINT('Ctrl Pts',(17.8269746127083,5.20744110119561,20.0466963552211));
#44155=CARTESIAN_POINT('Ctrl Pts',(17.7806707825455,5.07503359756761,19.2032764326517));
#44156=CARTESIAN_POINT('Ctrl Pts',(17.7343669523826,4.94262609393962,18.3598565100823));
#44157=CARTESIAN_POINT('Ctrl Pts',(17.6880631222197,4.59542104864494,17.5501574014474));
#44158=CARTESIAN_POINT('Ctrl Pts',(17.6417592920568,4.07571402172354,16.8728144167104));
#44159=CARTESIAN_POINT('Ctrl Pts',(17.595455461894,3.5560069948021,16.1954714319734));
#44160=CARTESIAN_POINT('Ctrl Pts',(17.5491516317311,2.8637979862539,15.6504845711344));
#44161=CARTESIAN_POINT('Ctrl Pts',(17.5028478015682,2.08340998642146,15.3042426289588));
#44162=CARTESIAN_POINT('Ctrl Pts',(17.4565439714053,1.30302198658901,14.9580006867833));
#44163=CARTESIAN_POINT('Ctrl Pts',(17.4102401412424,0.434454995472302,14.8105036632712));
#44164=CARTESIAN_POINT('Ctrl Pts',(17.3639363110796,-0.416484554045956,
14.8797192386111));
#44165=CARTESIAN_POINT('Ctrl Pts',(17.3176324809167,-1.26742410356419,14.9489348139509));
#44166=CARTESIAN_POINT('Ctrl Pts',(17.2713286507538,-2.10073621148394,15.2348629881427));
#44167=CARTESIAN_POINT('Ctrl Pts',(17.2250248205909,-2.81490909746055,15.7026727804085));
#44168=CARTESIAN_POINT('Ctrl Pts',(17.178720990428,-3.52908198343714,16.1704825726743));
#44169=CARTESIAN_POINT('Ctrl Pts',(17.1324171602652,-4.12411564747056,16.8201739830141));
#44170=CARTESIAN_POINT('Ctrl Pts',(17.0861133301023,-4.52752473140143,17.5726033975148));
#44171=CARTESIAN_POINT('Ctrl Pts',(17.0404227218359,-4.92559129220556,18.3150680598363));
#44172=CARTESIAN_POINT('Ctrl Pts',(16.9947321135695,-5.13707520056159,19.1575675366546));
#44173=CARTESIAN_POINT('Ctrl Pts',(16.9490415053031,-5.13718894078376,20.0000119941014));
#44174=CARTESIAN_POINT('Ctrl Pts',(17.4259584946968,-5.13631117261779,19.999995970574));
#44175=CARTESIAN_POINT('Ctrl Pts',(17.4488760716842,-5.1363227180941,19.577233171219));
#44176=CARTESIAN_POINT('Ctrl Pts',(17.4717936486717,-5.08471936726895,19.1544731410777));
#44177=CARTESIAN_POINT('Ctrl Pts',(17.4947112256591,-4.9814682768752,18.7447277425743));
#44178=CARTESIAN_POINT('Ctrl Pts',(17.5410150558219,-4.7728545584027,17.9168574422915));
#44179=CARTESIAN_POINT('Ctrl Pts',(17.5873188859848,-4.3534033904449,17.1421157351172));
#44180=CARTESIAN_POINT('Ctrl Pts',(17.6336227161477,-3.77421115624452,16.5148795168809));
#44181=CARTESIAN_POINT('Ctrl Pts',(17.6799265463106,-3.19501892204413,15.8876432986447));
#44182=CARTESIAN_POINT('Ctrl Pts',(17.7262303764735,-2.45608562160116,15.4079125693465));
#44183=CARTESIAN_POINT('Ctrl Pts',(17.7725342066363,-1.6474260694984,15.1341268019693));
#44184=CARTESIAN_POINT('Ctrl Pts',(17.8188380367992,-0.838766517395638,
14.8603410345921));
#44185=CARTESIAN_POINT('Ctrl Pts',(17.8651418669621,0.0396192863669109,
14.7925002291359));
#44186=CARTESIAN_POINT('Ctrl Pts',(17.911445697125,0.880728808258228,14.9388685652237));
#44187=CARTESIAN_POINT('Ctrl Pts',(17.9577495272879,1.72183833014957,15.0852369013115));
#44188=CARTESIAN_POINT('Ctrl Pts',(18.0040533574507,2.52567157016968,15.4458143789434));
#44189=CARTESIAN_POINT('Ctrl Pts',(18.0503571876136,3.19430778227486,15.9766764452912));
#44190=CARTESIAN_POINT('Ctrl Pts',(18.0966610177765,3.86294399438003,16.5075385116389));
#44191=CARTESIAN_POINT('Ctrl Pts',(18.1429648479394,4.39638317857029,17.2086851667026));
#44192=CARTESIAN_POINT('Ctrl Pts',(18.1892686781023,4.72964324616823,17.9947046607166));
#44193=CARTESIAN_POINT('Ctrl Pts',(18.2355725082651,5.06290331376618,18.7807241547306));
#44194=CARTESIAN_POINT('Ctrl Pts',(18.281876338428,5.19598426477179,19.6516164876949));
#44195=CARTESIAN_POINT('Ctrl Pts',(18.3281801685909,5.11267454514886,20.5012919600029));
#44196=CARTESIAN_POINT('Ctrl Pts',(18.3744839987538,5.02936482552594,21.3509674323108));
#44197=CARTESIAN_POINT('Ctrl Pts',(18.4207878289167,4.72966443527452,22.1794260439624));
#44198=CARTESIAN_POINT('Ctrl Pts',(18.4670916590795,4.25008204850996,22.8857472541285));
#44199=CARTESIAN_POINT('Ctrl Pts',(18.5133954892424,3.77049966174541,23.5920684642946));
#44200=CARTESIAN_POINT('Ctrl Pts',(18.5596993194053,3.11103527846767,24.1762522729753));
#44201=CARTESIAN_POINT('Ctrl Pts',(18.6060031495682,2.35202302917159,24.5671350214355));
#44202=CARTESIAN_POINT('Ctrl Pts',(18.652306979731,1.59301077987547,24.9580177698958));
#44203=CARTESIAN_POINT('Ctrl Pts',(18.6986108098939,0.734450664561022,25.1555994581356));
#44204=CARTESIAN_POINT('Ctrl Pts',(18.7449146400568,-0.119069893872046,
25.1358112303851));
#44205=CARTESIAN_POINT('Ctrl Pts',(18.7912184702197,-0.972590452305114,
25.1160230026347));
#44206=CARTESIAN_POINT('Ctrl Pts',(18.8375223003826,-1.82107145385673,24.8788648588939));
#44207=CARTESIAN_POINT('Ctrl Pts',(18.8838261305454,-2.5611532854388,24.4532267494776));
#44208=CARTESIAN_POINT('Ctrl Pts',(18.9301299607083,-3.30123511702085,24.0275886400612));
#44209=CARTESIAN_POINT('Ctrl Pts',(18.9764337908712,-3.93291777863336,23.4134705649693));
#44210=CARTESIAN_POINT('Ctrl Pts',(19.0227376210341,-4.37925143241393,22.6856826926272));
#44211=CARTESIAN_POINT('Ctrl Pts',(19.069041451197,-4.82558508619451,21.9578948202851));
#44212=CARTESIAN_POINT('Ctrl Pts',(19.1153452813598,-5.08656973214315,21.1164371506928));
#44213=CARTESIAN_POINT('Ctrl Pts',(19.1616491115227,-5.13041294122744,20.2638137340296));
#44214=CARTESIAN_POINT('Ctrl Pts',(19.1664189059141,-5.13492926508348,20.1759843174035));
#44215=CARTESIAN_POINT('Ctrl Pts',(19.1711887003055,-5.13714145250432,20.0880364185337));
#44216=CARTESIAN_POINT('Ctrl Pts',(19.1759584946968,-5.13707257898892,20.0000850551338));
#44217=CARTESIAN_POINT('Origin',(25.,0.,20.));
#44218=CARTESIAN_POINT('',(20.9259584946969,-5.13657443916938,19.9998752094656));
#44219=CARTESIAN_POINT('',(20.4490415053031,-5.13680856920626,20.000130812524));
#44220=CARTESIAN_POINT('',(25.,-5.13675,20.));
#44221=CARTESIAN_POINT('Ctrl Pts',(20.4490415053031,-5.13680856920626,20.000130812524));
#44222=CARTESIAN_POINT('Ctrl Pts',(20.4393573708119,-5.13699294951738,20.1787253578794));
#44223=CARTESIAN_POINT('Ctrl Pts',(20.4296732363207,-5.12786043275759,20.3573011391577));
#44224=CARTESIAN_POINT('Ctrl Pts',(20.4199891018296,-5.10926909616917,20.5348866815868));
#44225=CARTESIAN_POINT('Ctrl Pts',(20.3736852716667,-5.02037626917714,21.3839962022691));
#44226=CARTESIAN_POINT('Ctrl Pts',(20.3273814415038,-4.71523690500024,22.2104669872532));
#44227=CARTESIAN_POINT('Ctrl Pts',(20.2810776113409,-4.23102223854131,22.9136206472664));
#44228=CARTESIAN_POINT('Ctrl Pts',(20.234773781178,-3.74680757208241,23.6167743072796));
#44229=CARTESIAN_POINT('Ctrl Pts',(20.1884699510152,-3.08351760334145,24.1966108423221));
#44230=CARTESIAN_POINT('Ctrl Pts',(20.1421661208523,-2.32195248507256,24.5824961665313));
#44231=CARTESIAN_POINT('Ctrl Pts',(20.0958622906894,-1.56038736680363,24.9683814907404));
#44232=CARTESIAN_POINT('Ctrl Pts',(20.0495584605265,-0.700547099006791,
25.1603156041162));
#44233=CARTESIAN_POINT('Ctrl Pts',(20.0032546303637,0.152824950777143,25.1349176228668));
#44234=CARTESIAN_POINT('Ctrl Pts',(19.9569508002008,1.00619700056105,25.1095196416174));
#44235=CARTESIAN_POINT('Ctrl Pts',(19.9106469700379,1.85310083233197,24.8667895657428));
#44236=CARTESIAN_POINT('Ctrl Pts',(19.864343139875,2.59036895947021,24.4362961029469));
#44237=CARTESIAN_POINT('Ctrl Pts',(19.8180393097121,3.32763708660844,24.0058026401509));
#44238=CARTESIAN_POINT('Ctrl Pts',(19.7717354795493,3.95526950911397,23.3875457904338));
#44239=CARTESIAN_POINT('Ctrl Pts',(19.7254316493864,4.39680977807037,22.6568398963191));
#44240=CARTESIAN_POINT('Ctrl Pts',(19.6791278192235,4.83835004702677,21.9261340022045));
#44241=CARTESIAN_POINT('Ctrl Pts',(19.6328239890606,5.09379816243402,21.0829790636924));
#44242=CARTESIAN_POINT('Ctrl Pts',(19.5865201588977,5.13203614012476,20.2300858875759));
#44243=CARTESIAN_POINT('Ctrl Pts',(19.5402163287349,5.17027411781551,19.3771927114594));
#44244=CARTESIAN_POINT('Ctrl Pts',(19.493912498572,4.99130195778974,18.5145612977385));
#44245=CARTESIAN_POINT('Ctrl Pts',(19.4476086684091,4.6169215544682,17.7472750236447));
#44246=CARTESIAN_POINT('Ctrl Pts',(19.4013048382462,4.24254115114665,16.9799887495508));
#44247=CARTESIAN_POINT('Ctrl Pts',(19.3550010080833,3.67275250452931,16.3080476150841));
#44248=CARTESIAN_POINT('Ctrl Pts',(19.3086971779205,2.97696569445138,15.8133056341228));
#44249=CARTESIAN_POINT('Ctrl Pts',(19.2623933477576,2.28117888437348,15.3185636531615));
#44250=CARTESIAN_POINT('Ctrl Pts',(19.2160895175947,1.45939391083502,15.0010208257055));
#44251=CARTESIAN_POINT('Ctrl Pts',(19.1697856874318,0.611718350494981,14.8993593423104));
#44252=CARTESIAN_POINT('Ctrl Pts',(19.123481857269,-0.235957209845108,14.7976978589153));
#44253=CARTESIAN_POINT('Ctrl Pts',(19.0771780271061,-1.10952335698676,14.9119177195811));
#44254=CARTESIAN_POINT('Ctrl Pts',(19.0308741969432,-1.90256467466223,15.2281049762243));
#44255=CARTESIAN_POINT('Ctrl Pts',(18.9845703667803,-2.69560599233769,15.5442922328674));
#44256=CARTESIAN_POINT('Ctrl Pts',(18.9382665366174,-3.40812248054695,16.0624468854881));
#44257=CARTESIAN_POINT('Ctrl Pts',(18.8919627064546,-3.95331734784091,16.7194487648463));
#44258=CARTESIAN_POINT('Ctrl Pts',(18.8456588762917,-4.49851221513488,17.3764506442046));
#44259=CARTESIAN_POINT('Ctrl Pts',(18.7993550461288,-4.87638546151354,18.1722997503005));
#44260=CARTESIAN_POINT('Ctrl Pts',(18.7530512159659,-5.04090561135092,19.0100479422421));
#44261=CARTESIAN_POINT('Ctrl Pts',(18.7350479790783,-5.10487213895543,19.3357700066727));
#44262=CARTESIAN_POINT('Ctrl Pts',(18.7170447421907,-5.13658594929633,19.6678259813736));
#44263=CARTESIAN_POINT('Ctrl Pts',(18.6990415053031,-5.13639668367057,19.9999176386971));
#44264=CARTESIAN_POINT('Ctrl Pts',(19.1759584946968,-5.13707257898892,20.0000850551338));
#44265=CARTESIAN_POINT('Ctrl Pts',(19.2174925304683,-5.13647284767606,19.2342291766898));
#44266=CARTESIAN_POINT('Ctrl Pts',(19.2590265662398,-4.96291305319095,18.4681106023481));
#44267=CARTESIAN_POINT('Ctrl Pts',(19.3005606020113,-4.63162896954659,17.7776706539684));
#44268=CARTESIAN_POINT('Ctrl Pts',(19.3468644321742,-4.26230001656154,17.0079401543048));
#44269=CARTESIAN_POINT('Ctrl Pts',(19.3931682623371,-3.69694033837151,16.332268318712));
#44270=CARTESIAN_POINT('Ctrl Pts',(19.4394720925,-3.00442049010556,15.8329636247795));
#44271=CARTESIAN_POINT('Ctrl Pts',(19.4857759226629,-2.31190064183958,15.333658930847));
#44272=CARTESIAN_POINT('Ctrl Pts',(19.5320797528257,-1.49222062349769,15.0107213785748));
#44273=CARTESIAN_POINT('Ctrl Pts',(19.5783835829886,-0.645231591908269,
14.9034903290016));
#44274=CARTESIAN_POINT('Ctrl Pts',(19.6246874131515,0.20175743968115,14.7962592794284));
#44275=CARTESIAN_POINT('Ctrl Pts',(19.6709912433144,1.07605548451817,14.9047347325541));
#44276=CARTESIAN_POINT('Ctrl Pts',(19.7172950734773,1.87115796857826,15.2157025081625));
#44277=CARTESIAN_POINT('Ctrl Pts',(19.7635989036401,2.66626045263838,15.5266702837709));
#44278=CARTESIAN_POINT('Ctrl Pts',(19.809902733803,3.38216737592161,16.0401303818618));
#44279=CARTESIAN_POINT('Ctrl Pts',(19.8562065639659,3.93166893353869,16.6935345108676));
#44280=CARTESIAN_POINT('Ctrl Pts',(19.9025103941288,4.48117049115577,17.3469386398734));
#44281=CARTESIAN_POINT('Ctrl Pts',(19.9488142242917,4.86426668310665,18.1402867997939));
#44282=CARTESIAN_POINT('Ctrl Pts',(19.9951180544545,5.03428978895545,18.9769355080957));
#44283=CARTESIAN_POINT('Ctrl Pts',(20.0414218846174,5.20431289480425,19.8135842163973));
#44284=CARTESIAN_POINT('Ctrl Pts',(20.0877257147803,5.16126291455098,20.6935334730801));
#44285=CARTESIAN_POINT('Ctrl Pts',(20.1340295449432,4.91038407793598,21.5095902890948));
#44286=CARTESIAN_POINT('Ctrl Pts',(20.180333375106,4.65950524132096,22.3256471051096));
#44287=CARTESIAN_POINT('Ctrl Pts',(20.2266372052689,4.20079754834418,23.0778114804561));
#44288=CARTESIAN_POINT('Ctrl Pts',(20.2729410354318,3.59013950374517,23.6744568275359));
#44289=CARTESIAN_POINT('Ctrl Pts',(20.3192448655947,2.97948145914616,24.2711021746156));
#44290=CARTESIAN_POINT('Ctrl Pts',(20.3655486957576,2.21687306292492,24.7122284934286));
#44291=CARTESIAN_POINT('Ctrl Pts',(20.4118525259204,1.39521316446878,24.9440989936964));
#44292=CARTESIAN_POINT('Ctrl Pts',(20.4581563560833,0.57355326601265,25.1759694939642));
#44293=CARTESIAN_POINT('Ctrl Pts',(20.5044601862462,-0.307158134678377,
25.198584175687));
#44294=CARTESIAN_POINT('Ctrl Pts',(20.5507640164091,-1.13963520627605,25.0091881807727));
#44295=CARTESIAN_POINT('Ctrl Pts',(20.5970678465719,-1.97211227787367,24.8197921858584));
#44296=CARTESIAN_POINT('Ctrl Pts',(20.6433716767348,-2.75635502037793,24.4183855143072));
#44297=CARTESIAN_POINT('Ctrl Pts',(20.6896755068977,-3.39682914806631,23.8538664186274));
#44298=CARTESIAN_POINT('Ctrl Pts',(20.7359793370606,-4.03730327575471,23.2893473229476));
#44299=CARTESIAN_POINT('Ctrl Pts',(20.7822831672235,-4.53400878862721,22.5617158031392));
#44300=CARTESIAN_POINT('Ctrl Pts',(20.8285869973863,-4.82643839243051,21.7596099220706));
#44301=CARTESIAN_POINT('Ctrl Pts',(20.8610441631565,-5.03142005579099,21.1973652123891));
#44302=CARTESIAN_POINT('Ctrl Pts',(20.8935013289267,-5.13603158465629,20.5985278291506));
#44303=CARTESIAN_POINT('Ctrl Pts',(20.9259584946969,-5.13657443916938,19.9998752094656));
#44304=CARTESIAN_POINT('Origin',(25.,0.,20.));
#44305=CARTESIAN_POINT('',(22.6759584946968,-5.1365747461539,20.0001248276021));
#44306=CARTESIAN_POINT('',(22.1990415053031,-5.13685244596756,19.9998725425992));
#44307=CARTESIAN_POINT('',(25.,-5.13675,20.));
#44308=CARTESIAN_POINT('Ctrl Pts',(22.1990415053031,-5.13685244596756,19.9998725425992));
#44309=CARTESIAN_POINT('Ctrl Pts',(22.1616699994331,-5.13614579389918,20.6890598759674));
#44310=CARTESIAN_POINT('Ctrl Pts',(22.1242984935631,-4.99651893549095,21.3785248624566));
#44311=CARTESIAN_POINT('Ctrl Pts',(22.0869269876932,-4.72657997268596,22.012504961736));
#44312=CARTESIAN_POINT('Ctrl Pts',(22.0406231575303,-4.39212173780621,22.7980153702763));
#44313=CARTESIAN_POINT('Ctrl Pts',(21.9943193273674,-3.85761403741936,23.4983477972205));
#44314=CARTESIAN_POINT('Ctrl Pts',(21.9480154972046,-3.18816912389587,24.0281896798246));
#44315=CARTESIAN_POINT('Ctrl Pts',(21.9017116670417,-2.51872421037239,24.5580315624287));
#44316=CARTESIAN_POINT('Ctrl Pts',(21.8554078368788,-1.71434208371228,24.9173829006927));
#44317=CARTESIAN_POINT('Ctrl Pts',(21.8091040067159,-0.87301035381432,25.0624685067012));
#44318=CARTESIAN_POINT('Ctrl Pts',(21.762800176553,-0.031678623916381,25.2075541127096));
#44319=CARTESIAN_POINT('Ctrl Pts',(21.7164963463902,0.846602709219399,25.1383739864625));
#44320=CARTESIAN_POINT('Ctrl Pts',(21.6701925162273,1.65484383838534,24.8633554599439));
#44321=CARTESIAN_POINT('Ctrl Pts',(21.6238886860644,2.46308496755134,24.5883369334253));
#44322=CARTESIAN_POINT('Ctrl Pts',(21.5775848559015,3.20128589274747,24.1074800066352));
#44323=CARTESIAN_POINT('Ctrl Pts',(21.5312810257386,3.77952101532157,23.4793613428259));
#44324=CARTESIAN_POINT('Ctrl Pts',(21.4849771955758,4.35775613789566,22.8512426790165));
#44325=CARTESIAN_POINT('Ctrl Pts',(21.4386733654129,4.77602545784771,22.0758622781877));
#44326=CARTESIAN_POINT('Ctrl Pts',(21.39236953525,4.98337656139613,21.2476748400669));
#44327=CARTESIAN_POINT('Ctrl Pts',(21.3460657050871,5.19072766494455,20.419487401946));
#44328=CARTESIAN_POINT('Ctrl Pts',(21.2997618749242,5.18716055208937,19.538492926533));
#44329=CARTESIAN_POINT('Ctrl Pts',(21.2534580447614,4.97310975867039,18.7120117285372));
#44330=CARTESIAN_POINT('Ctrl Pts',(21.2071542145985,4.75905896525139,17.8855305305414));
#44331=CARTESIAN_POINT('Ctrl Pts',(21.1608503844356,4.33452449126856,17.1135626099627));
#44332=CARTESIAN_POINT('Ctrl Pts',(21.1145465542728,3.7512219542704,16.4901469676056));
#44333=CARTESIAN_POINT('Ctrl Pts',(21.0682427241099,3.16791941727224,15.8667313252485));
#44334=CARTESIAN_POINT('Ctrl Pts',(21.021938893947,2.42584881725878,15.391867961113));
#44335=CARTESIAN_POINT('Ctrl Pts',(20.9756350637841,1.61540714598487,15.123403419196));
#44336=CARTESIAN_POINT('Ctrl Pts',(20.9293312336212,0.804965474710955,14.8549388772789));
#44337=CARTESIAN_POINT('Ctrl Pts',(20.8830274034583,-0.0738472678233812,
14.7928731575803));
#44338=CARTESIAN_POINT('Ctrl Pts',(20.8367235732955,-0.913976539584659,
14.9447669347203));
#44339=CARTESIAN_POINT('Ctrl Pts',(20.7904197431326,-1.75410581134589,15.0966607118603));
#44340=CARTESIAN_POINT('Ctrl Pts',(20.7441159129697,-2.55555161233405,15.4625139858388));
#44341=CARTESIAN_POINT('Ctrl Pts',(20.6978120828068,-3.22068402773702,15.9977595208823));
#44342=CARTESIAN_POINT('Ctrl Pts',(20.6515082526439,-3.88581644314001,16.533005055926));
#44343=CARTESIAN_POINT('Ctrl Pts',(20.6052044224811,-4.41463547295778,17.2376428520347));
#44344=CARTESIAN_POINT('Ctrl Pts',(20.5589005923182,-4.74272184296308,18.0258358782793));
#44345=CARTESIAN_POINT('Ctrl Pts',(20.5222808966465,-5.00219115643817,18.6491836369876));
#44346=CARTESIAN_POINT('Ctrl Pts',(20.4856612009748,-5.13611135141281,19.3247913791957));
#44347=CARTESIAN_POINT('Ctrl Pts',(20.4490415053031,-5.13680856920626,20.000130812524));
#44348=CARTESIAN_POINT('Ctrl Pts',(20.9259584946969,-5.13657443916938,19.9998752094656));
#44349=CARTESIAN_POINT('Ctrl Pts',(20.9398051590896,-5.13680602822155,19.7444819329456));
#44350=CARTESIAN_POINT('Ctrl Pts',(20.9536518234823,-5.11809721635881,19.4891222832186));
#44351=CARTESIAN_POINT('Ctrl Pts',(20.967498487875,-5.08016083691862,19.2366517801062));
#44352=CARTESIAN_POINT('Ctrl Pts',(21.0138023180379,-4.95329998286932,18.3923797615392));
#44353=CARTESIAN_POINT('Ctrl Pts',(21.0601061482008,-4.61142458003661,17.5804159667339));
#44354=CARTESIAN_POINT('Ctrl Pts',(21.1064099783636,-4.09618094613004,16.8996715834709));
#44355=CARTESIAN_POINT('Ctrl Pts',(21.1527138085265,-3.58093731222347,16.2189272002079));
#44356=CARTESIAN_POINT('Ctrl Pts',(21.1990176386894,-2.89232544724305,15.6694022284871));
#44357=CARTESIAN_POINT('Ctrl Pts',(21.2453214688522,-2.11423014743298,15.3180382832127));
#44358=CARTESIAN_POINT('Ctrl Pts',(21.2916252990151,-1.3361348476229,14.9666743379382));
#44359=CARTESIAN_POINT('Ctrl Pts',(21.337929129178,-0.468556112983181,14.8134714191101));
#44360=CARTESIAN_POINT('Ctrl Pts',(21.3842329593409,0.382820010279116,14.877092283331));
#44361=CARTESIAN_POINT('Ctrl Pts',(21.4305367895038,1.23419613354144,14.940713147552));
#44362=CARTESIAN_POINT('Ctrl Pts',(21.4768406196667,2.06936964542633,15.221157794822));
#44363=CARTESIAN_POINT('Ctrl Pts',(21.5231444498295,2.78660201449705,15.6842632324738));
#44364=CARTESIAN_POINT('Ctrl Pts',(21.5694482799924,3.50383438356776,16.1473686701255));
#44365=CARTESIAN_POINT('Ctrl Pts',(21.6157521101553,4.10312560982429,16.7931348981589));
#44366=CARTESIAN_POINT('Ctrl Pts',(21.6620559403182,4.51147169063172,17.5428964575327));
#44367=CARTESIAN_POINT('Ctrl Pts',(21.708359770481,4.91981777143912,18.2926580169065));
#44368=CARTESIAN_POINT('Ctrl Pts',(21.7546636006439,5.13721870679744,19.1464149076206));
#44369=CARTESIAN_POINT('Ctrl Pts',(21.8009674308068,5.13719131497069,20.0001648223351));
#44370=CARTESIAN_POINT('Ctrl Pts',(21.8472712609697,5.13716392314393,20.8539147370496));
#44371=CARTESIAN_POINT('Ctrl Pts',(21.8935750911326,4.91970820413208,21.7076576757646));
#44372=CARTESIAN_POINT('Ctrl Pts',(21.9398789212954,4.51131401326454,22.4573930307339));
#44373=CARTESIAN_POINT('Ctrl Pts',(21.9861827514583,4.10291982239703,23.2071283857032));
#44374=CARTESIAN_POINT('Ctrl Pts',(22.0324865816212,3.50358715967385,23.852856156927));
#44375=CARTESIAN_POINT('Ctrl Pts',(22.0787904117841,2.7863250754059,24.3159155700663));
#44376=CARTESIAN_POINT('Ctrl Pts',(22.125094241947,2.06906299113791,24.7789749832056));
#44377=CARTESIAN_POINT('Ctrl Pts',(22.1713980721098,1.23387148532514,25.0593660382605));
#44378=CARTESIAN_POINT('Ctrl Pts',(22.2177019022727,0.382491281374938,25.1229322710191));
#44379=CARTESIAN_POINT('Ctrl Pts',(22.2640057324356,-0.468888922575259,
25.1864985037777));
#44380=CARTESIAN_POINT('Ctrl Pts',(22.3103095625985,-1.33645782466288,25.0332399142401));
#44381=CARTESIAN_POINT('Ctrl Pts',(22.3566133927614,-2.11453057645518,24.6818260406611));
#44382=CARTESIAN_POINT('Ctrl Pts',(22.4029172229242,-2.89260332824749,24.3304121670822));
#44383=CARTESIAN_POINT('Ctrl Pts',(22.4492210530871,-3.58117992974448,23.780843009462));
#44384=CARTESIAN_POINT('Ctrl Pts',(22.49552488325,-4.09637988040214,23.1000655653088));
#44385=CARTESIAN_POINT('Ctrl Pts',(22.5418287134129,-4.61157983105977,22.4192881211556));
#44386=CARTESIAN_POINT('Ctrl Pts',(22.5881325435757,-4.95340313087809,21.6073023904696));
#44387=CARTESIAN_POINT('Ctrl Pts',(22.6344363737386,-5.08020980919293,20.7630222331994));
#44388=CARTESIAN_POINT('Ctrl Pts',(22.6482770807247,-5.11811367313376,20.510657920575));
#44389=CARTESIAN_POINT('Ctrl Pts',(22.6621177877108,-5.13680632573211,20.2554081796058));
#44390=CARTESIAN_POINT('Ctrl Pts',(22.6759584946968,-5.1365747461539,20.0001248276021));
#44391=CARTESIAN_POINT('Origin',(25.,0.,20.));
#44392=CARTESIAN_POINT('',(24.4259584946968,-5.13707231536035,19.9999148579252));
#44393=CARTESIAN_POINT('',(23.9490415053031,-5.13637392180183,20.0000717483683));
#44394=CARTESIAN_POINT('',(25.,-5.13675,20.));
#44395=CARTESIAN_POINT('Ctrl Pts',(23.9490415053031,-5.13637392180183,20.0000717483683));
#44396=CARTESIAN_POINT('Ctrl Pts',(23.9302864582172,-5.13654471386954,20.3460358505988));
#44397=CARTESIAN_POINT('Ctrl Pts',(23.9115314111314,-5.10210725044954,20.6919664138276));
#44398=CARTESIAN_POINT('Ctrl Pts',(23.8927763640455,-5.03272390749879,21.0307397974748));
#44399=CARTESIAN_POINT('Ctrl Pts',(23.8464725338826,-4.86142524248265,21.8671282719098));
#44400=CARTESIAN_POINT('Ctrl Pts',(23.8001687037197,-4.47711976629267,22.6598913455785));
#44401=CARTESIAN_POINT('Ctrl Pts',(23.7538648735568,-3.9266225110321,23.3124568095394));
#44402=CARTESIAN_POINT('Ctrl Pts',(23.7075610433939,-3.37612525577151,23.9650222735004));
#44403=CARTESIAN_POINT('Ctrl Pts',(23.6612572132311,-2.65943622144031,24.4773901277534));
#44404=CARTESIAN_POINT('Ctrl Pts',(23.6149533830682,-1.86386048753644,24.7871451348595));
#44405=CARTESIAN_POINT('Ctrl Pts',(23.5686495529053,-1.06828475363257,25.0969001419655));
#44406=CARTESIAN_POINT('Ctrl Pts',(23.5223457227424,-0.193822320156021,
25.2040423019247));
#44407=CARTESIAN_POINT('Ctrl Pts',(23.4760418925795,0.65300221349861,25.0955198526131));
#44408=CARTESIAN_POINT('Ctrl Pts',(23.4297380624166,1.49982674715322,24.9869974033015));
#44409=CARTESIAN_POINT('Ctrl Pts',(23.3834342322538,2.31901338098592,24.6628103447192));
#44410=CARTESIAN_POINT('Ctrl Pts',(23.3371304020909,3.01077106090705,24.1624502493138));
#44411=CARTESIAN_POINT('Ctrl Pts',(23.2908265719281,3.7025287408282,23.6620901539085));
#44412=CARTESIAN_POINT('Ctrl Pts',(23.2445227417652,4.26685746683774,22.9855570216801));
#44413=CARTESIAN_POINT('Ctrl Pts',(23.1982189116023,4.63501227155502,22.2152642509964));
#44414=CARTESIAN_POINT('Ctrl Pts',(23.1519150814394,5.00316707627228,21.4449714803128));
#44415=CARTESIAN_POINT('Ctrl Pts',(23.1056112512765,5.17514795969726,20.5809190711738));
#44416=CARTESIAN_POINT('Ctrl Pts',(23.0593074211136,5.13000468542294,19.7283635025498));
#44417=CARTESIAN_POINT('Ctrl Pts',(23.0130035909508,5.08486141114861,18.8758079339259));
#44418=CARTESIAN_POINT('Ctrl Pts',(22.9666997607879,4.822593979175,18.0347492058169));
#44419=CARTESIAN_POINT('Ctrl Pts',(22.920395930625,4.37515108398647,17.3076427704518));
#44420=CARTESIAN_POINT('Ctrl Pts',(22.8740921004621,3.92770818879797,16.5805363350868));
#44421=CARTESIAN_POINT('Ctrl Pts',(22.8277882702993,3.2950898303946,15.9673821924658));
#44422=CARTESIAN_POINT('Ctrl Pts',(22.7814844401364,2.55435983063849,15.5428730874218));
#44423=CARTESIAN_POINT('Ctrl Pts',(22.7351806099735,1.81362983088237,15.1183639823779));
#44424=CARTESIAN_POINT('Ctrl Pts',(22.6888767798106,0.964788189773507,14.882499914911));
#44425=CARTESIAN_POINT('Ctrl Pts',(22.6425729496478,0.11123845251519,14.864013194537));
#44426=CARTESIAN_POINT('Ctrl Pts',(22.5962691194849,-0.742311284743175,
14.8455264741629));
#44427=CARTESIAN_POINT('Ctrl Pts',(22.549965289322,-1.60056911815101,15.0444171008817));
#44428=CARTESIAN_POINT('Ctrl Pts',(22.5036614591591,-2.35898444795574,15.4364567676518));
#44429=CARTESIAN_POINT('Ctrl Pts',(22.4573576289962,-3.11739977776043,15.8284964344218));
#44430=CARTESIAN_POINT('Ctrl Pts',(22.4110537988333,-3.77597260396205,16.4136851412431));
#44431=CARTESIAN_POINT('Ctrl Pts',(22.3647499686705,-4.25447740308742,17.1207368154636));
#44432=CARTESIAN_POINT('Ctrl Pts',(22.3184461385076,-4.73298220221278,17.827788489684));
#44433=CARTESIAN_POINT('Ctrl Pts',(22.2721423083447,-5.0314189742619,18.6567031313036));
#44434=CARTESIAN_POINT('Ctrl Pts',(22.2258384781818,-5.11343297560014,19.5065046471815));
#44435=CARTESIAN_POINT('Ctrl Pts',(22.2169061538889,-5.12925403519577,19.6704371490444));
#44436=CARTESIAN_POINT('Ctrl Pts',(22.207973829596,-5.1370213459166,19.8351469149609));
#44437=CARTESIAN_POINT('Ctrl Pts',(22.1990415053031,-5.13685244596756,19.9998725425992));
#44438=CARTESIAN_POINT('Ctrl Pts',(22.6759584946968,-5.1365747461539,20.0001248276021));
#44439=CARTESIAN_POINT('Ctrl Pts',(22.7084216178736,-5.13603158052079,19.4013624298848));
#44440=CARTESIAN_POINT('Ctrl Pts',(22.7408847410504,-5.03138084291631,18.802415128328));
#44441=CARTESIAN_POINT('Ctrl Pts',(22.7733478642272,-4.82632547137258,18.240080377359));
#44442=CARTESIAN_POINT('Ctrl Pts',(22.8196516943901,-4.53384439842607,17.437993262643));
#44443=CARTESIAN_POINT('Ctrl Pts',(22.865955524553,-4.0370921957217,16.7103936170653));
#44444=CARTESIAN_POINT('Ctrl Pts',(22.9122593547159,-3.39658184513919,16.1459156206632));
#44445=CARTESIAN_POINT('Ctrl Pts',(22.9585631848788,-2.75607149455666,15.5814376242612));
#44446=CARTESIAN_POINT('Ctrl Pts',(23.0048670150417,-1.97180299609605,15.180081277035));
#44447=CARTESIAN_POINT('Ctrl Pts',(23.0511708452045,-1.13931377299928,14.9907387011226));
#44448=CARTESIAN_POINT('Ctrl Pts',(23.0974746753674,-0.306824549902529,
14.8013961252102));
#44449=CARTESIAN_POINT('Ctrl Pts',(23.1437785055303,0.57388539783039,14.8240673206118));
#44450=CARTESIAN_POINT('Ctrl Pts',(23.1900823356932,1.39553041586644,15.0559905448949));
#44451=CARTESIAN_POINT('Ctrl Pts',(23.236386165856,2.21717543390246,15.2879137691781));
#44452=CARTESIAN_POINT('Ctrl Pts',(23.2826899960189,2.9797555222417,15.7290890223429));
#44453=CARTESIAN_POINT('Ctrl Pts',(23.3289938261818,3.59037527988484,16.3257735530634));
#44454=CARTESIAN_POINT('Ctrl Pts',(23.3752976563447,4.20099503752802,16.9224580837839));
#44455=CARTESIAN_POINT('Ctrl Pts',(23.4216014865076,4.6596544644751,17.6746518920602));
#44456=CARTESIAN_POINT('Ctrl Pts',(23.4679053166704,4.91048093562102,18.4907248048553));
#44457=CARTESIAN_POINT('Ctrl Pts',(23.5142091468333,5.16130740676694,19.3067977176504));
#44458=CARTESIAN_POINT('Ctrl Pts',(23.5605129769962,5.20430092211171,20.1867497349642));
#44459=CARTESIAN_POINT('Ctrl Pts',(23.6068168071591,5.0342241303143,21.0233875314552));
#44460=CARTESIAN_POINT('Ctrl Pts',(23.653120637322,4.86414733851688,21.8600253279462));
#44461=CARTESIAN_POINT('Ctrl Pts',(23.6994244674848,4.48100023957725,22.6533489036142));
#44462=CARTESIAN_POINT('Ctrl Pts',(23.7457282976477,3.93145675528012,23.3067177707115));
#44463=CARTESIAN_POINT('Ctrl Pts',(23.7920321278106,3.38191327098302,23.9600866378087));
#44464=CARTESIAN_POINT('Ctrl Pts',(23.8383359579735,2.66597340132842,24.4735007963352));
#44465=CARTESIAN_POINT('Ctrl Pts',(23.8846397881363,1.87085096464169,24.7844175509539));
#44466=CARTESIAN_POINT('Ctrl Pts',(23.9309436182992,1.07572852795493,25.0953343055727));
#44467=CARTESIAN_POINT('Ctrl Pts',(23.9772474484621,0.201423524236018,25.2037536562837));
#44468=CARTESIAN_POINT('Ctrl Pts',(24.023551278625,-0.645558624778892,25.096468257112));
#44469=CARTESIAN_POINT('Ctrl Pts',(24.0698551087879,-1.49254077379385,24.9891828579403));
#44470=CARTESIAN_POINT('Ctrl Pts',(24.1161589389507,-2.31220006810482,24.6661927088857));
#44471=CARTESIAN_POINT('Ctrl Pts',(24.1624627691136,-3.00468787542759,24.1668435781818));
#44472=CARTESIAN_POINT('Ctrl Pts',(24.2087665992765,-3.69717568275031,23.667494447478));
#44473=CARTESIAN_POINT('Ctrl Pts',(24.2550704294394,-4.26249200308487,22.9917863351248));
#44474=CARTESIAN_POINT('Ctrl Pts',(24.3013742596023,-4.63177156303645,22.2220321378467));
#44475=CARTESIAN_POINT('Ctrl Pts',(24.3429023379671,-4.96296383050694,21.5316699688036));
#44476=CARTESIAN_POINT('Ctrl Pts',(24.384430416332,-5.13647219728032,20.7656610002149));
#44477=CARTESIAN_POINT('Ctrl Pts',(24.4259584946968,-5.13707231536035,19.9999148579252));
#44478=CARTESIAN_POINT('Origin',(25.,0.,20.));
#44479=CARTESIAN_POINT('',(26.1759584946969,-5.13631118199777,20.0000041318326));
#44480=CARTESIAN_POINT('',(25.6990415053031,-5.13719123497192,20.0000027154119));
#44481=CARTESIAN_POINT('',(25.,-5.13675,20.));
#44482=CARTESIAN_POINT('Ctrl Pts',(25.6990415053031,-5.1371911776762,20.0000027150593));
#44483=CARTESIAN_POINT('Ctrl Pts',(25.6525990868384,-5.13721811325437,20.8563079779957));
#44484=CARTESIAN_POINT('Ctrl Pts',(25.6061566683738,-4.9184342166288,21.71259975382));
#44485=CARTESIAN_POINT('Ctrl Pts',(25.5597142499091,-4.50771973522286,22.4639799609353));
#44486=CARTESIAN_POINT('Ctrl Pts',(25.5134104197462,-4.09823086230967,23.2131179827739));
#44487=CARTESIAN_POINT('Ctrl Pts',(25.4671065895833,-3.49795564305339,23.8579696332713));
#44488=CARTESIAN_POINT('Ctrl Pts',(25.4208027594205,-2.78001794739953,24.3199808646966));
#44489=CARTESIAN_POINT('Ctrl Pts',(25.3744989292576,-2.06208025174567,24.7819920961219));
#44490=CARTESIAN_POINT('Ctrl Pts',(25.3281950990947,-1.22648007969423,25.0611629084752));
#44491=CARTESIAN_POINT('Ctrl Pts',(25.2818912689318,-0.375007937245508,
25.1234854841417));
#44492=CARTESIAN_POINT('Ctrl Pts',(25.235587438769,0.476464205203244,25.1858080598083));
#44493=CARTESIAN_POINT('Ctrl Pts',(25.1892836086061,1.34380831804928,25.031282398788));
#44494=CARTESIAN_POINT('Ctrl Pts',(25.1429797784432,2.12136693606468,24.6787323904857));
#44495=CARTESIAN_POINT('Ctrl Pts',(25.0966759482803,2.89892555408006,24.3261823821834));
#44496=CARTESIAN_POINT('Ctrl Pts',(25.0503721181174,3.5866986772648,23.7756080265991));
#44497=CARTESIAN_POINT('Ctrl Pts',(25.0040682879546,4.10090368258461,23.0940787716819));
#44498=CARTESIAN_POINT('Ctrl Pts',(24.9577644577917,4.61510868790441,22.4125495167647));
#44499=CARTESIAN_POINT('Ctrl Pts',(24.9114606276288,4.95574557535929,21.6000653625146));
#44500=CARTESIAN_POINT('Ctrl Pts',(24.8651567974659,5.08131889976369,20.755600885463));
#44501=CARTESIAN_POINT('Ctrl Pts',(24.818852967303,5.20689222416809,19.9111364084115));
#44502=CARTESIAN_POINT('Ctrl Pts',(24.7725491371402,5.11740198552201,19.0346916085584));
#44503=CARTESIAN_POINT('Ctrl Pts',(24.7262453069773,4.82374963762902,18.2330325716974));
#44504=CARTESIAN_POINT('Ctrl Pts',(24.6799414768144,4.53009728973603,17.4313735348365));
#44505=CARTESIAN_POINT('Ctrl Pts',(24.6336376466515,4.03228283259613,16.7045002609676));
#44506=CARTESIAN_POINT('Ctrl Pts',(24.5873338164887,3.39094864899165,16.1409584455321));
#44507=CARTESIAN_POINT('Ctrl Pts',(24.5410299863258,2.74961446538713,15.5774166300966));
#44508=CARTESIAN_POINT('Ctrl Pts',(24.4947261561629,1.96476055531803,15.1772062730945));
#44509=CARTESIAN_POINT('Ctrl Pts',(24.448422326,1.13199565525229,14.9890798952989));
#44510=CARTESIAN_POINT('Ctrl Pts',(24.4021184958371,0.299230755186634,14.8009535175032));
#44511=CARTESIAN_POINT('Ctrl Pts',(24.3558146656743,-0.581445134875576,
14.8249111189138));
#44512=CARTESIAN_POINT('Ctrl Pts',(24.3095108355114,-1.40275050941299,15.0580342506701));
#44513=CARTESIAN_POINT('Ctrl Pts',(24.2632070053485,-2.22405588395042,15.2911573824264));
#44514=CARTESIAN_POINT('Ctrl Pts',(24.2169031751856,-2.98599074296305,15.7334460445283));
#44515=CARTESIAN_POINT('Ctrl Pts',(24.1705993450227,-3.59573828550665,16.3310218532472));
#44516=CARTESIAN_POINT('Ctrl Pts',(24.1242955148599,-4.20548582805026,16.928597661966));
#44517=CARTESIAN_POINT('Ctrl Pts',(24.077991684697,-4.66304605412489,17.6814606173018));
#44518=CARTESIAN_POINT('Ctrl Pts',(24.0316878545341,-4.91268024024106,18.4978990325703));
#44519=CARTESIAN_POINT('Ctrl Pts',(24.0041390714571,-5.06120182080424,18.9836446980768));
#44520=CARTESIAN_POINT('Ctrl Pts',(23.9765902883801,-5.13612304993768,19.4918944048967));
#44521=CARTESIAN_POINT('Ctrl Pts',(23.9490415053031,-5.13637392180183,20.0000717483683));
#44522=CARTESIAN_POINT('Ctrl Pts',(24.4259584946968,-5.13707231536035,19.9999148579252));
#44523=CARTESIAN_POINT('Ctrl Pts',(24.4307342464949,-5.13714132926883,19.9118536314043));
#44524=CARTESIAN_POINT('Ctrl Pts',(24.4355099982929,-5.13492360976748,19.8237958807944));
#44525=CARTESIAN_POINT('Ctrl Pts',(24.4402857500909,-5.13039600219461,19.7358570568002));
#44526=CARTESIAN_POINT('Ctrl Pts',(24.4865895802538,-5.08649808183254,18.8832364552351));
#44527=CARTESIAN_POINT('Ctrl Pts',(24.5328934104167,-4.82545944153983,18.041795534308));
#44528=CARTESIAN_POINT('Ctrl Pts',(24.5791972405795,-4.3790790877908,17.3140363039218));
#44529=CARTESIAN_POINT('Ctrl Pts',(24.6255010707424,-3.93269873404178,16.5862770735357));
#44530=CARTESIAN_POINT('Ctrl Pts',(24.6718049009053,-3.30097666683647,15.9721995336905));
#44531=CARTESIAN_POINT('Ctrl Pts',(24.7181087310681,-2.56086752431778,15.5466089149199));
#44532=CARTESIAN_POINT('Ctrl Pts',(24.764412561231,-1.82075838179906,15.1210182961492));
#44533=CARTESIAN_POINT('Ctrl Pts',(24.8107163913939,-0.972262163966955,
14.8839145984532));
#44534=CARTESIAN_POINT('Ctrl Pts',(24.8570202215568,-0.118740337514819,
14.8641811396795));
#44535=CARTESIAN_POINT('Ctrl Pts',(24.9033240517197,0.734781488937317,14.8444476809058));
#44536=CARTESIAN_POINT('Ctrl Pts',(24.9496278818825,1.59332892400947,15.0420844610545));
#44537=CARTESIAN_POINT('Ctrl Pts',(24.9959317120454,2.35231608947392,15.4330159132116));
#44538=CARTESIAN_POINT('Ctrl Pts',(25.0422355422083,3.1113032549384,15.8239473653686));
#44539=CARTESIAN_POINT('Ctrl Pts',(25.0885393723712,3.77073015079515,16.408173489534));
#44540=CARTESIAN_POINT('Ctrl Pts',(25.1348432025341,4.25026721316356,17.1145254722172));
#44541=CARTESIAN_POINT('Ctrl Pts',(25.181147032697,4.72980427553196,17.8208774549004));
#44542=CARTESIAN_POINT('Ctrl Pts',(25.2274508628598,5.02945150441205,18.6493552961014));
#44543=CARTESIAN_POINT('Ctrl Pts',(25.2737546930227,5.11270670165989,19.4990361125004));
#44544=CARTESIAN_POINT('Ctrl Pts',(25.3200585231856,5.19596189890774,20.3487169288995));
#44545=CARTESIAN_POINT('Ctrl Pts',(25.3663623533485,5.06282506452336,21.2196007204967));
#44546=CARTESIAN_POINT('Ctrl Pts',(25.4126661835114,4.72951456010185,22.0055988281711));
#44547=CARTESIAN_POINT('Ctrl Pts',(25.4589700136742,4.39620405568035,22.7915969358455));
#44548=CARTESIAN_POINT('Ctrl Pts',(25.5052738438371,3.86271988122177,23.4927093595969));
#44549=CARTESIAN_POINT('Ctrl Pts',(25.551577674,3.19404960599373,24.023528519624));
#44550=CARTESIAN_POINT('Ctrl Pts',(25.5978815041629,2.52537933076573,24.5543476796511));
#44551=CARTESIAN_POINT('Ctrl Pts',(25.6441853343257,1.72152295476826,24.9148735759537));
#44552=CARTESIAN_POINT('Ctrl Pts',(25.6904891644886,0.880404042405986,25.0611879391989));
#44553=CARTESIAN_POINT('Ctrl Pts',(25.7367929946515,0.0392851300436907,
25.207502302444));
#44554=CARTESIAN_POINT('Ctrl Pts',(25.7830968248144,-0.839096318683453,
25.1396051326317));
#44555=CARTESIAN_POINT('Ctrl Pts',(25.8294006549773,-1.64773830076283,24.8657674755352));
#44556=CARTESIAN_POINT('Ctrl Pts',(25.8757044851401,-2.4563802828422,24.5919298184387));
#44557=CARTESIAN_POINT('Ctrl Pts',(25.922008315303,-3.19528279827379,24.112151674058));
#44558=CARTESIAN_POINT('Ctrl Pts',(25.9683121454659,-3.77443478261991,23.4848782913505));
#44559=CARTESIAN_POINT('Ctrl Pts',(26.0146159756288,-4.35358676696605,22.8576049086429));
#44560=CARTESIAN_POINT('Ctrl Pts',(26.0609198057917,-4.7729882202267,22.0828362876086));
#44561=CARTESIAN_POINT('Ctrl Pts',(26.1072236359545,-4.98154881526628,21.2549526026491));
#44562=CARTESIAN_POINT('Ctrl Pts',(26.1301352555353,-5.08474677958754,20.8453070942711));
#44563=CARTESIAN_POINT('Ctrl Pts',(26.1530468751161,-5.13632301784513,20.422657032113));
#44564=CARTESIAN_POINT('Ctrl Pts',(26.1759584946969,-5.13631118199777,20.0000041318326));
#44565=CARTESIAN_POINT('Origin',(25.,0.,20.));
#44566=CARTESIAN_POINT('',(27.9259584946968,-5.13709288667488,20.0000779211054));
#44567=CARTESIAN_POINT('',(27.4490415053031,-5.13638193362529,19.999924256499));
#44568=CARTESIAN_POINT('',(25.,-5.13675,20.));
#44569=CARTESIAN_POINT('Ctrl Pts',(27.4490415053031,-5.13638193362529,19.999924256499));
#44570=CARTESIAN_POINT('Ctrl Pts',(27.4212155456225,-5.13611389747151,20.5132122334074));
#44571=CARTESIAN_POINT('Ctrl Pts',(27.3933895859419,-5.05965382718386,21.0265783069614));
#44572=CARTESIAN_POINT('Ctrl Pts',(27.3655636262614,-4.90817380383266,21.5167611448673));
#44573=CARTESIAN_POINT('Ctrl Pts',(27.3192597960985,-4.65610324257109,22.33245063539));
#44574=CARTESIAN_POINT('Ctrl Pts',(27.2729559659356,-4.19629737338143,23.0839441833737));
#44575=CARTESIAN_POINT('Ctrl Pts',(27.2266521357728,-3.58476847779756,23.679696919557));
#44576=CARTESIAN_POINT('Ctrl Pts',(27.1803483056099,-2.97323958221369,24.2754496557403));
#44577=CARTESIAN_POINT('Ctrl Pts',(27.134044475447,-2.20998766023563,24.7154615801233));
#44578=CARTESIAN_POINT('Ctrl Pts',(27.0877406452841,-1.38798995378171,24.9461316548803));
#44579=CARTESIAN_POINT('Ctrl Pts',(27.0414368151212,-0.5659922473278,25.1768017296374));
#44580=CARTESIAN_POINT('Ctrl Pts',(26.9951329849583,0.314751243601958,25.1981299547686));
#44581=CARTESIAN_POINT('Ctrl Pts',(26.9488291547955,1.14695077853503,25.0075181847724));
#44582=CARTESIAN_POINT('Ctrl Pts',(26.9025253246326,1.9791503134681,24.8169064147761));
#44583=CARTESIAN_POINT('Ctrl Pts',(26.8562214944697,2.76280589240449,24.4143546496523));
#44584=CARTESIAN_POINT('Ctrl Pts',(26.8099176643068,3.40245475626642,23.8489006340471));
#44585=CARTESIAN_POINT('Ctrl Pts',(26.763613834144,4.04210362012837,23.2834466184419));
#44586=CARTESIAN_POINT('Ctrl Pts',(26.7173100039811,4.53774576891585,22.5550903523552));
#44587=CARTESIAN_POINT('Ctrl Pts',(26.6710061738182,4.82900344445263,21.752558185246));
#44588=CARTESIAN_POINT('Ctrl Pts',(26.6247023436553,5.1202611199894,20.9500260181369));
#44589=CARTESIAN_POINT('Ctrl Pts',(26.5783985134924,5.20713432227547,20.0733179500054));
#44590=CARTESIAN_POINT('Ctrl Pts',(26.5320946833296,5.07904039765143,19.2292321372598));
#44591=CARTESIAN_POINT('Ctrl Pts',(26.4857908531667,4.95094647302739,18.3851463245142));
#44592=CARTESIAN_POINT('Ctrl Pts',(26.4394870230038,4.60788542149324,17.5736827671547));
#44593=CARTESIAN_POINT('Ctrl Pts',(26.3931831928409,4.09164799320993,16.8936917154169));
#44594=CARTESIAN_POINT('Ctrl Pts',(26.346879362678,3.57541056492662,16.2137006636792));
#44595=CARTESIAN_POINT('Ctrl Pts',(26.3005755325152,2.88599675989413,15.6651821175633));
#44596=CARTESIAN_POINT('Ctrl Pts',(26.2542717023523,2.10738906447981,15.3149550919848));
#44597=CARTESIAN_POINT('Ctrl Pts',(26.2079678721894,1.32878136906554,14.9647280664063));
#44598=CARTESIAN_POINT('Ctrl Pts',(26.1616640420265,0.460979783269443,14.8127925613651));
#44599=CARTESIAN_POINT('Ctrl Pts',(26.1153602118637,-0.390302499588795,
14.8776569406157));
#44600=CARTESIAN_POINT('Ctrl Pts',(26.0690563817008,-1.24158478244708,14.9425213198662));
#44601=CARTESIAN_POINT('Ctrl Pts',(26.0227525515379,-2.07634776236751,15.2241855834085));
#44602=CARTESIAN_POINT('Ctrl Pts',(25.976448721375,-2.79290291778382,15.6883381682879));
#44603=CARTESIAN_POINT('Ctrl Pts',(25.9301448912121,-3.50945807320011,16.1524907531674));
#44604=CARTESIAN_POINT('Ctrl Pts',(25.8838410610492,-4.10780540411229,16.799131659384));
#44605=CARTESIAN_POINT('Ctrl Pts',(25.8375372308864,-4.51505589061035,17.549488877015));
#44606=CARTESIAN_POINT('Ctrl Pts',(25.7913719890253,-4.92108746815155,18.2976002602917));
#44607=CARTESIAN_POINT('Ctrl Pts',(25.7452067471642,-5.13716440285434,19.1488080340486));
#44608=CARTESIAN_POINT('Ctrl Pts',(25.6990415053031,-5.1371911776762,20.0000027150593));
#44609=CARTESIAN_POINT('Ctrl Pts',(26.1759584946969,-5.13631118199777,20.0000041318326));
#44610=CARTESIAN_POINT('Ctrl Pts',(26.199350705279,-5.13629909788329,19.5684857220737));
#44611=CARTESIAN_POINT('Ctrl Pts',(26.2227429158611,-5.08251203280468,19.1369643538796));
#44612=CARTESIAN_POINT('Ctrl Pts',(26.2461351264432,-4.97498580108714,18.7192771912869));
#44613=CARTESIAN_POINT('Ctrl Pts',(26.292438956606,-4.76214245504992,17.892484213769));
#44614=CARTESIAN_POINT('Ctrl Pts',(26.3387427867689,-4.33873602615698,17.1198970076177));
#44615=CARTESIAN_POINT('Ctrl Pts',(26.3850466169318,-3.75634471661833,16.4956300132962));
#44616=CARTESIAN_POINT('Ctrl Pts',(26.4313504470947,-3.17395340707964,15.8713630189747));
#44617=CARTESIAN_POINT('Ctrl Pts',(26.4776542772576,-2.43257721689522,15.395416236483));
#44618=CARTESIAN_POINT('Ctrl Pts',(26.5239581074204,-1.62252854673174,15.125768188851));
#44619=CARTESIAN_POINT('Ctrl Pts',(26.5702619375833,-0.812479876568274,
14.8561201412189));
#44620=CARTESIAN_POINT('Ctrl Pts',(26.6165657677462,0.0662412735742456,
14.7927708284465));
#44621=CARTESIAN_POINT('Ctrl Pts',(26.6628695979091,0.906591519194633,14.9434372889184));
#44622=CARTESIAN_POINT('Ctrl Pts',(26.709173428072,1.74694176481502,15.0941037493902));
#44623=CARTESIAN_POINT('Ctrl Pts',(26.7554772582348,2.54892110591328,15.4587859831063));
#44624=CARTESIAN_POINT('Ctrl Pts',(26.8017810883977,3.21483463329406,15.9930594071849));
#44625=CARTESIAN_POINT('Ctrl Pts',(26.8480849185606,3.88074816067483,16.5273328312634));
#44626=CARTESIAN_POINT('Ctrl Pts',(26.8943887487234,4.41059587433813,17.2311974457045));
#44627=CARTESIAN_POINT('Ctrl Pts',(26.9406925788863,4.73983318863067,18.0189104064349));
#44628=CARTESIAN_POINT('Ctrl Pts',(26.9869964090492,5.06907050292324,18.8066233671654));
#44629=CARTESIAN_POINT('Ctrl Pts',(27.0333002392121,5.19769741784503,19.6781846741854));
#44630=CARTESIAN_POINT('Ctrl Pts',(27.079604069375,5.11004495773869,20.5274231353155));
#44631=CARTESIAN_POINT('Ctrl Pts',(27.1259078995379,5.02239249763235,21.3766615964457));
#44632=CARTESIAN_POINT('Ctrl Pts',(27.1722117297007,4.71846066249789,22.2035772116861));
#44633=CARTESIAN_POINT('Ctrl Pts',(27.2185155598636,4.23527358938399,22.9074374037704));
#44634=CARTESIAN_POINT('Ctrl Pts',(27.2648193900265,3.7520865162701,23.6112975958547));
#44635=CARTESIAN_POINT('Ctrl Pts',(27.3111232201894,3.08964420517678,24.192102364783));
#44636=CARTESIAN_POINT('Ctrl Pts',(27.3574270503523,2.32864354954369,24.579099677114));
#44637=CARTESIAN_POINT('Ctrl Pts',(27.4037308805151,1.5676428939106,24.9660969894449));
#44638=CARTESIAN_POINT('Ctrl Pts',(27.450034710678,0.708083893737729,25.1592868451784));
#44639=CARTESIAN_POINT('Ctrl Pts',(27.4963385408409,-0.145324346679379,
25.1351353894556));
#44640=CARTESIAN_POINT('Ctrl Pts',(27.5426423710038,-0.998732587096511,
25.1109839337327));
#44641=CARTESIAN_POINT('Ctrl Pts',(27.5889462011667,-1.84599006775788,24.8694911665534));
#44642=CARTESIAN_POINT('Ctrl Pts',(27.6352500313295,-2.58388622151231,24.4400750700923));
#44643=CARTESIAN_POINT('Ctrl Pts',(27.6815538614924,-3.32178237526671,24.0106589736313));
#44644=CARTESIAN_POINT('Ctrl Pts',(27.7278576916553,-3.95031720211417,23.3933195478886));
#44645=CARTESIAN_POINT('Ctrl Pts',(27.7741615218182,-4.3929243247327,22.6632593773323));
#44646=CARTESIAN_POINT('Ctrl Pts',(27.820465351981,-4.83553144735123,21.933199206776));
#44647=CARTESIAN_POINT('Ctrl Pts',(27.8667691821439,-5.09221086574084,21.0904182914061));
#44648=CARTESIAN_POINT('Ctrl Pts',(27.9130730123068,-5.13169460180429,20.2375818755491));
#44649=CARTESIAN_POINT('Ctrl Pts',(27.9173681731035,-5.13535712809314,20.1584724470961));
#44650=CARTESIAN_POINT('Ctrl Pts',(27.9216633339002,-5.13715079679223,20.0792764962122));
#44651=CARTESIAN_POINT('Ctrl Pts',(27.9259584946968,-5.13709288667488,20.0000779211054));
#44652=CARTESIAN_POINT('Origin',(25.,0.,20.));
#44653=CARTESIAN_POINT('',(29.6759584946968,-5.13655037571547,19.9998784050199));
#44654=CARTESIAN_POINT('',(29.1990415053031,-5.13683630912746,20.0001288548401));
#44655=CARTESIAN_POINT('',(25.,-5.13675,20.));
#44656=CARTESIAN_POINT('Ctrl Pts',(29.1990415053031,-5.13683630912746,20.0001288548401));
#44657=CARTESIAN_POINT('Ctrl Pts',(29.1898320044066,-5.13701109509047,20.1699675778401));
#44658=CARTESIAN_POINT('Ctrl Pts',(29.1806225035101,-5.1287533857283,20.3397893799859));
#44659=CARTESIAN_POINT('Ctrl Pts',(29.1714130026137,-5.11193684989818,20.5087593752073));
#44660=CARTESIAN_POINT('Ctrl Pts',(29.1251091724508,-5.0273861204115,21.3583122499286));
#44661=CARTESIAN_POINT('Ctrl Pts',(29.0788053422879,-4.7264759427746,22.1863322104349));
#44662=CARTESIAN_POINT('Ctrl Pts',(29.032501512125,-4.24586236406213,22.8919521511687));
#44663=CARTESIAN_POINT('Ctrl Pts',(28.9861976819621,-3.76524878534965,23.5975720919024));
#44664=CARTESIAN_POINT('Ctrl Pts',(28.9398938517992,-3.1049318055616,24.1807920128636));
#44665=CARTESIAN_POINT('Ctrl Pts',(28.8935900216364,-2.34534941614573,24.5705656734581));
#44666=CARTESIAN_POINT('Ctrl Pts',(28.8472861914735,-1.58576702672985,24.9603393340525));
#44667=CARTESIAN_POINT('Ctrl Pts',(28.8009823613106,-0.72691922768615,25.1566667342802));
#44668=CARTESIAN_POINT('Ctrl Pts',(28.7546785311478,0.126571513247889,25.1356318122742));
#44669=CARTESIAN_POINT('Ctrl Pts',(28.7083747009849,0.980062254181953,25.1145968902681));
#44670=CARTESIAN_POINT('Ctrl Pts',(28.662070870822,1.82819593700634,24.8761996460282));
#44671=CARTESIAN_POINT('Ctrl Pts',(28.6157670406591,2.56765525804144,24.449480973671));
#44672=CARTESIAN_POINT('Ctrl Pts',(28.5694632104962,3.30711457907652,24.0227623013138));
#44673=CARTESIAN_POINT('Ctrl Pts',(28.5231593803334,3.93789953832229,23.4077222008393));
#44674=CARTESIAN_POINT('Ctrl Pts',(28.4768555501705,4.38316965354029,22.6792831592595));
#44675=CARTESIAN_POINT('Ctrl Pts',(28.4305517200076,4.82843976875827,21.9508441176798));
#44676=CARTESIAN_POINT('Ctrl Pts',(28.3842478898447,5.08819503994849,21.1090061349946));
#44677=CARTESIAN_POINT('Ctrl Pts',(28.3379440596818,5.13079279711745,20.2563195900744));
#44678=CARTESIAN_POINT('Ctrl Pts',(28.2916402295189,5.17339055428642,19.403633045154));
#44679=CARTESIAN_POINT('Ctrl Pts',(28.2453363993561,4.99883079743415,18.5400979379986));
#44680=CARTESIAN_POINT('Ctrl Pts',(28.1990325691932,4.62837791420866,17.7709077312786));
#44681=CARTESIAN_POINT('Ctrl Pts',(28.1527287390303,4.25792503098319,17.0017175245586));
#44682=CARTESIAN_POINT('Ctrl Pts',(28.1064249088674,3.69157902138449,16.3268722182742));
#44683=CARTESIAN_POINT('Ctrl Pts',(28.0601210787046,2.99833059271081,15.8285796044965));
#44684=CARTESIAN_POINT('Ctrl Pts',(28.0138172485417,2.30508216403714,15.3302869907188));
#44685=CARTESIAN_POINT('Ctrl Pts',(27.9675134183788,1.48493131628847,15.0085470694478));
#44686=CARTESIAN_POINT('Ctrl Pts',(27.9212095882159,0.637786561431619,14.9025533096201));
#44687=CARTESIAN_POINT('Ctrl Pts',(27.8749057580531,-0.209358193425278,
14.7965595497923));
#44688=CARTESIAN_POINT('Ctrl Pts',(27.8286019278902,-1.08349685539034,14.9063119514078));
#44689=CARTESIAN_POINT('Ctrl Pts',(27.7822980977273,-1.87814426602063,15.2184407799106));
#44690=CARTESIAN_POINT('Ctrl Pts',(27.7359942675644,-2.6727916766509,15.5305696084134));
#44691=CARTESIAN_POINT('Ctrl Pts',(27.6896904374015,-3.38794783594639,16.0450748638036));
#44692=CARTESIAN_POINT('Ctrl Pts',(27.6433866072387,-3.93649439501402,16.6992809363365));
#44693=CARTESIAN_POINT('Ctrl Pts',(27.5970827770758,-4.48504095408165,17.3534870088695));
#44694=CARTESIAN_POINT('Ctrl Pts',(27.5507789469129,-4.8669779129214,18.1473938985452));
#44695=CARTESIAN_POINT('Ctrl Pts',(27.50447511675,-5.03577876567455,18.984290059914));
#44696=CARTESIAN_POINT('Ctrl Pts',(27.4859972462677,-5.10313993824936,19.3182593843202));
#44697=CARTESIAN_POINT('Ctrl Pts',(27.4675193757854,-5.13655992343736,19.6590746014891));
#44698=CARTESIAN_POINT('Ctrl Pts',(27.4490415053031,-5.13638193362529,19.999924256499));
#44699=CARTESIAN_POINT('Ctrl Pts',(27.9259584946968,-5.13709288667488,20.0000779211054));
#44700=CARTESIAN_POINT('Ctrl Pts',(27.967967164063,-5.13652649880541,19.2254790379847));
#44701=CARTESIAN_POINT('Ctrl Pts',(28.0099758334292,-4.95884272242568,18.4506291282816));
#44702=CARTESIAN_POINT('Ctrl Pts',(28.0519845027954,-4.62020714167552,17.7540212374586));
#44703=CARTESIAN_POINT('Ctrl Pts',(28.0982883329583,-4.24694789174599,16.9861889315691));
#44704=CARTESIAN_POINT('Ctrl Pts',(28.1445921631212,-3.67814133814964,16.3134162361345));
#44705=CARTESIAN_POINT('Ctrl Pts',(28.1908959932841,-2.98307792486126,15.8176584634942));
#44706=CARTESIAN_POINT('Ctrl Pts',(28.237199823447,-2.28801451157289,15.3219006908538));
#44707=CARTESIAN_POINT('Ctrl Pts',(28.2835036536098,-1.46669423859254,15.0031578410078));
#44708=CARTESIAN_POINT('Ctrl Pts',(28.3298074837727,-0.619168074040091,
14.9002582879261));
#44709=CARTESIAN_POINT('Ctrl Pts',(28.3761113139356,0.228358090512335,14.7973587348444));
#44710=CARTESIAN_POINT('Ctrl Pts',(28.4224151440985,1.10209014663687,14.9103024785271));
#44711=CARTESIAN_POINT('Ctrl Pts',(28.4687189742614,1.89559246749136,15.2253310239382));
#44712=CARTESIAN_POINT('Ctrl Pts',(28.5150228044242,2.68909478834583,15.5403595693494));
#44713=CARTESIAN_POINT('Ctrl Pts',(28.5613266345871,3.40236737393034,16.0574729164892));
#44714=CARTESIAN_POINT('Ctrl Pts',(28.60763046475,3.948521327101,16.7136777450765));
#44715=CARTESIAN_POINT('Ctrl Pts',(28.6539342949129,4.49467528027171,17.369882573664));
#44716=CARTESIAN_POINT('Ctrl Pts',(28.7002381250758,4.87371060102853,18.1651788836989));
#44717=CARTESIAN_POINT('Ctrl Pts',(28.7465419552386,5.03945425305308,19.0026858743796));
#44718=CARTESIAN_POINT('Ctrl Pts',(28.7928457854015,5.20519790507761,19.8401928650602));
#44719=CARTESIAN_POINT('Ctrl Pts',(28.8391496155644,5.15764988836987,20.7199105363865));
#44720=CARTESIAN_POINT('Ctrl Pts',(28.8854534457272,4.90260237105269,21.5346741103978));
#44721=CARTESIAN_POINT('Ctrl Pts',(28.9317572758901,4.6475548537355,22.3494376844091));
#44722=CARTESIAN_POINT('Ctrl Pts',(28.978061106053,4.18500783580885,23.0992471611055));
#44723=CARTESIAN_POINT('Ctrl Pts',(29.0243649362159,3.57130751797791,23.6927628201404));
#44724=CARTESIAN_POINT('Ctrl Pts',(29.0706687663788,2.95760720014698,24.2862784791752));
#44725=CARTESIAN_POINT('Ctrl Pts',(29.1169725965417,2.19275358241176,24.7235003205486));
#44726=CARTESIAN_POINT('Ctrl Pts',(29.1632764267045,1.36991902084573,24.9511671866442));
#44727=CARTESIAN_POINT('Ctrl Pts',(29.2095802568674,0.547084459279668,25.1788340527397));
#44728=CARTESIAN_POINT('Ctrl Pts',(29.2558840870303,-0.333731046117226,
25.1969459435576));
#44729=CARTESIAN_POINT('Ctrl Pts',(29.3021879171932,-1.16522898226883,25.0032965185623));
#44730=CARTESIAN_POINT('Ctrl Pts',(29.348491747356,-1.99672691842042,24.809647093567));
#44731=CARTESIAN_POINT('Ctrl Pts',(29.3947955775189,-2.77890728532674,24.4042363527586));
#44732=CARTESIAN_POINT('Ctrl Pts',(29.4410994076818,-3.41648703016668,23.8364503133078));
#44733=CARTESIAN_POINT('Ctrl Pts',(29.4874032378447,-4.05406677500665,23.268664273857));
#44734=CARTESIAN_POINT('Ctrl Pts',(29.5337070680076,-4.54704589778025,22.5385029357639));
#44735=CARTESIAN_POINT('Ctrl Pts',(29.5800108981704,-4.83537104278805,21.7349125373757));
#44736=CARTESIAN_POINT('Ctrl Pts',(29.6119934303459,-5.03452018865289,21.1798643765229));
#44737=CARTESIAN_POINT('Ctrl Pts',(29.6439759625214,-5.13603286926705,20.5897846273661));
#44738=CARTESIAN_POINT('Ctrl Pts',(29.6759584946968,-5.13655037571547,19.9998784050199));
#44739=CARTESIAN_POINT('Origin',(25.,0.,20.));
#44740=CARTESIAN_POINT('',(31.4259584946968,-5.13659957288456,20.0001275332863));
#44741=CARTESIAN_POINT('',(30.9490415053031,-5.1368247808178,19.9998702638696));
#44742=CARTESIAN_POINT('',(25.,-5.13675,20.));
#44743=CARTESIAN_POINT('Ctrl Pts',(30.9490415053031,-5.1368247808178,19.9998702638696));
#44744=CARTESIAN_POINT('Ctrl Pts',(30.9121446330278,-5.13612325801613,20.6803151941057));
#44745=CARTESIAN_POINT('Ctrl Pts',(30.8752477607525,-5.0001139989638,21.3610321796951));
#44746=CARTESIAN_POINT('Ctrl Pts',(30.8383508884773,-4.7368068132147,21.9883147822946));
#44747=CARTESIAN_POINT('Ctrl Pts',(30.7920470583144,-4.4063687446805,22.7755247896416));
#44748=CARTESIAN_POINT('Ctrl Pts',(30.7457432281516,-3.87544836617376,23.4785806492208));
#44749=CARTESIAN_POINT('Ctrl Pts',(30.6994393979887,-3.20872093241755,24.0118380372435));
#44750=CARTESIAN_POINT('Ctrl Pts',(30.6531355678258,-2.54199349866135,24.5450954252662));
#44751=CARTESIAN_POINT('Ctrl Pts',(30.6068317376629,-1.73945900965567,24.9085543417324));
#44752=CARTESIAN_POINT('Ctrl Pts',(30.5605279075,-0.898880001181268,25.0579392248904));
#44753=CARTESIAN_POINT('Ctrl Pts',(30.5142240773371,-0.0583009927068438,
25.2073241080484));
#44754=CARTESIAN_POINT('Ctrl Pts',(30.4679202471743,0.820322535236316,25.1426349578981));
#44755=CARTESIAN_POINT('Ctrl Pts',(30.4216164170114,1.6299590902138,24.8717520281145));
#44756=CARTESIAN_POINT('Ctrl Pts',(30.3753125868485,2.43959564519129,24.6008690983309));
#44757=CARTESIAN_POINT('Ctrl Pts',(30.3290087566856,3.18024522720312,24.1237923889139));
#44758=CARTESIAN_POINT('Ctrl Pts',(30.2827049265227,3.76168394898414,23.4986380674719));
#44759=CARTESIAN_POINT('Ctrl Pts',(30.2364010963599,4.34312267076514,22.8734837460299));
#44760=CARTESIAN_POINT('Ctrl Pts',(30.190097266197,4.76535053231536,22.1002518125629));
#44761=CARTESIAN_POINT('Ctrl Pts',(30.1437934360341,4.97693290124465,21.2731352464357));
#44762=CARTESIAN_POINT('Ctrl Pts',(30.0974896058712,5.18851527017395,20.4460186803083));
#44763=CARTESIAN_POINT('Ctrl Pts',(30.0511857757083,5.18945214648229,19.5650174815208));
#44764=CARTESIAN_POINT('Ctrl Pts',(30.0048819455455,4.97962940248438,18.7374527838052));
#44765=CARTESIAN_POINT('Ctrl Pts',(29.9585781153826,4.76980665848647,17.9098880860896));
#44766=CARTESIAN_POINT('Ctrl Pts',(29.9122742852197,4.3492242941823,17.135759889446));
#44767=CARTESIAN_POINT('Ctrl Pts',(29.8659704550569,3.76911649203047,16.5093703535448));
#44768=CARTESIAN_POINT('Ctrl Pts',(29.819666624894,3.18900868987863,15.8829808176436));
#44769=CARTESIAN_POINT('Ctrl Pts',(29.7733627947311,2.4493754498791,15.4043299424848));
#44770=CARTESIAN_POINT('Ctrl Pts',(29.7270589645682,1.64031685131906,15.1317256562015));
#44771=CARTESIAN_POINT('Ctrl Pts',(29.6807551344053,0.831258252759049,14.8591213699182));
#44772=CARTESIAN_POINT('Ctrl Pts',(29.6344513042424,-0.0472257043614852,
14.7925636725103));
#44773=CARTESIAN_POINT('Ctrl Pts',(29.5881474740796,-0.888120529740423,
14.9401604389208));
#44774=CARTESIAN_POINT('Ctrl Pts',(29.5418436439167,-1.72901535511936,15.0877572053314));
#44775=CARTESIAN_POINT('Ctrl Pts',(29.4955398137538,-2.53232104875672,15.4495084355604));
#44776=CARTESIAN_POINT('Ctrl Pts',(29.4492359835909,-3.20018112885267,15.9813465934789));
#44777=CARTESIAN_POINT('Ctrl Pts',(29.402932153428,-3.86804120894865,16.5131847513974));
#44778=CARTESIAN_POINT('Ctrl Pts',(29.3566283232652,-4.40045567550322,17.2151098370055));
#44779=CARTESIAN_POINT('Ctrl Pts',(29.3103244931023,-4.73256726811228,18.0016152742776));
#44780=CARTESIAN_POINT('Ctrl Pts',(29.2732301638359,-4.99862423847722,18.6316904010514));
#44781=CARTESIAN_POINT('Ctrl Pts',(29.2361358345695,-5.13613230050249,19.3160468851478));
#44782=CARTESIAN_POINT('Ctrl Pts',(29.1990415053031,-5.13683630912746,20.0001288548401));
#44783=CARTESIAN_POINT('Ctrl Pts',(29.6759584946968,-5.13655037571547,19.9998784050199));
#44784=CARTESIAN_POINT('Ctrl Pts',(29.6902797926843,-5.13678210733751,19.735727250618));
#44785=CARTESIAN_POINT('Ctrl Pts',(29.7046010906717,-5.11676315508257,19.4716108903201));
#44786=CARTESIAN_POINT('Ctrl Pts',(29.7189223886591,-5.0761919539234,19.210690250472));
#44787=CARTESIAN_POINT('Ctrl Pts',(29.765226218822,-4.94501655280897,18.3670778206395));
#44788=CARTESIAN_POINT('Ctrl Pts',(29.8115300489848,-4.59899458333809,17.5568724196578));
#44789=CARTESIAN_POINT('Ctrl Pts',(29.8578338791477,-4.08027748652016,16.8787710326262));
#44790=CARTESIAN_POINT('Ctrl Pts',(29.9041377093106,-3.56156038970222,16.2006696455946));
#44791=CARTESIAN_POINT('Ctrl Pts',(29.9504415394735,-2.87014816553721,15.6546722725132));
#44792=CARTESIAN_POINT('Ctrl Pts',(29.9967453696363,-2.09026674229388,15.307290805959));
#44793=CARTESIAN_POINT('Ctrl Pts',(30.0430491997992,-1.31038531905059,14.9599093394048));
#44794=CARTESIAN_POINT('Ctrl Pts',(30.0893530299621,-0.442034696728981,
14.8111437793778));
#44795=CARTESIAN_POINT('Ctrl Pts',(30.135656860125,0.409005049237525,14.8791163356824));
#44796=CARTESIAN_POINT('Ctrl Pts',(30.1819606902879,1.26004479520408,14.947088891987));
#44797=CARTESIAN_POINT('Ctrl Pts',(30.2282645204507,2.09377366481553,15.2317995646233));
#44798=CARTESIAN_POINT('Ctrl Pts',(30.2745683506136,2.80862910896845,15.6985656854914));
#44799=CARTESIAN_POINT('Ctrl Pts',(30.3208721807765,3.52348455312135,16.1653318063596));
#44800=CARTESIAN_POINT('Ctrl Pts',(30.3671760109394,4.11946657181572,16.8141533754597));
#44801=CARTESIAN_POINT('Ctrl Pts',(30.4134798411023,4.52397428094567,17.565992740537));
#44802=CARTESIAN_POINT('Ctrl Pts',(30.4597836712652,4.92848199007563,18.3178321056142));
#44803=CARTESIAN_POINT('Ctrl Pts',(30.506087501428,5.14151538964116,19.1726892666687));
#44804=CARTESIAN_POINT('Ctrl Pts',(30.5523913315909,5.13712333905848,20.0264278844652));
#44805=CARTESIAN_POINT('Ctrl Pts',(30.5986951617538,5.13273128847581,20.8801665022617));
#44806=CARTESIAN_POINT('Ctrl Pts',(30.6449989919167,4.91091378774491,21.7327865768002));
#44807=CARTESIAN_POINT('Ctrl Pts',(30.6913028220795,4.49869203240205,22.4804242845487));
#44808=CARTESIAN_POINT('Ctrl Pts',(30.7376066522424,4.08647027705919,23.2280619922972));
#44809=CARTESIAN_POINT('Ctrl Pts',(30.7839104824053,3.48384426710438,23.8707173332557));
#44810=CARTESIAN_POINT('Ctrl Pts',(30.8302143125682,2.76422423931584,24.3301038080577));
#44811=CARTESIAN_POINT('Ctrl Pts',(30.876518142731,2.04460421152731,24.7894902828596));
#44812=CARTESIAN_POINT('Ctrl Pts',(30.9228219728939,1.20799016590505,25.0656078915051));
#44813=CARTESIAN_POINT('Ctrl Pts',(30.9691258030568,0.356296115728621,25.1248207492256));
#44814=CARTESIAN_POINT('Ctrl Pts',(31.0154296332197,-0.495397934447808,
25.1840336069461));
#44815=CARTESIAN_POINT('Ctrl Pts',(31.0617334633826,-1.36217198917841,25.0263417137417));
#44816=CARTESIAN_POINT('Ctrl Pts',(31.1080372935454,-2.13843802614104,24.6709546606803));
#44817=CARTESIAN_POINT('Ctrl Pts',(31.1543411237083,-2.91470406310367,24.3155676076188));
#44818=CARTESIAN_POINT('Ctrl Pts',(31.2006449538712,-3.60046208229834,23.7624853947004));
#44819=CARTESIAN_POINT('Ctrl Pts',(31.2469487840341,-4.11217493509543,23.0790829701308));
#44820=CARTESIAN_POINT('Ctrl Pts',(31.293252614197,-4.62388778789254,22.3956805455612));
#44821=CARTESIAN_POINT('Ctrl Pts',(31.3395564443598,-4.96155547429207,21.5819579093403));
#44822=CARTESIAN_POINT('Ctrl Pts',(31.3858602745227,-5.08404424898353,20.7370405064541));
#44823=CARTESIAN_POINT('Ctrl Pts',(31.3992263479141,-5.11940188454817,20.4931464705417));
#44824=CARTESIAN_POINT('Ctrl Pts',(31.4125924213055,-5.13682979808384,20.2466531395095));
#44825=CARTESIAN_POINT('Ctrl Pts',(31.4259584946968,-5.13659957288456,20.0001275332863));
#44826=CARTESIAN_POINT('Origin',(25.,0.,20.));
#44827=CARTESIAN_POINT('',(33.1759584946969,-5.13705066379934,19.9999081473515));
#44828=CARTESIAN_POINT('',(32.6990415053031,-5.13638791342383,20.0000785319455));
#44829=CARTESIAN_POINT('',(25.,-5.13675,20.));
#44830=CARTESIAN_POINT('Ctrl Pts',(32.6990415053031,-5.13638791342383,20.0000785319455));
#44831=CARTESIAN_POINT('Ctrl Pts',(32.6807610918119,-5.13657075558928,20.3372846981639));
#44832=CARTESIAN_POINT('Ctrl Pts',(32.6624806783207,-5.10386611251029,20.6744558642531));
#44833=CARTESIAN_POINT('Ctrl Pts',(32.6442002648296,-5.03792763082465,21.0049973362063));
#44834=CARTESIAN_POINT('Ctrl Pts',(32.5978964346667,-4.87090710589811,21.842250617512));
#44835=CARTESIAN_POINT('Ctrl Pts',(32.5515926045038,-4.49065952554585,22.6369680312125));
#44836=CARTESIAN_POINT('Ctrl Pts',(32.5052887743409,-3.94350560020336,23.2923392960588));
#44837=CARTESIAN_POINT('Ctrl Pts',(32.458984944178,-3.39635167486089,23.9477105609051));
#44838=CARTESIAN_POINT('Ctrl Pts',(32.4126811140152,-2.68229140452821,24.4637356768973));
#44839=CARTESIAN_POINT('Ctrl Pts',(32.3663772838523,-1.88830963993053,24.7775538890685));
#44840=CARTESIAN_POINT('Ctrl Pts',(32.3200734536894,-1.09432787533286,25.0913721012397));
#44841=CARTESIAN_POINT('Ctrl Pts',(32.2737696235265,-0.220424616470207,
25.2029834095897));
#44842=CARTESIAN_POINT('Ctrl Pts',(32.2274657933636,0.626943654370524,25.0987916326766));
#44843=CARTESIAN_POINT('Ctrl Pts',(32.1811619632008,1.47431192521126,24.9945998557634));
#44844=CARTESIAN_POINT('Ctrl Pts',(32.1348581330379,2.29514520803006,24.674604993587));
#44845=CARTESIAN_POINT('Ctrl Pts',(32.088554302875,2.98945185850394,24.1777879368029));
#44846=CARTESIAN_POINT('Ctrl Pts',(32.0422504727122,3.68375850897784,23.6809708800187));
#44847=CARTESIAN_POINT('Ctrl Pts',(31.9959466425492,4.2515385271068,23.0073316286267));
#44848=CARTESIAN_POINT('Ctrl Pts',(31.9496428123864,4.62362651863257,22.2389310564209));
#44849=CARTESIAN_POINT('Ctrl Pts',(31.9033389822235,4.99571451015832,21.470530484215));
#44850=CARTESIAN_POINT('Ctrl Pts',(31.8570351520606,5.1721104750809,20.6073685911953));
#44851=CARTESIAN_POINT('Ctrl Pts',(31.8107313218978,5.1313263439546,19.7545933761168));
#44852=CARTESIAN_POINT('Ctrl Pts',(31.7644274917349,5.0905422128283,18.9018181610383));
#44853=CARTESIAN_POINT('Ctrl Pts',(31.718123661572,4.83257798565312,18.059429623901));
#44854=CARTESIAN_POINT('Ctrl Pts',(31.6718198314091,4.38885815238538,17.3300452105984));
#44855=CARTESIAN_POINT('Ctrl Pts',(31.6255160012462,3.94513831911763,16.6006607972957));
#44856=CARTESIAN_POINT('Ctrl Pts',(31.5792121710834,3.31566287975732,15.9842805078278));
#44857=CARTESIAN_POINT('Ctrl Pts',(31.5329083409205,2.57711279444588,15.5559900873297));
#44858=CARTESIAN_POINT('Ctrl Pts',(31.4866045107576,1.83856270913447,15.1276996668317));
#44859=CARTESIAN_POINT('Ctrl Pts',(31.4403006805947,0.990937977871945,14.8874991153034));
#44860=CARTESIAN_POINT('Ctrl Pts',(31.3939968504318,0.137493905263782,14.8646490007767));
#44861=CARTESIAN_POINT('Ctrl Pts',(31.3476930202689,-0.71595016734443,14.84179888625));
#44862=CARTESIAN_POINT('Ctrl Pts',(31.3013891901061,-1.57521358129828,15.0362992087248));
#44863=CARTESIAN_POINT('Ctrl Pts',(31.2550853599432,-2.33562323979935,15.4244564759018));
#44864=CARTESIAN_POINT('Ctrl Pts',(31.2087815297803,-3.09603289830041,15.8126137430787));
#44865=CARTESIAN_POINT('Ctrl Pts',(31.1624776996174,-3.7575888013487,16.3944279549576));
#44866=CARTESIAN_POINT('Ctrl Pts',(31.1161738694545,-4.23970203528538,17.099024110544));
#44867=CARTESIAN_POINT('Ctrl Pts',(31.0698700392917,-4.72181526922206,17.8036202661303));
#44868=CARTESIAN_POINT('Ctrl Pts',(31.0235662091288,-5.02448583404714,18.630998365424));
#44869=CARTESIAN_POINT('Ctrl Pts',(30.9772623789659,-5.11084323717886,19.4803694926283));
#44870=CARTESIAN_POINT('Ctrl Pts',(30.9678554210783,-5.12838736801396,19.6529253783177));
#44871=CARTESIAN_POINT('Ctrl Pts',(30.9584484631907,-5.13700363596311,19.8263889791738));
#44872=CARTESIAN_POINT('Ctrl Pts',(30.9490415053031,-5.1368247808178,19.9998702638696));
#44873=CARTESIAN_POINT('Ctrl Pts',(31.4259584946968,-5.13659957288456,20.0001275332863));
#44874=CARTESIAN_POINT('Ctrl Pts',(31.4588962514683,-5.13603223336795,19.3926192383697));
#44875=CARTESIAN_POINT('Ctrl Pts',(31.4918340082398,-5.02823267856117,18.7849149465654));
#44876=CARTESIAN_POINT('Ctrl Pts',(31.5247717650114,-4.81726509452241,18.215429563488));
#44877=CARTESIAN_POINT('Ctrl Pts',(31.5710755951742,-4.52068730238642,17.4148481929596));
#44878=CARTESIAN_POINT('Ctrl Pts',(31.6173794253371,-4.02022185513104,16.6897976214544));
#44879=CARTESIAN_POINT('Ctrl Pts',(31.6636832555,-3.3768340718355,16.128601507844));
#44880=CARTESIAN_POINT('Ctrl Pts',(31.7099870856629,-2.73344628853994,15.5674053942336));
#44881=CARTESIAN_POINT('Ctrl Pts',(31.7562909158257,-1.94713616920423,15.170063738518));
#44882=CARTESIAN_POINT('Ctrl Pts',(31.8025947459886,-1.11368984168881,14.9849796041994));
#44883=CARTESIAN_POINT('Ctrl Pts',(31.8488985761515,-0.28024351417343,14.7998954698808));
#44884=CARTESIAN_POINT('Ctrl Pts',(31.8952024063144,0.600339021521638,14.8270688569593));
#44885=CARTESIAN_POINT('Ctrl Pts',(31.9415062364773,1.4207876320462,15.0631895784423));
#44886=CARTESIAN_POINT('Ctrl Pts',(31.9878100666401,2.24123624257079,15.2993102999252));
#44887=CARTESIAN_POINT('Ctrl Pts',(32.034113896803,3.00155092792492,15.7443783558127));
#44888=CARTESIAN_POINT('Ctrl Pts',(32.0804177269659,3.60911225224641,16.3441767842986));
#44889=CARTESIAN_POINT('Ctrl Pts',(32.1267215571288,4.21667357656793,16.9439752127844));
#44890=CARTESIAN_POINT('Ctrl Pts',(32.1730253872917,4.67148153985684,17.6985040138686));
#44891=CARTESIAN_POINT('Ctrl Pts',(32.2193292174545,4.91813269167768,18.515848572137));
#44892=CARTESIAN_POINT('Ctrl Pts',(32.2656330476174,5.16478384349852,19.3331931304053));
#44893=CARTESIAN_POINT('Ctrl Pts',(32.3119368777803,5.20327818385128,20.2133534458577));
#44894=CARTESIAN_POINT('Ctrl Pts',(32.3582407079432,5.02892643847093,21.0491108188484));
#44895=CARTESIAN_POINT('Ctrl Pts',(32.4045445381061,4.85457469309059,21.884868191839));
#44896=CARTESIAN_POINT('Ctrl Pts',(32.4508483682689,4.46737686197716,22.6762226223678));
#44897=CARTESIAN_POINT('Ctrl Pts',(32.4971521984318,3.91450031592533,23.3267734985113));
#44898=CARTESIAN_POINT('Ctrl Pts',(32.5434560285947,3.36162376987346,23.9773243746549));
#44899=CARTESIAN_POINT('Ctrl Pts',(32.5897598587576,2.64306850888318,24.4870716964132));
#44900=CARTESIAN_POINT('Ctrl Pts',(32.6360636889204,1.84636695103165,24.7939194523808));
#44901=CARTESIAN_POINT('Ctrl Pts',(32.6823675190833,1.04966539318013,25.1007672083484));
#44902=CARTESIAN_POINT('Ctrl Pts',(32.7286713492462,0.174817538467357,25.2047153985253));
#44903=CARTESIAN_POINT('Ctrl Pts',(32.7749751794091,-0.671605062761131,
25.0931013413686));
#44904=CARTESIAN_POINT('Ctrl Pts',(32.821279009572,-1.51802766398958,24.9814872842118));
#44905=CARTESIAN_POINT('Ctrl Pts',(32.8675828397349,-2.33602501173377,24.6543109797215));
#44906=CARTESIAN_POINT('Ctrl Pts',(32.9138866698977,-3.02595092745193,24.1514281420289));
#44907=CARTESIAN_POINT('Ctrl Pts',(32.9601905000606,-3.71587684317011,23.6485453043363));
#44908=CARTESIAN_POINT('Ctrl Pts',(33.0064943302235,-4.27773132686224,22.9699559334413));
#44909=CARTESIAN_POINT('Ctrl Pts',(33.0527981603863,-4.64307081651572,22.1983239130293));
#44910=CARTESIAN_POINT('Ctrl Pts',(33.0938516051565,-4.96698450806331,21.5141871489335));
#44911=CARTESIAN_POINT('Ctrl Pts',(33.1349050499267,-5.1364221807677,20.7569116497994));
#44912=CARTESIAN_POINT('Ctrl Pts',(33.1759584946969,-5.13705066379934,19.9999081473515));
#44913=CARTESIAN_POINT('Origin',(25.,0.,20.));
#44914=CARTESIAN_POINT('',(34.9259584946969,-5.13631268534711,20.0000122781576));
#44915=CARTESIAN_POINT('',(34.4490415053031,-5.13719091754074,19.9999934144287));
#44916=CARTESIAN_POINT('',(25.,-5.13675,20.));
#44917=CARTESIAN_POINT('Ctrl Pts',(34.4490415053031,-5.13719058367308,19.9999934194154));
#44918=CARTESIAN_POINT('Ctrl Pts',(34.4030737204331,-5.1371267473639,20.847547674618));
#44919=CARTESIAN_POINT('Ctrl Pts',(34.3571059355632,-4.92296721330138,21.6951330054991));
#44920=CARTESIAN_POINT('Ctrl Pts',(34.3111381506932,-4.52025752915113,22.4409027693378));
#44921=CARTESIAN_POINT('Ctrl Pts',(34.2648343205303,-4.11460385511416,23.1921244473692));
#44922=CARTESIAN_POINT('Ctrl Pts',(34.2185304903674,-3.51763318064836,23.840036481391));
#44923=CARTESIAN_POINT('Ctrl Pts',(34.1722266602046,-2.80206682517619,24.3057120162007));
#44924=CARTESIAN_POINT('Ctrl Pts',(34.1259228300417,-2.08650046970406,24.7713875510104));
#44925=CARTESIAN_POINT('Ctrl Pts',(34.0796189998788,-1.25233843322558,25.0548265866079));
#44926=CARTESIAN_POINT('Ctrl Pts',(34.0333151697159,-0.401196032035998,
25.1215013622069));
#44927=CARTESIAN_POINT('Ctrl Pts',(33.9870113395531,0.449946369153583,25.1881761378058));
#44928=CARTESIAN_POINT('Ctrl Pts',(33.9407075093902,1.31806913505426,25.0380866534062));
#44929=CARTESIAN_POINT('Ctrl Pts',(33.8944036792273,2.09741994707273,24.6895163956244));
#44930=CARTESIAN_POINT('Ctrl Pts',(33.8480998490644,2.87677075909122,24.3409461378425));
#44931=CARTESIAN_POINT('Ctrl Pts',(33.8017960189015,3.56734961722749,23.7938951066785));
#44932=CARTESIAN_POINT('Ctrl Pts',(33.7554921887387,4.08503211156166,23.1150035484279));
#44933=CARTESIAN_POINT('Ctrl Pts',(33.7091883585758,4.60271460589581,22.4361119901773));
#44934=CARTESIAN_POINT('Ctrl Pts',(33.6628845284129,4.94750073642786,21.6253799048401));
#44935=CARTESIAN_POINT('Ctrl Pts',(33.61658069825,5.07738960863597,20.7815684367499));
#44936=CARTESIAN_POINT('Ctrl Pts',(33.5702768680871,5.20727848084407,19.9377569686598));
#44937=CARTESIAN_POINT('Ctrl Pts',(33.5239730379243,5.12227009472827,19.0608661178167));
#44938=CARTESIAN_POINT('Ctrl Pts',(33.4776692077614,4.83271993719056,18.2577163067143));
#44939=CARTESIAN_POINT('Ctrl Pts',(33.4313653775985,4.54316977965285,17.4545664956119));
#44940=CARTESIAN_POINT('Ctrl Pts',(33.3850615474356,4.04907785069323,16.7251577242503));
#44941=CARTESIAN_POINT('Ctrl Pts',(33.3387577172727,3.41063306498843,16.1583445553751));
#44942=CARTESIAN_POINT('Ctrl Pts',(33.2924538871099,2.77218827928362,15.5915313865));
#44943=CARTESIAN_POINT('Ctrl Pts',(33.246150056947,1.98939063683364,15.1873138201114));
#44944=CARTESIAN_POINT('Ctrl Pts',(33.1998462267841,1.15759838526208,14.9949325241664));
#44945=CARTESIAN_POINT('Ctrl Pts',(33.1535423966212,0.325806133690502,14.8025512282215));
#44946=CARTESIAN_POINT('Ctrl Pts',(33.1072385664583,-0.554980727002643,
14.8220062027202));
#44947=CARTESIAN_POINT('Ctrl Pts',(33.0609347362955,-1.37746717315998,15.0509274963813));
#44948=CARTESIAN_POINT('Ctrl Pts',(33.0146309061326,-2.19995361931729,15.2798487900423));
#44949=CARTESIAN_POINT('Ctrl Pts',(32.9683270759697,-2.9641396509388,15.7182364028657));
#44950=CARTESIAN_POINT('Ctrl Pts',(32.9220232458069,-3.57693423544831,16.3126871661756));
#44951=CARTESIAN_POINT('Ctrl Pts',(32.875719415644,-4.18972881995782,16.9071379294855));
#44952=CARTESIAN_POINT('Ctrl Pts',(32.8294155854811,-4.65113195735533,17.657651843282));
#44953=CARTESIAN_POINT('Ctrl Pts',(32.7831117553182,-4.90493679130367,18.4728033746358));
#44954=CARTESIAN_POINT('Ctrl Pts',(32.7550883386465,-5.05854133308798,18.9661390432695));
#44955=CARTESIAN_POINT('Ctrl Pts',(32.7270649219748,-5.13610762095725,19.4831499129748));
#44956=CARTESIAN_POINT('Ctrl Pts',(32.6990415053031,-5.13638791342383,20.0000785319455));
#44957=CARTESIAN_POINT('Ctrl Pts',(33.1759584946969,-5.13705066379934,19.9999081473515));
#44958=CARTESIAN_POINT('Ctrl Pts',(33.1812088800896,-5.13713104141801,19.9030938567668));
#44959=CARTESIAN_POINT('Ctrl Pts',(33.1864592654823,-5.13445033743313,19.8062840150219));
#44960=CARTESIAN_POINT('Ctrl Pts',(33.191709650875,-5.12897856940196,19.7096321843039));
#44961=CARTESIAN_POINT('Ctrl Pts',(33.2380134810379,-5.08072233701988,18.8572471459194));
#44962=CARTESIAN_POINT('Ctrl Pts',(33.2843173112007,-4.81538537664088,18.0171517390795));
#44963=CARTESIAN_POINT('Ctrl Pts',(33.3306211413636,-4.36529030422524,17.2916840668759));
#44964=CARTESIAN_POINT('Ctrl Pts',(33.3769249715265,-3.91519523180961,16.5662163946723));
#44965=CARTESIAN_POINT('Ctrl Pts',(33.4232288016894,-3.28034204735735,15.9553764571049));
#44966=CARTESIAN_POINT('Ctrl Pts',(33.4695326318523,-2.53806681306989,15.5335750889364));
#44967=CARTESIAN_POINT('Ctrl Pts',(33.5158364620152,-1.79579157878242,15.1117737207678));
#44968=CARTESIAN_POINT('Ctrl Pts',(33.562140292178,-0.946094294659754,14.8790109219982));
#44969=CARTESIAN_POINT('Ctrl Pts',(33.6084441223409,-0.0924827379748081,
14.8636412141524));
#44970=CARTESIAN_POINT('Ctrl Pts',(33.6547479525038,0.761128818710162,14.8482715063067));
#44971=CARTESIAN_POINT('Ctrl Pts',(33.7010517826667,1.61865464795741,15.050294889385));
#44972=CARTESIAN_POINT('Ctrl Pts',(33.7473556128296,2.37563332074029,15.4451014326151));
#44973=CARTESIAN_POINT('Ctrl Pts',(33.7936594429924,3.13261199352313,15.8399079758451));
#44974=CARTESIAN_POINT('Ctrl Pts',(33.8399632731553,3.78904350984162,16.4274976792269));
#44975=CARTESIAN_POINT('Ctrl Pts',(33.8862671033182,4.26496319468072,17.1362919873361));
#44976=CARTESIAN_POINT('Ctrl Pts',(33.9325709334811,4.74088287951985,17.8450862954453));
#44977=CARTESIAN_POINT('Ctrl Pts',(33.9788747636439,5.03629073287958,18.6750852082819));
#44978=CARTESIAN_POINT('Ctrl Pts',(34.0251785938068,5.11520098563766,19.525180549779));
#44979=CARTESIAN_POINT('Ctrl Pts',(34.0714824239697,5.19411123839575,20.3752758912761));
#44980=CARTESIAN_POINT('Ctrl Pts',(34.1177862541326,5.05652389055219,21.2454676614337));
#44981=CARTESIAN_POINT('Ctrl Pts',(34.1640900842955,4.71919945296453,22.029751501272));
#44982=CARTESIAN_POINT('Ctrl Pts',(34.2103939144583,4.38187501537688,22.8140353411103));
#44983=CARTESIAN_POINT('Ctrl Pts',(34.2566977446212,3.84481348804514,23.5124112506294));
#44984=CARTESIAN_POINT('Ctrl Pts',(34.3030015747841,3.17343822348752,24.0398050046363));
#44985=CARTESIAN_POINT('Ctrl Pts',(34.349305404947,2.50206295892989,24.5671987586433));
#44986=CARTESIAN_POINT('Ctrl Pts',(34.3956092351099,1.69637395714638,24.9236103571381));
#44987=CARTESIAN_POINT('Ctrl Pts',(34.4419130652727,0.854518027955203,25.0656227231878));
#44988=CARTESIAN_POINT('Ctrl Pts',(34.4882168954356,0.0126620987640046,
25.2076350892374));
#44989=CARTESIAN_POINT('Ctrl Pts',(34.5345207255985,-0.865360757834854,
25.135248222842));
#44990=CARTESIAN_POINT('Ctrl Pts',(34.5808245557613,-1.67259222153178,24.857280092217));
#44991=CARTESIAN_POINT('Ctrl Pts',(34.6271283859242,-2.47982368522869,24.5793119615921));
#44992=CARTESIAN_POINT('Ctrl Pts',(34.6734322160871,-3.21626375602367,24.0957625667378));
#44993=CARTESIAN_POINT('Ctrl Pts',(34.71973604625,-3.79220133768625,23.4655365599323));
#44994=CARTESIAN_POINT('Ctrl Pts',(34.7660398764129,-4.36813891934883,22.8353105531268));
#44995=CARTESIAN_POINT('Ctrl Pts',(34.8123437065758,-4.78357401187901,22.0584079343701));
#44996=CARTESIAN_POINT('Ctrl Pts',(34.8586475367386,-4.98789945925489,21.2294688357748));
#44997=CARTESIAN_POINT('Ctrl Pts',(34.8810845227247,-5.08690740704766,20.8277980695969));
#44998=CARTESIAN_POINT('Ctrl Pts',(34.9035215087108,-5.13634714026073,20.41390921932));
#44999=CARTESIAN_POINT('Ctrl Pts',(34.9259584946969,-5.13631268534711,20.0000122781576));
#45000=CARTESIAN_POINT('Origin',(25.,0.,20.));
#45001=CARTESIAN_POINT('',(36.6759584946969,-5.13711172348184,20.0000703967194));
#45002=CARTESIAN_POINT('',(36.1990415053031,-5.1363684901921,19.9999311527925));
#45003=CARTESIAN_POINT('',(25.,-5.13675,20.));
#45004=CARTESIAN_POINT('Ctrl Pts',(36.1990415053031,-5.1363684901921,19.9999311527925));
#45005=CARTESIAN_POINT('Ctrl Pts',(36.1716901792172,-5.13612980667983,20.5044676422258));
#45006=CARTESIAN_POINT('Ctrl Pts',(36.1443388531313,-5.06229487396435,21.0090724832292));
#45007=CARTESIAN_POINT('Ctrl Pts',(36.1169875270455,-4.91586386075298,21.4916490745987));
#45008=CARTESIAN_POINT('Ctrl Pts',(36.0706836968826,-4.66796667488968,22.3086165758158));
#45009=CARTESIAN_POINT('Ctrl Pts',(36.0243798667197,-4.21200870437187,23.0624509867601));
#45010=CARTESIAN_POINT('Ctrl Pts',(35.9780760365568,-3.60353349034068,23.661322280707));
#45011=CARTESIAN_POINT('Ctrl Pts',(35.931772206394,-2.99505827630949,24.2601935746539));
#45012=CARTESIAN_POINT('Ctrl Pts',(35.8854683762311,-2.23406581876493,24.7041017516034));
#45013=CARTESIAN_POINT('Ctrl Pts',(35.8391645460682,-1.41325811790606,24.9389711429994));
#45014=CARTESIAN_POINT('Ctrl Pts',(35.7928607159053,-0.592450417047175,
25.1738405343954));
#45015=CARTESIAN_POINT('Ctrl Pts',(35.7465568857425,0.288172527126009,25.1996711402378));
#45016=CARTESIAN_POINT('Ctrl Pts',(35.7002530555796,1.12133565881403,25.0133163474371));
#45017=CARTESIAN_POINT('Ctrl Pts',(35.6539492254167,1.95449879050203,24.8269615546364));
#45018=CARTESIAN_POINT('Ctrl Pts',(35.6076453952538,2.74020210970485,24.4284213631927));
#45019=CARTESIAN_POINT('Ctrl Pts',(35.5613415650909,3.38273340727898,23.8662448389215));
#45020=CARTESIAN_POINT('Ctrl Pts',(35.515037734928,4.02526470485311,23.3040683146503));
#45021=CARTESIAN_POINT('Ctrl Pts',(35.4687339047652,4.52462398079854,22.5782554575517));
#45022=CARTESIAN_POINT('Ctrl Pts',(35.4224300746023,4.81998066677103,21.7772227860237));
#45023=CARTESIAN_POINT('Ctrl Pts',(35.3761262444394,5.11533735274352,20.9761901144957));
#45024=CARTESIAN_POINT('Ctrl Pts',(35.3298224142765,5.20669144874308,20.0999376285383));
#45025=CARTESIAN_POINT('Ctrl Pts',(35.2835185841136,5.08291445100915,19.2552079867973));
#45026=CARTESIAN_POINT('Ctrl Pts',(35.2372147539508,4.95913745327523,18.4104783450563));
#45027=CARTESIAN_POINT('Ctrl Pts',(35.1909109237879,4.62022936180781,17.5972715475316));
#45028=CARTESIAN_POINT('Ctrl Pts',(35.144607093625,4.1074750246382,16.9146502011633));
#45029=CARTESIAN_POINT('Ctrl Pts',(35.0983032634622,3.59472068746857,16.232028854795));
#45030=CARTESIAN_POINT('Ctrl Pts',(35.0519994332993,2.90812010459674,15.679992959583));
#45031=CARTESIAN_POINT('Ctrl Pts',(35.0056956031364,2.13131306343327,15.3257900041989));
#45032=CARTESIAN_POINT('Ctrl Pts',(34.9593917729735,1.3545060222698,14.9715870488148));
#45033=CARTESIAN_POINT('Ctrl Pts',(34.9130879428106,0.487492522814696,14.8152170332586));
#45034=CARTESIAN_POINT('Ctrl Pts',(34.8667841126478,-0.364110244114622,
14.8757285211126));
#45035=CARTESIAN_POINT('Ctrl Pts',(34.8204802824849,-1.21571301104392,14.9362400089666));
#45036=CARTESIAN_POINT('Ctrl Pts',(34.774176452322,-2.05190504544742,15.2136330002308));
#45037=CARTESIAN_POINT('Ctrl Pts',(34.7278726221591,-2.77082374228716,15.6741162465473));
#45038=CARTESIAN_POINT('Ctrl Pts',(34.6815687919962,-3.48974243912691,16.1345994928638));
#45039=CARTESIAN_POINT('Ctrl Pts',(34.6352649618334,-4.09138779840288,16.7781729942326));
#45040=CARTESIAN_POINT('Ctrl Pts',(34.5889611316705,-4.50246904349511,17.5264384035209));
#45041=CARTESIAN_POINT('Ctrl Pts',(34.5426573015076,-4.91355028858735,18.2747038128091));
#45042=CARTESIAN_POINT('Ctrl Pts',(34.4963534713447,-5.13406741949585,19.1276611300169));
#45043=CARTESIAN_POINT('Ctrl Pts',(34.4500496411818,-5.13715764814602,19.9814054496412));
#45044=CARTESIAN_POINT('Ctrl Pts',(34.4497135958889,-5.13718007516315,19.9876014113782));
#45045=CARTESIAN_POINT('Ctrl Pts',(34.449377550596,-5.13719105034537,19.9937974145664));
#45046=CARTESIAN_POINT('Ctrl Pts',(34.4490415053031,-5.13719058367308,19.9999934194154));
#45047=CARTESIAN_POINT('Ctrl Pts',(34.9259584946969,-5.13631268534711,20.0000122781576));
#45048=CARTESIAN_POINT('Ctrl Pts',(34.9498253388737,-5.13627603470006,19.5597386243741));
#45049=CARTESIAN_POINT('Ctrl Pts',(34.9736921830504,-5.08025851475436,19.1194558156187));
#45050=CARTESIAN_POINT('Ctrl Pts',(34.9975590272272,-4.96837329816293,18.6938601132045));
#45051=CARTESIAN_POINT('Ctrl Pts',(35.0438628573901,-4.75130588747351,17.8681660676634));
#45052=CARTESIAN_POINT('Ctrl Pts',(35.090166687553,-4.32395526387306,17.0977535550153));
#45053=CARTESIAN_POINT('Ctrl Pts',(35.1364705177159,-3.73838010048158,16.4764721005646));
#45054=CARTESIAN_POINT('Ctrl Pts',(35.1827743478788,-3.15280493709009,15.8551906461138));
#45055=CARTESIAN_POINT('Ctrl Pts',(35.2290781780417,-2.40900523390756,15.3830402498605));
#45056=CARTESIAN_POINT('Ctrl Pts',(35.2753820082046,-1.59758861726315,15.1175369695442));
#45057=CARTESIAN_POINT('Ctrl Pts',(35.3216858383674,-0.786172000618762,
14.8520336892278));
#45058=CARTESIAN_POINT('Ctrl Pts',(35.3679896685303,0.0928615294875015,
14.7931775248485));
#45059=CARTESIAN_POINT('Ctrl Pts',(35.4142934986932,0.932430535289689,14.9481381718582));
#45060=CARTESIAN_POINT('Ctrl Pts',(35.460597328856,1.77199954109188,15.103098818868));
#45061=CARTESIAN_POINT('Ctrl Pts',(35.5069011590189,2.57210402259,15.4718762772669));
#45062=CARTESIAN_POINT('Ctrl Pts',(35.5532049891818,3.235277460809,16.0095470952086));
#45063=CARTESIAN_POINT('Ctrl Pts',(35.5995088193447,3.89845089902802,16.5472179131504));
#45064=CARTESIAN_POINT('Ctrl Pts',(35.6458126495076,4.4246932939679,17.2537820906349));
#45065=CARTESIAN_POINT('Ctrl Pts',(35.6921164796704,4.74989924994857,18.0431679302723));
#45066=CARTESIAN_POINT('Ctrl Pts',(35.7384203098333,5.07510520592925,18.8325537699098));
#45067=CARTESIAN_POINT('Ctrl Pts',(35.7847241399962,5.19927472295068,19.7047612717001));
#45068=CARTESIAN_POINT('Ctrl Pts',(35.8310279701591,5.10728181326158,20.5535405258011));
#45069=CARTESIAN_POINT('Ctrl Pts',(35.877331800322,5.01528890357248,21.4023197799021));
#45070=CARTESIAN_POINT('Ctrl Pts',(35.9236356304849,4.70713356717287,22.2276707863139));
#45071=CARTESIAN_POINT('Ctrl Pts',(35.9699394606477,4.22035443637511,22.9290515640981));
#45072=CARTESIAN_POINT('Ctrl Pts',(36.0162432908106,3.73357530557736,23.6304323418823));
#45073=CARTESIAN_POINT('Ctrl Pts',(36.0625471209735,3.06817238038148,24.2078428910389));
#45074=CARTESIAN_POINT('Ctrl Pts',(36.1088509511364,2.30520320806331,24.5909446526081));
#45075=CARTESIAN_POINT('Ctrl Pts',(36.1551547812992,1.54223403574514,24.9740464141774));
#45076=CARTESIAN_POINT('Ctrl Pts',(36.2014586114621,0.681698616304682,25.1628393881594));
#45077=CARTESIAN_POINT('Ctrl Pts',(36.247762441625,-0.171575001263084,25.134325335691));
#45078=CARTESIAN_POINT('Ctrl Pts',(36.2940662717879,-1.02484861883088,25.1058112832225));
#45079=CARTESIAN_POINT('Ctrl Pts',(36.3403701019507,-1.87086043452598,24.8599902043036));
#45080=CARTESIAN_POINT('Ctrl Pts',(36.3866739321136,-2.60655162466432,24.4268073440954));
#45081=CARTESIAN_POINT('Ctrl Pts',(36.4329777622765,-3.34224281480263,23.9936244838871));
#45082=CARTESIAN_POINT('Ctrl Pts',(36.4792815924394,-3.96761337938419,23.3730798423894));
#45083=CARTESIAN_POINT('Ctrl Pts',(36.5255854226023,-4.4064824027802,22.6407664546046));
#45084=CARTESIAN_POINT('Ctrl Pts',(36.5718892527651,-4.84535142617622,21.9084530668199));
#45085=CARTESIAN_POINT('Ctrl Pts',(36.618193082928,-5.09771890838669,21.064370932748));
#45086=CARTESIAN_POINT('Ctrl Pts',(36.6644969130909,-5.13284213947516,20.2113438075854));
#45087=CARTESIAN_POINT('Ctrl Pts',(36.6683174402929,-5.13574015588813,20.1409605731045));
#45088=CARTESIAN_POINT('Ctrl Pts',(36.6721379674949,-5.13715919655493,20.0705164420761));
#45089=CARTESIAN_POINT('Ctrl Pts',(36.6759584946969,-5.13711172348184,20.0000703967194));
#45090=CARTESIAN_POINT('Origin',(25.,0.,20.));
#45091=CARTESIAN_POINT('',(38.4259584946969,-5.13652713961075,19.9998820685162));
#45092=CARTESIAN_POINT('',(37.9490415053031,-5.13686389810347,20.0001263479959));
#45093=CARTESIAN_POINT('',(25.,-5.13675,20.));
#45094=CARTESIAN_POINT('Ctrl Pts',(37.9490415053031,-5.13686389810347,20.0001263479959));
#45095=CARTESIAN_POINT('Ctrl Pts',(37.9403066380013,-5.13702848944412,20.1612095334366));
#45096=CARTESIAN_POINT('Ctrl Pts',(37.9315717706995,-5.12960133194211,20.3222776015441));
#45097=CARTESIAN_POINT('Ctrl Pts',(37.9228369033977,-5.11447099711345,20.4826187717999));
#45098=CARTESIAN_POINT('Ctrl Pts',(37.8765330732349,-5.03426457496541,21.3325927964913));
#45099=CARTESIAN_POINT('Ctrl Pts',(37.830229243072,-4.73759144851179,22.1621402912393));
#45100=CARTESIAN_POINT('Ctrl Pts',(37.7839254129091,-4.26059151894989,22.8702080704821));
#45101=CARTESIAN_POINT('Ctrl Pts',(37.7376215827462,-3.78359158938799,23.5782758497249));
#45102=CARTESIAN_POINT('Ctrl Pts',(37.6913177525833,-3.12626485671779,24.1648639134627));
#45103=CARTESIAN_POINT('Ctrl Pts',(37.6450139224205,-2.36868504873878,24.5585157232469));
#45104=CARTESIAN_POINT('Ctrl Pts',(37.5987100922576,-1.61110524075978,24.9521675330312));
#45105=CARTESIAN_POINT('Ctrl Pts',(37.5524062620947,-0.753272357471954,
25.1528830888621));
#45106=CARTESIAN_POINT('Ctrl Pts',(37.5061024319319,0.100314767622557,25.1362117758719));
#45107=CARTESIAN_POINT('Ctrl Pts',(37.459798601769,0.953901892717081,25.1195404628817));
#45108=CARTESIAN_POINT('Ctrl Pts',(37.4134947716061,1.80324325961826,24.8854822810705));
#45109=CARTESIAN_POINT('Ctrl Pts',(37.3671909414432,2.54487444790653,24.4625495519491));
#45110=CARTESIAN_POINT('Ctrl Pts',(37.3208871112803,3.28650563619479,24.0396168228276));
#45111=CARTESIAN_POINT('Ctrl Pts',(37.2745832811174,3.92042664587011,23.427809546396));
#45112=CARTESIAN_POINT('Ctrl Pts',(37.2282794509546,4.36941496968878,22.7016563959667));
#45113=CARTESIAN_POINT('Ctrl Pts',(37.1819756207917,4.81840329350746,21.9755032455374));
#45114=CARTESIAN_POINT('Ctrl Pts',(37.1356717906288,5.08245893146949,21.1350042211103));
#45115=CARTESIAN_POINT('Ctrl Pts',(37.0893679604659,5.12941535477392,20.2825465933572));
#45116=CARTESIAN_POINT('Ctrl Pts',(37.0430641303031,5.17637177807835,19.4300889656041));
#45117=CARTESIAN_POINT('Ctrl Pts',(36.9967603001402,5.00622898672518,18.5656727345251));
#45118=CARTESIAN_POINT('Ctrl Pts',(36.9504564699773,4.6397133058199,17.7945986988745));
#45119=CARTESIAN_POINT('Ctrl Pts',(36.9041526398144,4.27319762491461,17.0235246632239));
#45120=CARTESIAN_POINT('Ctrl Pts',(36.8578488096515,3.71030905445721,16.3457928230018));
#45121=CARTESIAN_POINT('Ctrl Pts',(36.8115449794886,3.0196171260551,15.8439625998744));
#45122=CARTESIAN_POINT('Ctrl Pts',(36.7652411493258,2.328925197653,15.3421323767469));
#45123=CARTESIAN_POINT('Ctrl Pts',(36.7189373191629,1.51042991130619,15.0162037707142));
#45124=CARTESIAN_POINT('Ctrl Pts',(36.672633489,0.663838103062301,14.905880504726));
#45125=CARTESIAN_POINT('Ctrl Pts',(36.6263296588372,-0.182753705181584,
14.7955572387378));
#45126=CARTESIAN_POINT('Ctrl Pts',(36.5800258286743,-1.05744203532252,14.9008393127942));
#45127=CARTESIAN_POINT('Ctrl Pts',(36.5337219985114,-1.85367476985798,15.2089015553007));
#45128=CARTESIAN_POINT('Ctrl Pts',(36.4874181683485,-2.64990750439343,15.5169637978072));
#45129=CARTESIAN_POINT('Ctrl Pts',(36.4411143381856,-3.36768464332339,16.0278062087637));
#45130=CARTESIAN_POINT('Ctrl Pts',(36.3948105080228,-3.91956855725179,16.6791993760222));
#45131=CARTESIAN_POINT('Ctrl Pts',(36.3485066778599,-4.47145247118018,17.3305925432806));
#45132=CARTESIAN_POINT('Ctrl Pts',(36.302202847697,-4.85744316010701,18.122536466841));
#45133=CARTESIAN_POINT('Ctrl Pts',(36.2558990175341,-5.03052030396604,18.9585587243662));
#45134=CARTESIAN_POINT('Ctrl Pts',(36.2369465134571,-5.10136207370919,19.3007488885163));
#45135=CARTESIAN_POINT('Ctrl Pts',(36.2179940093801,-5.13653388071924,19.6503236111705));
#45136=CARTESIAN_POINT('Ctrl Pts',(36.1990415053031,-5.1363684901921,19.9999311527925));
#45137=CARTESIAN_POINT('Ctrl Pts',(36.6759584946969,-5.13711172348184,20.0000703967194));
#45138=CARTESIAN_POINT('Ctrl Pts',(36.7184417976577,-5.13658383483194,19.2167280648719));
#45139=CARTESIAN_POINT('Ctrl Pts',(36.7609251006186,-4.9547232608138,18.4331490285896));
#45140=CARTESIAN_POINT('Ctrl Pts',(36.8034084035795,-4.60866455922797,17.7304305222592));
#45141=CARTESIAN_POINT('Ctrl Pts',(36.8497122337424,-4.23148476792581,16.9645164783491));
#45142=CARTESIAN_POINT('Ctrl Pts',(36.8960160639053,-3.659246205355,16.2946605067825));
#45143=CARTESIAN_POINT('Ctrl Pts',(36.9423198940682,-2.96165739334837,15.8024626126499));
#45144=CARTESIAN_POINT('Ctrl Pts',(36.9886237242311,-2.26406858134175,15.3102647185174));
#45145=CARTESIAN_POINT('Ctrl Pts',(37.0349275543939,-1.44112951989932,14.9957249018188));
#45146=CARTESIAN_POINT('Ctrl Pts',(37.0812313845568,-0.593088373482288,
14.8971595346301));
#45147=CARTESIAN_POINT('Ctrl Pts',(37.1275352147197,0.254952772934734,14.7985941674414));
#45148=CARTESIAN_POINT('Ctrl Pts',(37.1738390448826,1.12809600432639,14.9160032497626));
#45149=CARTESIAN_POINT('Ctrl Pts',(37.2201428750454,1.91997742285391,15.235084331333));
#45150=CARTESIAN_POINT('Ctrl Pts',(37.2664467052083,2.71185884138146,15.5541654129035));
#45151=CARTESIAN_POINT('Ctrl Pts',(37.3127505353712,3.42247844704487,16.0749184937233));
#45152=CARTESIAN_POINT('Ctrl Pts',(37.3590543655341,3.96527052138986,16.7339068712033));
#45153=CARTESIAN_POINT('Ctrl Pts',(37.4053581956969,4.50806259573483,17.3928952486832));
#45154=CARTESIAN_POINT('Ctrl Pts',(37.4516620258598,4.88302713876135,18.1901189228233));
#45155=CARTESIAN_POINT('Ctrl Pts',(37.4979658560227,5.04448700505531,19.0284623066475));
#45156=CARTESIAN_POINT('Ctrl Pts',(37.5442696861856,5.20594687134927,19.8668056904716));
#45157=CARTESIAN_POINT('Ctrl Pts',(37.5905735163485,5.15390206091068,20.7462687839798));
#45158=CARTESIAN_POINT('Ctrl Pts',(37.6368773465114,4.89469252885972,21.5597178211784));
#45159=CARTESIAN_POINT('Ctrl Pts',(37.6831811766742,4.63548299680876,22.373166858377));
#45160=CARTESIAN_POINT('Ctrl Pts',(37.7294850068371,4.16910874314546,23.120601839266));
#45161=CARTESIAN_POINT('Ctrl Pts',(37.775788837,3.55238219186601,23.7109722980224));
#45162=CARTESIAN_POINT('Ctrl Pts',(37.8220926671629,2.93565564058657,24.3013427567789));
#45163=CARTESIAN_POINT('Ctrl Pts',(37.8683964973257,2.16857679169099,24.7346486934028));
#45164=CARTESIAN_POINT('Ctrl Pts',(37.9147003274886,1.34458907276917,24.9581059749834));
#45165=CARTESIAN_POINT('Ctrl Pts',(37.9610041576515,0.520601353847358,25.181563256564));
#45166=CARTESIAN_POINT('Ctrl Pts',(38.0073079878144,-0.360295235100682,
25.1951718831012));
#45167=CARTESIAN_POINT('Ctrl Pts',(38.0536118179773,-1.19079230362451,24.9972740892816));
#45168=CARTESIAN_POINT('Ctrl Pts',(38.0999156481402,-2.02128937214836,24.7993762954619));
#45169=CARTESIAN_POINT('Ctrl Pts',(38.146219478303,-2.80138692024799,24.3899720812854));
#45170=CARTESIAN_POINT('Ctrl Pts',(38.1925233084659,-3.43605561833901,23.8189339378232));
#45171=CARTESIAN_POINT('Ctrl Pts',(38.2388271386288,-4.07072431643002,23.2478957943609));
#45172=CARTESIAN_POINT('Ctrl Pts',(38.2851309687917,-4.55996416451244,22.5152237216129));
#45173=CARTESIAN_POINT('Ctrl Pts',(38.3314347989545,-4.84417731500616,21.7101698086905));
#45174=CARTESIAN_POINT('Ctrl Pts',(38.3629426975353,-5.03757296045447,21.1623629220638));
#45175=CARTESIAN_POINT('Ctrl Pts',(38.3944505961161,-5.136035987151,20.5810413872539));
#45176=CARTESIAN_POINT('Ctrl Pts',(38.4259584946969,-5.13652713961075,19.9998820685162));
#45177=CARTESIAN_POINT('Origin',(25.,0.,20.));
#45178=CARTESIAN_POINT('',(40.1759584946969,-5.13662507615807,20.0001297408024));
#45179=CARTESIAN_POINT('',(39.6990415053031,-5.13679701019626,19.9998685352764));
#45180=CARTESIAN_POINT('',(25.,-5.13675,20.));
#45181=CARTESIAN_POINT('Ctrl Pts',(39.6990415053031,-5.13679701019626,19.9998685352764));
#45182=CARTESIAN_POINT('Ctrl Pts',(39.6626192666225,-5.13610342108661,20.671570825383));
#45183=CARTESIAN_POINT('Ctrl Pts',(39.626197027942,-5.00366088383949,21.3435385570443));
#45184=CARTESIAN_POINT('Ctrl Pts',(39.5897747892614,-4.74690985169674,21.9640726358953));
#45185=CARTESIAN_POINT('Ctrl Pts',(39.5434709590985,-4.42050058589771,22.7529616673848));
#45186=CARTESIAN_POINT('Ctrl Pts',(39.4971671289356,-3.89318140550294,23.4587225844028));
#45187=CARTESIAN_POINT('Ctrl Pts',(39.4508632987728,-3.22918887722381,23.9953815405318));
#45188=CARTESIAN_POINT('Ctrl Pts',(39.4045594686099,-2.56519634894465,24.5320404966608));
#45189=CARTESIAN_POINT('Ctrl Pts',(39.358255638447,-1.76453047278113,24.8995974919006));
#45190=CARTESIAN_POINT('Ctrl Pts',(39.3119518082841,-0.924726155256508,
25.0532777478576));
#45191=CARTESIAN_POINT('Ctrl Pts',(39.2656479781212,-0.0849218377319214,
25.2069580038146));
#45192=CARTESIAN_POINT('Ctrl Pts',(39.2193441479584,0.794020921153764,25.1467615204886));
#45193=CARTESIAN_POINT('Ctrl Pts',(39.1730403177955,1.60503174113409,24.8800212672857));
#45194=CARTESIAN_POINT('Ctrl Pts',(39.1267364876326,2.41604256111441,24.6132810140827));
#45195=CARTESIAN_POINT('Ctrl Pts',(39.0804326574697,3.15912144218937,24.1399969910027));
#45196=CARTESIAN_POINT('Ctrl Pts',(39.0341288273068,3.74374856658888,23.5178233510755));
#45197=CARTESIAN_POINT('Ctrl Pts',(38.987824997144,4.32837569098839,22.8956497111483));
#45198=CARTESIAN_POINT('Ctrl Pts',(38.9415211669811,4.75455105871245,22.1245864543738));
#45199=CARTESIAN_POINT('Ctrl Pts',(38.8952173368182,4.97035916306724,21.2985623779094));
#45200=CARTESIAN_POINT('Ctrl Pts',(38.8489135066553,5.18616726742202,20.4725383014451));
#45201=CARTESIAN_POINT('Ctrl Pts',(38.8026096764924,5.19160810840753,19.5915534052909));
#45202=CARTESIAN_POINT('Ctrl Pts',(38.7563058463296,4.9860188977962,18.7629268372374));
#45203=CARTESIAN_POINT('Ctrl Pts',(38.7100020161667,4.78042968718488,17.9343002691839));
#45204=CARTESIAN_POINT('Ctrl Pts',(38.6636981860038,4.36381042497672,17.158032029231));
#45205=CARTESIAN_POINT('Ctrl Pts',(38.6173943558409,3.78691251947449,16.5286849712169));
#45206=CARTESIAN_POINT('Ctrl Pts',(38.5710905256781,3.21001461397227,15.8993379132027));
#45207=CARTESIAN_POINT('Ctrl Pts',(38.5247866955152,2.47283806517597,15.4169120371273));
#45208=CARTESIAN_POINT('Ctrl Pts',(38.4784828653523,1.6651836850329,15.140175131313));
#45209=CARTESIAN_POINT('Ctrl Pts',(38.4321790351894,0.857529304889817,14.8634382254988));
#45210=CARTESIAN_POINT('Ctrl Pts',(38.3858752050266,-0.0206029066000382,
14.7923902899457));
#45211=CARTESIAN_POINT('Ctrl Pts',(38.3395713748637,-0.862241307816169,
14.9356861880109));
#45212=CARTESIAN_POINT('Ctrl Pts',(38.2932675447008,-1.70387970903231,15.0789820860761));
#45213=CARTESIAN_POINT('Ctrl Pts',(38.2469637145379,-2.50902429997473,15.4366218177595));
#45214=CARTESIAN_POINT('Ctrl Pts',(38.200659884375,-3.17959458945082,15.9650386983339));
#45215=CARTESIAN_POINT('Ctrl Pts',(38.1543560542121,-3.85016487892688,16.4934555789082));
#45216=CARTESIAN_POINT('Ctrl Pts',(38.1080522240493,-4.38616086693662,17.1926496083734));
#45217=CARTESIAN_POINT('Ctrl Pts',(38.0617483938864,-4.72228900202028,17.9774469004235));
#45218=CARTESIAN_POINT('Ctrl Pts',(38.0241794310253,-4.99500910701175,18.6141981198108));
#45219=CARTESIAN_POINT('Ctrl Pts',(37.9866104681642,-5.1361559851209,19.3073020608843));
#45220=CARTESIAN_POINT('Ctrl Pts',(37.9490415053031,-5.13686389810347,20.0001263479959));
#45221=CARTESIAN_POINT('Ctrl Pts',(38.4259584946969,-5.13652713961075,19.9998820685162));
#45222=CARTESIAN_POINT('Ctrl Pts',(38.440754426279,-5.13675778203751,19.726972928089));
#45223=CARTESIAN_POINT('Ctrl Pts',(38.4555503578611,-5.11538377782675,19.4540995593661));
#45224=CARTESIAN_POINT('Ctrl Pts',(38.4703462894432,-5.07209039864956,19.1847493503814));
#45225=CARTESIAN_POINT('Ctrl Pts',(38.516650119606,-4.9366038788942,18.3418185580918));
#45226=CARTESIAN_POINT('Ctrl Pts',(38.5629539497689,-4.58644438647845,17.5333927266096));
#45227=CARTESIAN_POINT('Ctrl Pts',(38.6092577799318,-4.0642673840338,16.857952058791));
#45228=CARTESIAN_POINT('Ctrl Pts',(38.6555616100947,-3.54209038158914,16.1825113909724));
#45229=CARTESIAN_POINT('Ctrl Pts',(38.7018654402576,-2.84789586911556,15.6400558868173));
#45230=CARTESIAN_POINT('Ctrl Pts',(38.7481692704204,-2.06624870556211,15.2966659782087));
#45231=CARTESIAN_POINT('Ctrl Pts',(38.7944731005833,-1.28460154200866,14.9532760696001));
#45232=CARTESIAN_POINT('Ctrl Pts',(38.8407769307462,-0.415501727375322,
14.808951756538));
#45233=CARTESIAN_POINT('Ctrl Pts',(38.8870807609091,0.43517939836545,14.8812742283831));
#45234=CARTESIAN_POINT('Ctrl Pts',(38.933384591072,1.28586052410621,14.9535967002282));
#45235=CARTESIAN_POINT('Ctrl Pts',(38.9796884212348,2.11812296095441,15.2425659569806));
#45236=CARTESIAN_POINT('Ctrl Pts',(39.0259922513977,2.83058279659726,15.7129805615808));
#45237=CARTESIAN_POINT('Ctrl Pts',(39.0722960815606,3.54304263224011,16.1833951661809));
#45238=CARTESIAN_POINT('Ctrl Pts',(39.1185999117235,4.13569986667761,16.8352551186289));
#45239=CARTESIAN_POINT('Ctrl Pts',(39.1649037418864,4.53635863184284,17.5891526391989));
#45240=CARTESIAN_POINT('Ctrl Pts',(39.2112075720492,4.93701739700806,18.3430501597689));
#45241=CARTESIAN_POINT('Ctrl Pts',(39.2575114022121,5.145677692901,19.198985248461));
#45242=CARTESIAN_POINT('Ctrl Pts',(39.303815232375,5.13692109835384,20.0526902558713));
#45243=CARTESIAN_POINT('Ctrl Pts',(39.3501190625379,5.12816450380669,20.9063952632815));
#45244=CARTESIAN_POINT('Ctrl Pts',(39.3964228927008,4.90199101881941,21.7578701894099));
#45245=CARTESIAN_POINT('Ctrl Pts',(39.4427267228636,4.48595247290419,22.503390709542));
#45246=CARTESIAN_POINT('Ctrl Pts',(39.4890305530265,4.06991392698898,23.2489112296742));
#45247=CARTESIAN_POINT('Ctrl Pts',(39.5353343831894,3.46401032014584,23.8884773438102));
#45248=CARTESIAN_POINT('Ctrl Pts',(39.5816382133523,2.74205115695702,24.3441788736662));
#45249=CARTESIAN_POINT('Ctrl Pts',(39.6279420435151,2.02009199376821,24.7998804035221));
#45250=CARTESIAN_POINT('Ctrl Pts',(39.674245873678,1.18207727423371,25.071717349098));
#45251=CARTESIAN_POINT('Ctrl Pts',(39.7205497038409,0.330091637862047,25.1265752841824));
#45252=CARTESIAN_POINT('Ctrl Pts',(39.7668535340038,-0.52189399850962,25.1814332192668));
#45253=CARTESIAN_POINT('Ctrl Pts',(39.8131573641667,-1.38785055171847,25.0193121438596));
#45254=CARTESIAN_POINT('Ctrl Pts',(39.8594611943296,-2.16228958522074,24.6599611997765));
#45255=CARTESIAN_POINT('Ctrl Pts',(39.9057650244924,-2.93672861872303,24.3006102556934));
#45256=CARTESIAN_POINT('Ctrl Pts',(39.9520688546553,-3.61965013251875,23.7440294429343));
#45257=CARTESIAN_POINT('Ctrl Pts',(39.9983726848182,-4.12786251323483,23.0580198994786));
#45258=CARTESIAN_POINT('Ctrl Pts',(40.044676514981,-4.6360748939509,22.3720103560229));
#45259=CARTESIAN_POINT('Ctrl Pts',(40.0909803451439,-4.96957814158735,21.5565720818707));
#45260=CARTESIAN_POINT('Ctrl Pts',(40.1372841753068,-5.08774581126648,20.7110395162838));
#45261=CARTESIAN_POINT('Ctrl Pts',(40.1501756151035,-5.1206448477873,20.4756349692505));
#45262=CARTESIAN_POINT('Ctrl Pts',(40.1630670549002,-5.13685279015782,20.2378977531038));
#45263=CARTESIAN_POINT('Ctrl Pts',(40.1759584946969,-5.13662507615807,20.0001297408024));
#45264=CARTESIAN_POINT('Origin',(25.,0.,20.));
#45265=CARTESIAN_POINT('',(41.9259584946969,-5.13702782547439,19.9999018799691));
#45266=CARTESIAN_POINT('',(41.4490415053031,-5.13640319548555,20.0000850263462));
#45267=CARTESIAN_POINT('',(25.,-5.13675,20.));
#45268=CARTESIAN_POINT('Ctrl Pts',(41.4490415053031,-5.13640319548555,20.0000850263462));
#45269=CARTESIAN_POINT('Ctrl Pts',(41.4312357254066,-5.13659675996406,20.3285331564035));
#45270=CARTESIAN_POINT('Ctrl Pts',(41.4134299455101,-5.10557932918625,20.6569451919344));
#45271=CARTESIAN_POINT('Ctrl Pts',(41.3956241656136,-5.0429996819552,20.9792286081442));
#45272=CARTESIAN_POINT('Ctrl Pts',(41.3493203354508,-4.88026166239715,21.8173248137163));
#45273=CARTESIAN_POINT('Ctrl Pts',(41.3030165052879,-4.50408191610273,22.613975796569));
#45274=CARTESIAN_POINT('Ctrl Pts',(41.2567126751251,-3.96028562119314,23.2721357333979));
#45275=CARTESIAN_POINT('Ctrl Pts',(41.2104088449622,-3.41648932628355,23.9302956702267));
#45276=CARTESIAN_POINT('Ctrl Pts',(41.1641050147993,-2.70507648275881,24.4499645610316));
#45277=CARTESIAN_POINT('Ctrl Pts',(41.1178011846364,-1.91270943911951,24.7678377762578));
#45278=CARTESIAN_POINT('Ctrl Pts',(41.0714973544735,-1.12034239548021,25.0857109914841));
#45279=CARTESIAN_POINT('Ctrl Pts',(41.0251935243106,-0.247021151726365,
25.2017885311316));
#45280=CARTESIAN_POINT('Ctrl Pts',(40.9788896941478,0.600868709328828,25.1019301497921));
#45281=CARTESIAN_POINT('Ctrl Pts',(40.9325858639849,1.44875857038403,25.0020717684527));
#45282=CARTESIAN_POINT('Ctrl Pts',(40.886282033822,2.27121704874058,24.6862774661262));
#45283=CARTESIAN_POINT('Ctrl Pts',(40.8399782036591,2.96805452324197,24.1930164328644));
#45284=CARTESIAN_POINT('Ctrl Pts',(40.7936743734962,3.66489199774336,23.6997553996026));
#45285=CARTESIAN_POINT('Ctrl Pts',(40.7473705433334,4.23610846838958,23.0290276354055));
#45286=CARTESIAN_POINT('Ctrl Pts',(40.7010667131705,4.61211992176423,22.262539344735));
#45287=CARTESIAN_POINT('Ctrl Pts',(40.6547628830076,4.98813137513887,21.4960510540645));
#45288=CARTESIAN_POINT('Ctrl Pts',(40.6084590528447,5.16893781124195,20.6338022369205));
#45289=CARTESIAN_POINT('Ctrl Pts',(40.5621552226818,5.13251388920516,19.780829663676));
#45290=CARTESIAN_POINT('Ctrl Pts',(40.5158513925189,5.09608996716837,18.9278570904315));
#45291=CARTESIAN_POINT('Ctrl Pts',(40.4695475623561,4.84243568699171,18.0841607610863));
#45292=CARTESIAN_POINT('Ctrl Pts',(40.4232437321932,4.40245051278724,17.3525174331702));
#45293=CARTESIAN_POINT('Ctrl Pts',(40.3769399020303,3.96246533858275,16.6208741052541));
#45294=CARTESIAN_POINT('Ctrl Pts',(40.3306360718675,3.33614927035045,16.0012837787669));
#45295=CARTESIAN_POINT('Ctrl Pts',(40.2843322417046,2.59979840236344,15.5692232366912));
#45296=CARTESIAN_POINT('Ctrl Pts',(40.2380284115417,1.86344753437645,15.1371626946156));
#45297=CARTESIAN_POINT('Ctrl Pts',(40.1917245813788,1.01706186663476,14.8926319369513));
#45298=CARTESIAN_POINT('Ctrl Pts',(40.1454207512159,0.163745764446629,14.8654190254867));
#45299=CARTESIAN_POINT('Ctrl Pts',(40.099116921053,-0.689570337741517,14.8382061140221));
#45300=CARTESIAN_POINT('Ctrl Pts',(40.0528130908902,-1.54981687437611,15.028311048757));
#45301=CARTESIAN_POINT('Ctrl Pts',(40.0065092607273,-2.31220098736803,15.4125757713917));
#45302=CARTESIAN_POINT('Ctrl Pts',(39.9602054305644,-3.07458510035994,15.7968404940263));
#45303=CARTESIAN_POINT('Ctrl Pts',(39.9139016004016,-3.73910678970917,16.3752650045606));
#45304=CARTESIAN_POINT('Ctrl Pts',(39.8675977702387,-4.22481585785777,17.0773872260592));
#45305=CARTESIAN_POINT('Ctrl Pts',(39.8212939400758,-4.71052492600638,17.7795094475579));
#45306=CARTESIAN_POINT('Ctrl Pts',(39.7749901099129,-5.01742137295435,18.6053293800208));
#45307=CARTESIAN_POINT('Ctrl Pts',(39.72868627975,-5.10811992082669,19.4542479192328));
#45308=CARTESIAN_POINT('Ctrl Pts',(39.7188046882677,-5.12747568459311,19.635413627917));
#45309=CARTESIAN_POINT('Ctrl Pts',(39.7089230967854,-5.13698518545639,19.8176313123869));
#45310=CARTESIAN_POINT('Ctrl Pts',(39.6990415053031,-5.13679701019626,19.9998685352764));
#45311=CARTESIAN_POINT('Ctrl Pts',(40.1759584946969,-5.13662507615807,20.0001297408024));
#45312=CARTESIAN_POINT('Ctrl Pts',(40.2093708850631,-5.13603488071278,19.3838760275705));
#45313=CARTESIAN_POINT('Ctrl Pts',(40.2427832754292,-5.02503700210934,18.7674154389927));
#45314=CARTESIAN_POINT('Ctrl Pts',(40.2761956657955,-4.80807881275319,18.1908253914753));
#45315=CARTESIAN_POINT('Ctrl Pts',(40.3224994959583,-4.50741205283897,17.3917706892752));
#45316=CARTESIAN_POINT('Ctrl Pts',(40.3688033261212,-4.00324644128875,16.6692881418965));
#45317=CARTESIAN_POINT('Ctrl Pts',(40.4151071562841,-3.35699804098061,16.1113885786017));
#45318=CARTESIAN_POINT('Ctrl Pts',(40.461410986447,-2.71074964067246,15.5534890153069));
#45319=CARTESIAN_POINT('Ctrl Pts',(40.5077148166099,-1.92241845160638,15.160172436096));
#45320=CARTESIAN_POINT('Ctrl Pts',(40.5540186467727,-1.08803680277753,14.9793515807639));
#45321=CARTESIAN_POINT('Ctrl Pts',(40.6003224769356,-0.253655153948683,
14.7985307254318));
#45322=CARTESIAN_POINT('Ctrl Pts',(40.6466263070985,0.626776954642942,14.8302055939786));
#45323=CARTESIAN_POINT('Ctrl Pts',(40.6929301372614,1.44600771426156,15.0705176413671));
#45324=CARTESIAN_POINT('Ctrl Pts',(40.7392339674242,2.26523847388015,15.3108296887557));
#45325=CARTESIAN_POINT('Ctrl Pts',(40.7855377975871,3.02326788452574,15.759778914986));
#45326=CARTESIAN_POINT('Ctrl Pts',(40.83184162775,3.62775489619198,16.362675564796));
#45327=CARTESIAN_POINT('Ctrl Pts',(40.8781454579129,4.23224190785823,16.9655722146061));
#45328=CARTESIAN_POINT('Ctrl Pts',(40.9244492880757,4.68318652054512,17.7224162879959));
#45329=CARTESIAN_POINT('Ctrl Pts',(40.9707531182386,4.92565590652139,18.541011129471));
#45330=CARTESIAN_POINT('Ctrl Pts',(41.0170569484015,5.16812529249767,19.3596059709461));
#45331=CARTESIAN_POINT('Ctrl Pts',(41.0633607785644,5.20211945176333,20.2399515805066));
#45332=CARTESIAN_POINT('Ctrl Pts',(41.1096646087273,5.0234973096891,21.0748066864897));
#45333=CARTESIAN_POINT('Ctrl Pts',(41.1559684388902,4.84487516761487,21.9096617924729));
#45334=CARTESIAN_POINT('Ctrl Pts',(41.202272269053,4.45363672420075,22.6990263948788));
#45335=CARTESIAN_POINT('Ctrl Pts',(41.2485760992159,3.8974415664764,23.3467422771523));
#45336=CARTESIAN_POINT('Ctrl Pts',(41.2948799293788,3.34124640875205,23.9944581594258));
#45337=CARTESIAN_POINT('Ctrl Pts',(41.3411837595417,2.62009453671747,24.500525321567));
#45338=CARTESIAN_POINT('Ctrl Pts',(41.3874875897045,1.82183468043843,24.8032960590545));
#45339=CARTESIAN_POINT('Ctrl Pts',(41.4337914198674,1.0235748241594,25.106066796542));
#45340=CARTESIAN_POINT('Ctrl Pts',(41.4800952500303,0.148206983635904,25.205541109376));
#45341=CARTESIAN_POINT('Ctrl Pts',(41.5263990801932,-0.697633947550682,
25.0896013113997));
#45342=CARTESIAN_POINT('Ctrl Pts',(41.5727029103561,-1.54347487873726,24.9736615134234));
#45343=CARTESIAN_POINT('Ctrl Pts',(41.6190067405189,-2.35978890058693,24.6423076046368));
#45344=CARTESIAN_POINT('Ctrl Pts',(41.6653105706818,-3.04713489267099,24.135904203393));
#45345=CARTESIAN_POINT('Ctrl Pts',(41.7116144008447,-3.73448088475504,23.6295008021491));
#45346=CARTESIAN_POINT('Ctrl Pts',(41.7579182310076,-4.29285884707349,22.948047908448));
#45347=CARTESIAN_POINT('Ctrl Pts',(41.8042220611704,-4.65424871784935,22.1745582324174));
#45348=CARTESIAN_POINT('Ctrl Pts',(41.8448008723459,-4.97095624021537,21.4967030442091));
#45349=CARTESIAN_POINT('Ctrl Pts',(41.8853796835214,-5.13637565909862,20.7481630235307));
#45350=CARTESIAN_POINT('Ctrl Pts',(41.9259584946969,-5.13702782547439,19.9999018799691));
#45351=CARTESIAN_POINT('Origin',(25.,0.,20.));
#45352=CARTESIAN_POINT('',(43.6759584946968,-5.13631567875976,20.0000203800902));
#45353=CARTESIAN_POINT('',(43.1990415053031,-5.13718721057151,19.9999841637545));
#45354=CARTESIAN_POINT('',(25.,-5.13675,20.));
#45355=CARTESIAN_POINT('Ctrl Pts',(43.1990415053031,-5.13718721057151,19.9999841637545));
#45356=CARTESIAN_POINT('Ctrl Pts',(43.1535483540278,-5.13703940376405,20.8387887285521));
#45357=CARTESIAN_POINT('Ctrl Pts',(43.1080552027526,-4.92745027586239,21.6776644683076));
#45358=CARTESIAN_POINT('Ctrl Pts',(43.0625620514773,-4.53267718080418,22.4177617818605));
#45359=CARTESIAN_POINT('Ctrl Pts',(43.0162582213144,-4.13086930788185,23.1710474820179));
#45360=CARTESIAN_POINT('Ctrl Pts',(42.9699543911515,-3.537218780741,23.822002965617));
#45361=CARTESIAN_POINT('Ctrl Pts',(42.9236505609887,-2.82404246762336,24.2913306328303));
#45362=CARTESIAN_POINT('Ctrl Pts',(42.8773467308258,-2.11086615450573,24.7606583000437));
#45363=CARTESIAN_POINT('Ctrl Pts',(42.8310429006629,-1.27816405541132,25.0483581508711));
#45364=CARTESIAN_POINT('Ctrl Pts',(42.7847390705,-0.427373641093902,25.1193833837784));
#45365=CARTESIAN_POINT('Ctrl Pts',(42.7384352403371,0.423416773223512,25.1904086166857));
#45366=CARTESIAN_POINT('Ctrl Pts',(42.6921314101743,1.29229550276393,25.0447592316728));
#45367=CARTESIAN_POINT('Ctrl Pts',(42.6458275800114,2.07341813953054,24.7001778347073));
#45368=CARTESIAN_POINT('Ctrl Pts',(42.5995237498485,2.85454077629716,24.3555964377418));
#45369=CARTESIAN_POINT('Ctrl Pts',(42.5532199196856,3.54790732028998,23.8120830288236));
#45370=CARTESIAN_POINT('Ctrl Pts',(42.5069160895227,4.0690537733944,23.1358469108732));
#45371=CARTESIAN_POINT('Ctrl Pts',(42.4606122593599,4.59020022649883,22.4596107929228));
#45372=CARTESIAN_POINT('Ctrl Pts',(42.414308429197,4.93912658871485,21.6506519659402));
#45373=CARTESIAN_POINT('Ctrl Pts',(42.3680045990342,5.07332761392745,20.8075155608218));
#45374=CARTESIAN_POINT('Ctrl Pts',(42.3217007688713,5.20752863914005,19.9643791557036));
#45375=CARTESIAN_POINT('Ctrl Pts',(42.2753969387083,5.12700432734922,19.0870651724496));
#45376=CARTESIAN_POINT('Ctrl Pts',(42.2290931085455,4.84156392790253,18.2824455783757));
#45377=CARTESIAN_POINT('Ctrl Pts',(42.1827892783826,4.55612352845583,17.4778259843018));
#45378=CARTESIAN_POINT('Ctrl Pts',(42.1364854482197,4.06576704135327,16.745900779408));
#45379=CARTESIAN_POINT('Ctrl Pts',(42.0901816180569,3.43022834005749,16.1758310714255));
#45380=CARTESIAN_POINT('Ctrl Pts',(42.043877787894,2.79468963876171,15.605761363443));
#45381=CARTESIAN_POINT('Ctrl Pts',(41.9975739577311,2.01396872327272,15.1975471523719));
#45382=CARTESIAN_POINT('Ctrl Pts',(41.9512701275682,1.18317086006926,15.0009159663903));
#45383=CARTESIAN_POINT('Ctrl Pts',(41.9049662974053,0.352372996865793,14.8042847804088));
#45384=CARTESIAN_POINT('Ctrl Pts',(41.8586624672425,-0.528501814052137,
14.8192366195168));
#45385=CARTESIAN_POINT('Ctrl Pts',(41.8123586370796,-1.35214783517359,15.0439500919539));
#45386=CARTESIAN_POINT('Ctrl Pts',(41.7660548069167,-2.17579385629504,15.268663564391));
#45387=CARTESIAN_POINT('Ctrl Pts',(41.7197509767538,-2.94221108762,15.7031386701572));
#45388=CARTESIAN_POINT('Ctrl Pts',(41.6734471465909,-3.55803669798442,16.2944488513847));
#45389=CARTESIAN_POINT('Ctrl Pts',(41.627143316428,-4.17386230834885,16.8857590326121));
#45390=CARTESIAN_POINT('Ctrl Pts',(41.5808394862652,-4.63909629775273,17.6339042893008));
#45391=CARTESIAN_POINT('Ctrl Pts',(41.5345356561023,-4.89706514604382,18.4477476317908));
#45392=CARTESIAN_POINT('Ctrl Pts',(41.5060376058359,-5.05583406818061,18.9486338090611));
#45393=CARTESIAN_POINT('Ctrl Pts',(41.4775395555695,-5.13609339662976,19.4744056472516));
#45394=CARTESIAN_POINT('Ctrl Pts',(41.4490415053031,-5.13640319548555,20.0000850263462));
#45395=CARTESIAN_POINT('Ctrl Pts',(41.9259584946969,-5.13702782547439,19.9999018799691));
#45396=CARTESIAN_POINT('Ctrl Pts',(41.9316835136843,-5.13711983568307,19.8943342418265));
#45397=CARTESIAN_POINT('Ctrl Pts',(41.9374085326717,-5.13393220627652,19.788772154644));
#45398=CARTESIAN_POINT('Ctrl Pts',(41.9431335516591,-5.12742708469005,19.6834149009136));
#45399=CARTESIAN_POINT('Ctrl Pts',(41.989437381822,-5.07481380152163,18.8312877038006));
#45400=CARTESIAN_POINT('Ctrl Pts',(42.0357412119849,-4.80518545595153,17.9925597679348));
#45401=CARTESIAN_POINT('Ctrl Pts',(42.0820450421477,-4.35138742863618,17.2694026148691));
#45402=CARTESIAN_POINT('Ctrl Pts',(42.1283488723106,-3.89758940132085,16.5462454618034));
#45403=CARTESIAN_POINT('Ctrl Pts',(42.1746527024735,-3.25962169226028,15.9386590915378));
#45404=CARTESIAN_POINT('Ctrl Pts',(42.2209565326364,-2.51519976644497,15.5206579982489));
#45405=CARTESIAN_POINT('Ctrl Pts',(42.2672603627992,-1.77077784062965,15.1026569049599));
#45406=CARTESIAN_POINT('Ctrl Pts',(42.3135641929621,-0.919901698059582,
14.8742410886476));
#45407=CARTESIAN_POINT('Ctrl Pts',(42.359868023125,-0.0662227212891285,
14.8632355334353));
#45408=CARTESIAN_POINT('Ctrl Pts',(42.4061718532879,0.787456255481325,14.8522299782231));
#45409=CARTESIAN_POINT('Ctrl Pts',(42.4524756834507,1.64393806645217,15.0586346841109));
#45410=CARTESIAN_POINT('Ctrl Pts',(42.4987795136136,2.39888846202082,15.4573059996782));
#45411=CARTESIAN_POINT('Ctrl Pts',(42.5450833437765,3.15383885758947,15.8559773152454));
#45412=CARTESIAN_POINT('Ctrl Pts',(42.5913871739394,3.80725783775592,16.446915240492));
#45413=CARTESIAN_POINT('Ctrl Pts',(42.6376910041023,4.27954770634207,17.1581333488499));
#45414=CARTESIAN_POINT('Ctrl Pts',(42.6839948342652,4.75183757492822,17.8693514572079));
#45415=CARTESIAN_POINT('Ctrl Pts',(42.730298664428,5.04299833193406,18.7008497486771));
#45416=CARTESIAN_POINT('Ctrl Pts',(42.7766024945909,5.11756157778963,19.5513373970253));
#45417=CARTESIAN_POINT('Ctrl Pts',(42.8229063247538,5.19212482364519,20.4018250453735));
#45418=CARTESIAN_POINT('Ctrl Pts',(42.8692101549167,5.05009055835048,21.2713020506007));
#45419=CARTESIAN_POINT('Ctrl Pts',(42.9155139850795,4.70876100396969,22.0538511244175));
#45420=CARTESIAN_POINT('Ctrl Pts',(42.9618178152424,4.36743144958891,22.8364001982343));
#45421=CARTESIAN_POINT('Ctrl Pts',(43.0081216454053,3.82680660612205,23.5320213406409));
#45422=CARTESIAN_POINT('Ctrl Pts',(43.0544254755682,3.15274389942116,24.0559759045684));
#45423=CARTESIAN_POINT('Ctrl Pts',(43.1007293057311,2.47868119272028,24.5799304684959));
#45424=CARTESIAN_POINT('Ctrl Pts',(43.1470331358939,1.67118062278537,24.9322184539443));
#45425=CARTESIAN_POINT('Ctrl Pts',(43.1933369660568,0.828609679665406,25.0699251111374));
#45426=CARTESIAN_POINT('Ctrl Pts',(43.2396407962197,-0.0139612634545576,
25.2076317683305));
#45427=CARTESIAN_POINT('Ctrl Pts',(43.2859446263826,-0.89160257975957,25.1307570972682));
#45428=CARTESIAN_POINT('Ctrl Pts',(43.3322484565454,-1.69740242712528,24.8486657581407));
#45429=CARTESIAN_POINT('Ctrl Pts',(43.3785522867083,-2.50320227449099,24.5665744190131));
#45430=CARTESIAN_POINT('Ctrl Pts',(43.4248561168712,-3.2371606529174,24.0792664118203));
#45431=CARTESIAN_POINT('Ctrl Pts',(43.4711599470341,-3.80986877908679,23.4461042526186));
#45432=CARTESIAN_POINT('Ctrl Pts',(43.517463777197,-4.38257690525619,22.812942093417));
#45433=CARTESIAN_POINT('Ctrl Pts',(43.5637676073598,-4.79403477916857,22.0339257822065));
#45434=CARTESIAN_POINT('Ctrl Pts',(43.6100714375227,-4.99411973859361,21.2039529352788));
#45435=CARTESIAN_POINT('Ctrl Pts',(43.6320337899141,-5.08902196097241,20.810288824224));
#45436=CARTESIAN_POINT('Ctrl Pts',(43.6539961423055,-5.13637169871656,20.4051610405998));
#45437=CARTESIAN_POINT('Ctrl Pts',(43.6759584946968,-5.13631567875976,20.0000203800902));
#45438=CARTESIAN_POINT('Origin',(25.,0.,20.));
#45439=CARTESIAN_POINT('',(45.4259584946969,-5.13712894348962,20.0000625125626));
#45440=CARTESIAN_POINT('',(44.9490415053031,-5.13635638952797,19.9999383013781));
#45441=CARTESIAN_POINT('',(25.,-5.13675,20.));
#45442=CARTESIAN_POINT('Ctrl Pts',(44.9490415053031,-5.13635638952797,19.9999383013781));
#45443=CARTESIAN_POINT('Ctrl Pts',(44.9221648128119,-5.13614682048153,20.4957228006643));
#45444=CARTESIAN_POINT('Ctrl Pts',(44.8952881203207,-5.06488923577723,20.9915662676101));
#45445=CARTESIAN_POINT('Ctrl Pts',(44.8684114278296,-4.92342543575894,21.4664980183179));
#45446=CARTESIAN_POINT('Ctrl Pts',(44.8221075976667,-4.67970810437996,22.2847221778178));
#45447=CARTESIAN_POINT('Ctrl Pts',(44.7758037675038,-4.22760994953467,23.040877749369));
#45448=CARTESIAN_POINT('Ctrl Pts',(44.7294999373409,-3.62220432027531,23.6428519488702));
#45449=CARTESIAN_POINT('Ctrl Pts',(44.6831961071781,-3.01679869101595,24.2448261483713));
#45450=CARTESIAN_POINT('Ctrl Pts',(44.6368922770152,-2.25808558734251,24.6926189758224));
#45451=CARTESIAN_POINT('Ctrl Pts',(44.5905884468523,-1.43848934485844,24.931681545268));
#45452=CARTESIAN_POINT('Ctrl Pts',(44.5442846166895,-0.618893102374381,
25.1707441147136));
#45453=CARTESIAN_POINT('Ctrl Pts',(44.4979807865265,0.261586278920312,25.2010764261538));
#45454=CARTESIAN_POINT('Ctrl Pts',(44.4516769563636,1.09569123165968,25.0189834811516));
#45455=CARTESIAN_POINT('Ctrl Pts',(44.4053731262007,1.92979618439905,24.8368905361493));
#45456=CARTESIAN_POINT('Ctrl Pts',(44.3590692960379,2.7175267085831,24.4423723347047));
#45457=CARTESIAN_POINT('Ctrl Pts',(44.312765465875,3.36292364655426,23.8834879949157));
#45458=CARTESIAN_POINT('Ctrl Pts',(44.2664616357121,4.00832058452544,23.3246036551267));
#45459=CARTESIAN_POINT('Ctrl Pts',(44.2201578055493,4.51138393628372,22.6013531769933));
#45460=CARTESIAN_POINT('Ctrl Pts',(44.1738539753864,4.81083191319573,21.8018409369824));
#45461=CARTESIAN_POINT('Ctrl Pts',(44.1275501452235,5.11027989010774,21.0023286969715));
#45462=CARTESIAN_POINT('Ctrl Pts',(44.0812463150606,5.20611249217347,20.1265546950831));
#45463=CARTESIAN_POINT('Ctrl Pts',(44.0349424848978,5.08665565638783,19.2812033023546));
#45464=CARTESIAN_POINT('Ctrl Pts',(43.9886386547349,4.96719882060219,18.4358519096261));
#45465=CARTESIAN_POINT('Ctrl Pts',(43.942334824572,4.63245254696518,17.6209231260575));
#45466=CARTESIAN_POINT('Ctrl Pts',(43.8960309944091,4.12319470235011,16.9356893261746));
#45467=CARTESIAN_POINT('Ctrl Pts',(43.8497271642462,3.61393685773505,16.2504555262917));
#45468=CARTESIAN_POINT('Ctrl Pts',(43.8034233340834,2.93016744214192,15.6949167100945));
#45469=CARTESIAN_POINT('Ctrl Pts',(43.7571195039205,2.15518135799981,15.3367470824179));
#45470=CARTESIAN_POINT('Ctrl Pts',(43.7108156737576,1.3801952738577,14.9785774547412));
#45471=CARTESIAN_POINT('Ctrl Pts',(43.6645118435947,0.513992521166593,14.8177770155852));
#45472=CARTESIAN_POINT('Ctrl Pts',(43.6182080134318,-0.337908472188524,
14.8739340305034));
#45473=CARTESIAN_POINT('Ctrl Pts',(43.571904183269,-1.18980946554365,14.9300910454215));
#45474=CARTESIAN_POINT('Ctrl Pts',(43.5256003531061,-2.02740869956279,15.2032055144139));
#45475=CARTESIAN_POINT('Ctrl Pts',(43.4792965229432,-2.74867214803584,15.6600073868934));
#45476=CARTESIAN_POINT('Ctrl Pts',(43.4329926927803,-3.46993559650886,16.1168092593728));
#45477=CARTESIAN_POINT('Ctrl Pts',(43.3866888626174,-4.07486325943579,16.7572985353393));
#45478=CARTESIAN_POINT('Ctrl Pts',(43.3403850324546,-4.48976451902782,17.5034525794836));
#45479=CARTESIAN_POINT('Ctrl Pts',(43.2940812022917,-4.90466577861986,18.2496066236279));
#45480=CARTESIAN_POINT('Ctrl Pts',(43.2477773721288,-5.129540634877,19.1014254359499));
#45481=CARTESIAN_POINT('Ctrl Pts',(43.2014735419659,-5.13699545365367,19.9551428004687));
#45482=CARTESIAN_POINT('Ctrl Pts',(43.2006628630783,-5.13712597124092,19.9700895260629));
#45483=CARTESIAN_POINT('Ctrl Pts',(43.1998521841907,-5.13718984445936,19.985036833608));
#45484=CARTESIAN_POINT('Ctrl Pts',(43.1990415053031,-5.13718721057151,19.9999841637545));
#45485=CARTESIAN_POINT('Ctrl Pts',(43.6759584946968,-5.13631567875976,20.0000203800902));
#45486=CARTESIAN_POINT('Ctrl Pts',(43.7002999724684,-5.13625359030453,19.5509918695563));
#45487=CARTESIAN_POINT('Ctrl Pts',(43.7246414502399,-5.07795875684034,19.1019475411889));
#45488=CARTESIAN_POINT('Ctrl Pts',(43.7489829280114,-4.96163094092812,18.6684771726323));
#45489=CARTESIAN_POINT('Ctrl Pts',(43.7952867581742,-4.74034513889991,17.8439036395583));
#45490=CARTESIAN_POINT('Ctrl Pts',(43.8415905883371,-4.30906148990579,17.0756859560552));
#45491=CARTESIAN_POINT('Ctrl Pts',(43.8878944185,-3.72031777736076,16.4574062794006));
#45492=CARTESIAN_POINT('Ctrl Pts',(43.9341982486629,-3.13157406481572,15.8391266027461));
#45493=CARTESIAN_POINT('Ctrl Pts',(43.9805020788258,-2.38537028871977,15.37078493294));
#45494=CARTESIAN_POINT('Ctrl Pts',(44.0268059089886,-1.57260693292711,15.1094333591816));
#45495=CARTESIAN_POINT('Ctrl Pts',(44.0731097391515,-0.759843577134466,
14.8480817854231));
#45496=CARTESIAN_POINT('Ctrl Pts',(44.1194135693144,0.119479358354885,14.7937203077121));
#45497=CARTESIAN_POINT('Ctrl Pts',(44.1657173994773,0.95824518121023,14.9529710911801));
#45498=CARTESIAN_POINT('Ctrl Pts',(44.2120212296401,1.79701100406557,15.112221874648));
#45499=CARTESIAN_POINT('Ctrl Pts',(44.258325059803,2.59521971428691,15.4850849192949));
#45500=CARTESIAN_POINT('Ctrl Pts',(44.3046288899659,3.25563573052222,16.0261390784372));
#45501=CARTESIAN_POINT('Ctrl Pts',(44.3509327201288,3.91605174675754,16.5671932375796));
#45502=CARTESIAN_POINT('Ctrl Pts',(44.3972365502917,4.43867506900683,17.2764385112175));
#45503=CARTESIAN_POINT('Ctrl Pts',(44.4435403804546,4.75984116703344,18.0674765982296));
#45504=CARTESIAN_POINT('Ctrl Pts',(44.4898442106174,5.08100726506006,18.8585146852417));
#45505=CARTESIAN_POINT('Ctrl Pts',(44.5361480407803,5.200716138864,19.7313455856279));
#45506=CARTESIAN_POINT('Ctrl Pts',(44.5824518709432,5.10438518393562,20.5796434488505));
#45507=CARTESIAN_POINT('Ctrl Pts',(44.6287557011061,5.00805422900723,21.427941312073));
#45508=CARTESIAN_POINT('Ctrl Pts',(44.6750595312689,4.69568344534651,22.2517061381319));
#45509=CARTESIAN_POINT('Ctrl Pts',(44.7213633614318,4.20532497941302,22.9505891702));
#45510=CARTESIAN_POINT('Ctrl Pts',(44.7676671915947,3.71496651347954,23.6494722022681));
#45511=CARTESIAN_POINT('Ctrl Pts',(44.8139710217576,3.04662036527329,24.2234734403455));
#45512=CARTESIAN_POINT('Ctrl Pts',(44.8602748519205,2.28170261737147,24.6026696383357));
#45513=CARTESIAN_POINT('Ctrl Pts',(44.9065786820833,1.51678486946965,24.9818658363258));
#45514=CARTESIAN_POINT('Ctrl Pts',(44.9528825122462,0.655295521872253,25.1662569942286));
#45515=CARTESIAN_POINT('Ctrl Pts',(44.9991863424091,-0.197821171531303,
25.1333810902631));
#45516=CARTESIAN_POINT('Ctrl Pts',(45.0454901725719,-1.05093786493486,25.1005051862975));
#45517=CARTESIAN_POINT('Ctrl Pts',(45.0917940027349,-1.89568190414457,24.8503622204636));
#45518=CARTESIAN_POINT('Ctrl Pts',(45.1380978328977,-2.6291489025077,24.4134239182543));
#45519=CARTESIAN_POINT('Ctrl Pts',(45.1844016630606,-3.36261590087082,23.976485616045));
#45520=CARTESIAN_POINT('Ctrl Pts',(45.2307054932235,-3.98480585838736,23.3527519774603));
#45521=CARTESIAN_POINT('Ctrl Pts',(45.2770093233863,-4.41992531220002,22.6182045123233));
#45522=CARTESIAN_POINT('Ctrl Pts',(45.3233131535492,-4.85504476601268,21.8836570471864));
#45523=CARTESIAN_POINT('Ctrl Pts',(45.3696169837121,-5.10309371612148,21.0382957554972));
#45524=CARTESIAN_POINT('Ctrl Pts',(45.415920813875,-5.13385552424782,20.1851002159014));
#45525=CARTESIAN_POINT('Ctrl Pts',(45.4192667074823,-5.13607835844526,20.1234486961101));
#45526=CARTESIAN_POINT('Ctrl Pts',(45.4226126010896,-5.1371666405299,20.0617562702512));
#45527=CARTESIAN_POINT('Ctrl Pts',(45.4259584946969,-5.13712894348962,20.0000625125626));
#45528=CARTESIAN_POINT('Origin',(25.,0.,20.));
#45529=CARTESIAN_POINT('',(47.1759584946969,-5.13650480025366,19.9998861825852));
#45530=CARTESIAN_POINT('',(46.6990415053031,-5.13689122437247,20.0001232958892));
#45531=CARTESIAN_POINT('',(25.,-5.13675,20.));
#45532=CARTESIAN_POINT('Ctrl Pts',(46.6990415053031,-5.13689122437247,20.0001232958892));
#45533=CARTESIAN_POINT('Ctrl Pts',(46.690781271596,-5.13704510784903,20.152451236073));
#45534=CARTESIAN_POINT('Ctrl Pts',(46.6825210378889,-5.13040429337675,20.3047658062091));
#45535=CARTESIAN_POINT('Ctrl Pts',(46.6742608041819,-5.11687147158231,20.4564655545811));
#45536=CARTESIAN_POINT('Ctrl Pts',(46.627956974019,-5.04101145306286,21.3068385141673));
#45537=CARTESIAN_POINT('Ctrl Pts',(46.5816531438561,-4.74858313169487,22.1378918619507));
#45538=CARTESIAN_POINT('Ctrl Pts',(46.5353493136932,-4.27520931824056,22.8483889735136));
#45539=CARTESIAN_POINT('Ctrl Pts',(46.4890454835303,-3.80183550478624,23.5588860850765));
#45540=CARTESIAN_POINT('Ctrl Pts',(46.4427416533675,-3.14751619924559,24.1488269604189));
#45541=CARTESIAN_POINT('Ctrl Pts',(46.3964378232046,-2.39195877294756,24.5463466308377));
#45542=CARTESIAN_POINT('Ctrl Pts',(46.3501339930417,-1.63640134664952,24.9438663012566));
#45543=CARTESIAN_POINT('Ctrl Pts',(46.3038301628788,-0.779605799594105,
25.1489647667518));
#45544=CARTESIAN_POINT('Ctrl Pts',(46.2575263327159,0.0740554001521648,
25.1366574985019));
#45545=CARTESIAN_POINT('Ctrl Pts',(46.211222502553,0.927716599898423,25.1243502302519));
#45546=CARTESIAN_POINT('Ctrl Pts',(46.1649186723902,1.77824345233553,24.8946372282569));
#45547=CARTESIAN_POINT('Ctrl Pts',(46.1186148422273,2.52202712446896,24.4755014962182));
#45548=CARTESIAN_POINT('Ctrl Pts',(46.0723110120645,3.2658107966024,24.0563657641796));
#45549=CARTESIAN_POINT('Ctrl Pts',(46.0260071819015,3.90285128843215,23.4478073020973));
#45550=CARTESIAN_POINT('Ctrl Pts',(45.9797033517386,4.35554608601079,22.7239590216896));
#45551=CARTESIAN_POINT('Ctrl Pts',(45.9333995215757,4.80824088358944,22.0001107412819));
#45552=CARTESIAN_POINT('Ctrl Pts',(45.8870956914129,5.07658998691698,21.1609726425487));
#45553=CARTESIAN_POINT('Ctrl Pts',(45.8407918612501,5.12790384909524,20.3087662119509));
#45554=CARTESIAN_POINT('Ctrl Pts',(45.7944880310872,5.17921771127349,19.4565597813531));
#45555=CARTESIAN_POINT('Ctrl Pts',(45.7481842009243,5.01349633230246,18.5912850188906));
#45556=CARTESIAN_POINT('Ctrl Pts',(45.7018803707614,4.65092743303804,17.818347307241));
#45557=CARTESIAN_POINT('Ctrl Pts',(45.6555765405985,4.28835853377361,17.0454095955914));
#45558=CARTESIAN_POINT('Ctrl Pts',(45.6092727104357,3.7289421142158,16.3648089347546));
#45559=CARTESIAN_POINT('Ctrl Pts',(45.5629688802728,3.04082473813548,15.8594542182037));
#45560=CARTESIAN_POINT('Ctrl Pts',(45.5166650501099,2.35270736205516,15.3540995016527));
#45561=CARTESIAN_POINT('Ctrl Pts',(45.470361219947,1.53588902945233,15.0239907293876));
#45562=CARTESIAN_POINT('Ctrl Pts',(45.4240573897841,0.689872294499334,14.909340840668));
#45563=CARTESIAN_POINT('Ctrl Pts',(45.3777535596212,-0.156144440453653,
14.7946909519484));
#45564=CARTESIAN_POINT('Ctrl Pts',(45.3314497294584,-1.03135957775681,14.8954999467743));
#45565=CARTESIAN_POINT('Ctrl Pts',(45.2851458992955,-1.8291568257135,15.1994875517135));
#45566=CARTESIAN_POINT('Ctrl Pts',(45.2388420691326,-2.62695407367019,15.5034751566527));
#45567=CARTESIAN_POINT('Ctrl Pts',(45.1925382389697,-3.3473334322804,16.0106413717052));
#45568=CARTESIAN_POINT('Ctrl Pts',(45.1462344088068,-3.90254027693094,16.6592046087586));
#45569=CARTESIAN_POINT('Ctrl Pts',(45.099930578644,-4.45774712158149,17.3077678458119));
#45570=CARTESIAN_POINT('Ctrl Pts',(45.0536267484811,-4.84778145227236,18.0977281048661));
#45571=CARTESIAN_POINT('Ctrl Pts',(45.0073229183182,-5.02513036366146,18.9328546081176));
#45572=CARTESIAN_POINT('Ctrl Pts',(44.9878957806465,-5.09953850021006,19.2832385287324));
#45573=CARTESIAN_POINT('Ctrl Pts',(44.9684686429748,-5.13650787121488,19.6415730104744));
#45574=CARTESIAN_POINT('Ctrl Pts',(44.9490415053031,-5.13635638952797,19.9999383013781));
#45575=CARTESIAN_POINT('Ctrl Pts',(45.4259584946969,-5.13712894348962,20.0000625125626));
#45576=CARTESIAN_POINT('Ctrl Pts',(45.4689164312525,-5.13664495109337,19.207976200288));
#45577=CARTESIAN_POINT('Ctrl Pts',(45.511874367808,-4.95055457497461,18.415670349234));
#45578=CARTESIAN_POINT('Ctrl Pts',(45.5548323043636,-4.59700152388307,17.7068991249416));
#45579=CARTESIAN_POINT('Ctrl Pts',(45.6011361345265,-4.21591104924808,16.9429233610801));
#45580=CARTESIAN_POINT('Ctrl Pts',(45.6474399646894,-3.64025543383418,16.2760016208595));
#45581=CARTESIAN_POINT('Ctrl Pts',(45.6937437948523,-2.94015945541774,15.7873764694085));
#45582=CARTESIAN_POINT('Ctrl Pts',(45.7400476250152,-2.2400634770013,15.2987513179574));
#45583=CARTESIAN_POINT('Ctrl Pts',(45.786351455178,-1.4155271355823,14.9884227552759));
#45584=CARTESIAN_POINT('Ctrl Pts',(45.8326552853409,-0.566993171858652,
14.8941941501028));
#45585=CARTESIAN_POINT('Ctrl Pts',(45.8789591155038,0.281540791864998,14.7999655449297));
#45586=CARTESIAN_POINT('Ctrl Pts',(45.9252629456667,1.1540723778933,14.9218368972651));
#45587=CARTESIAN_POINT('Ctrl Pts',(45.9715667758296,1.9443121973366,15.2449621754332));
#45588=CARTESIAN_POINT('Ctrl Pts',(46.0178706059924,2.73455201677989,15.5680874536012));
#45589=CARTESIAN_POINT('Ctrl Pts',(46.0641744361553,3.44250006963818,16.0924666576019));
#45590=CARTESIAN_POINT('Ctrl Pts',(46.1104782663182,3.981916078645,16.7542213605348));
#45591=CARTESIAN_POINT('Ctrl Pts',(46.1567820964811,4.52133208765183,17.4159760634677));
#45592=CARTESIAN_POINT('Ctrl Pts',(46.2030859266439,4.89221605280719,18.2151062653327));
#45593=CARTESIAN_POINT('Ctrl Pts',(46.2493897568068,5.04938791342566,19.0542641312032));
#45594=CARTESIAN_POINT('Ctrl Pts',(46.2956935869697,5.20655977404413,19.8934219970738));
#45595=CARTESIAN_POINT('Ctrl Pts',(46.3419974171325,5.15001953012569,20.7726075269498));
#45596=CARTESIAN_POINT('Ctrl Pts',(46.3883012472954,4.8866547580894,21.5847207668863));
#45597=CARTESIAN_POINT('Ctrl Pts',(46.4346050774583,4.62328998605311,22.3968340068228));
#45598=CARTESIAN_POINT('Ctrl Pts',(46.4809089076212,4.15310068589896,23.1418749568197));
#45599=CARTESIAN_POINT('Ctrl Pts',(46.5272127377841,3.53336402004704,23.7290847852619));
#45600=CARTESIAN_POINT('Ctrl Pts',(46.573516567947,2.91362735419512,24.316294613704));
#45601=CARTESIAN_POINT('Ctrl Pts',(46.6198203981098,2.14434332264542,24.7456733205914));
#45602=CARTESIAN_POINT('Ctrl Pts',(46.6661242282727,1.31922398226423,24.9649151773485));
#45603=CARTESIAN_POINT('Ctrl Pts',(46.7124280584356,0.494104641883048,25.1841570341056));
#45604=CARTESIAN_POINT('Ctrl Pts',(46.7587318885985,-0.386850007329603,
25.1932620407324));
#45605=CARTESIAN_POINT('Ctrl Pts',(46.8050357187614,-1.21632450220898,24.9911210503581));
#45606=CARTESIAN_POINT('Ctrl Pts',(46.8513395489243,-2.04579899708836,24.7889800599838));
#45607=CARTESIAN_POINT('Ctrl Pts',(46.8976433790871,-2.82379333763447,24.3755930726083));
#45608=CARTESIAN_POINT('Ctrl Pts',(46.94394720925,-3.45553440114763,23.8013177499372));
#45609=CARTESIAN_POINT('Ctrl Pts',(46.9902510394129,-4.0872754646608,23.2270424272662));
#45610=CARTESIAN_POINT('Ctrl Pts',(47.0365548695757,-4.57276325114104,22.4918787692994));
#45611=CARTESIAN_POINT('Ctrl Pts',(47.0828586997386,-4.85285697889777,21.6853823827887));
#45612=CARTESIAN_POINT('Ctrl Pts',(47.1138919647247,-5.04057844478594,21.1448608754995));
#45613=CARTESIAN_POINT('Ctrl Pts',(47.1449252297108,-5.13604085957544,20.572298081872));
#45614=CARTESIAN_POINT('Ctrl Pts',(47.1759584946969,-5.13650480025366,19.9998861825852));
#45615=CARTESIAN_POINT('Origin',(25.,0.,20.));
#45616=CARTESIAN_POINT('',(48.9259584946969,-5.13665113575917,20.0001315872378));
#45617=CARTESIAN_POINT('',(48.4490415053031,-5.1367692385953,19.9998673509107));
#45618=CARTESIAN_POINT('',(25.,-5.13675,20.));
#45619=CARTESIAN_POINT('',(50.,3.87994761181438,23.3663343702128));
#45620=CARTESIAN_POINT('Ctrl Pts',(48.9259584946969,-5.13665113575917,20.0001315872378));
#45621=CARTESIAN_POINT('Ctrl Pts',(48.9598455186578,-5.13603933143329,19.3751337947736));
#45622=CARTESIAN_POINT('Ctrl Pts',(48.9937325426186,-5.02179317828337,18.7499187416812));
#45623=CARTESIAN_POINT('Ctrl Pts',(49.0276195665795,-4.79876653798914,18.1662697419488));
#45624=CARTESIAN_POINT('Ctrl Pts',(49.0739233967424,-4.49401898370703,17.3687614039629));
#45625=CARTESIAN_POINT('Ctrl Pts',(49.1202272269053,-3.98616766501212,16.6488609360172));
#45626=CARTESIAN_POINT('Ctrl Pts',(49.1665310570682,-3.33707491734228,16.0942748452934));
#45627=CARTESIAN_POINT('Ctrl Pts',(49.212834887231,-2.68798216967244,15.5396887545696));
#45628=CARTESIAN_POINT('Ctrl Pts',(49.2591387173939,-1.89764799302765,15.1504170410676));
#45629=CARTESIAN_POINT('Ctrl Pts',(49.3054425475568,-1.0623540544481,14.9738595777119));
#45630=CARTESIAN_POINT('Ctrl Pts',(49.3517463777197,-0.22706011586855,14.7973021143561));
#45631=CARTESIAN_POINT('Ctrl Pts',(49.3980502078826,0.653193584645775,14.8334589011466));
#45632=CARTESIAN_POINT('Ctrl Pts',(49.4443540380455,1.47118750635313,15.0779651040003));
#45633=CARTESIAN_POINT('Ctrl Pts',(49.4906578682084,2.28918142806049,15.3224713068541));
#45634=CARTESIAN_POINT('Ctrl Pts',(49.5369616983712,3.04491557096088,15.7753269257712));
#45635=CARTESIAN_POINT('Ctrl Pts',(49.5832655285341,3.64630753914303,16.3812878173559));
#45636=CARTESIAN_POINT('Ctrl Pts',(49.6295693586969,4.24769950732517,16.9872487089406));
#45637=CARTESIAN_POINT('Ctrl Pts',(49.6758731888598,4.69474930078906,17.7463148731928));
#45638=CARTESIAN_POINT('Ctrl Pts',(49.7221770190227,4.93304205845025,18.5661776434962));
#45639=CARTESIAN_POINT('Ctrl Pts',(49.7684808491856,5.17133481611145,19.3860404137995));
#45640=CARTESIAN_POINT('Ctrl Pts',(49.8147846793485,5.20087053796993,20.2666997901539));
#45641=CARTESIAN_POINT('Ctrl Pts',(49.8610885095113,5.0179360691547,21.1005140400636));
#45642=CARTESIAN_POINT('Ctrl Pts',(49.9073923396742,4.83500160033947,21.9343282899734));
#45643=CARTESIAN_POINT('Ctrl Pts',(49.9536961698371,4.43959694085051,22.7212974134384));
#45644=CARTESIAN_POINT('Ctrl Pts',(50.,3.87994761181434,23.3663343702128));
#45645=CARTESIAN_POINT('',(50.,-3.88028650238532,23.366567607224));
#45646=CARTESIAN_POINT('Origin',(50.,0.,20.));
#45647=CARTESIAN_POINT('Ctrl Pts',(50.,-3.88028650238532,23.366567607224));
#45648=CARTESIAN_POINT('Ctrl Pts',(49.9564083618068,-3.35323397491262,23.9734064748655));
#45649=CARTESIAN_POINT('Ctrl Pts',(49.9128167236137,-2.68147453498408,24.4549327642161));
#45650=CARTESIAN_POINT('Ctrl Pts',(49.8692250854205,-1.93705761091916,24.7579923400498));
#45651=CARTESIAN_POINT('Ctrl Pts',(49.8229212552576,-1.14632442788237,25.0799077281905));
#45652=CARTESIAN_POINT('Ctrl Pts',(49.7766174250947,-0.273611264823877,
25.2004577954347));
#45653=CARTESIAN_POINT('Ctrl Pts',(49.7303135949318,0.574777228598876,25.1049377152569));
#45654=CARTESIAN_POINT('Ctrl Pts',(49.6840097647689,1.42316572202163,25.0094176350791));
#45655=CARTESIAN_POINT('Ctrl Pts',(49.6377059346061,2.24722954580865,24.6978274074791));
#45656=CARTESIAN_POINT('Ctrl Pts',(49.5914021044432,2.94658003659829,24.2081341237764));
#45657=CARTESIAN_POINT('Ctrl Pts',(49.5450982742803,3.64593052738793,23.7184408400736));
#45658=CARTESIAN_POINT('Ctrl Pts',(49.4987944441175,4.22056768518019,23.0506445002681));
#45659=CARTESIAN_POINT('Ctrl Pts',(49.4524906139546,4.60049256722468,22.2860891164051));
#45660=CARTESIAN_POINT('Ctrl Pts',(49.4061867837917,4.98041744926916,21.5215337325421));
#45661=CARTESIAN_POINT('Ctrl Pts',(49.3598829536288,5.16563005556587,20.6602193046217));
#45662=CARTESIAN_POINT('Ctrl Pts',(49.3135791234659,5.13356739906873,19.8070713658671));
#45663=CARTESIAN_POINT('Ctrl Pts',(49.2672752933031,5.10150474257159,18.9539234271126));
#45664=CARTESIAN_POINT('Ctrl Pts',(49.2209714631402,4.85216682328062,18.108941977524));
#45665=CARTESIAN_POINT('Ctrl Pts',(49.1746676329773,4.41592775461009,17.3750590101374));
#45666=CARTESIAN_POINT('Ctrl Pts',(49.1283638028144,3.97968868593957,16.6411760427509));
#45667=CARTESIAN_POINT('Ctrl Pts',(49.0820599726515,3.3565484678895,16.0183915575663));
#45668=CARTESIAN_POINT('Ctrl Pts',(49.0357561424887,2.62241608957914,15.5825721087253));
#45669=CARTESIAN_POINT('Ctrl Pts',(48.9894523123258,1.88828371126878,15.1467526598842));
#45670=CARTESIAN_POINT('Ctrl Pts',(48.9431484821629,1.04315917269814,14.8978982473866));
#45671=CARTESIAN_POINT('Ctrl Pts',(48.8968446520001,0.189993329665845,14.8663232896413));
#45672=CARTESIAN_POINT('Ctrl Pts',(48.8505408218372,-0.663172513366446,
14.834748331896));
#45673=CARTESIAN_POINT('Ctrl Pts',(48.8042369916742,-1.52437966086038,15.0204528289029));
#45674=CARTESIAN_POINT('Ctrl Pts',(48.7579331615114,-2.28871829557969,15.4008149437621));
#45675=CARTESIAN_POINT('Ctrl Pts',(48.7116293313485,-3.053056930299,15.7811770586214));
#45676=CARTESIAN_POINT('Ctrl Pts',(48.6653255011856,-3.72052705224367,16.3561967913331));
#45677=CARTESIAN_POINT('Ctrl Pts',(48.6190216710228,-4.20981926355514,17.0558267381184));
#45678=CARTESIAN_POINT('Ctrl Pts',(48.5727178408599,-4.69911147486661,17.7554566849037));
#45679=CARTESIAN_POINT('Ctrl Pts',(48.526414010697,-5.01022577554488,18.5796968457626));
#45680=CARTESIAN_POINT('Ctrl Pts',(48.4801101805341,-5.1052630958502,19.4281406043275));
#45681=CARTESIAN_POINT('Ctrl Pts',(48.4697539554571,-5.12651895905494,19.6179018940085));
#45682=CARTESIAN_POINT('Ctrl Pts',(48.4593977303801,-5.13696601854414,19.8088739185692));
#45683=CARTESIAN_POINT('Ctrl Pts',(48.4490415053031,-5.1367692385953,19.9998673509107));
#45684=CARTESIAN_POINT('Origin',(53.8647410325606,0.,20.));
#45685=CARTESIAN_POINT('',(0.635258967439483,-6.11286903553622,19.9998876627387));
#45686=CARTESIAN_POINT('',(0.489741032560566,-6.11272135172475,19.9999876119473));
#45687=CARTESIAN_POINT('',(53.8647410325606,-6.11325,19.9999999999994));
#45688=CARTESIAN_POINT('',(0.,1.1399249411295,26.0060300274883));
#45689=CARTESIAN_POINT('Ctrl Pts',(0.489741032560565,-6.11272135172475,
19.9999876119473));
#45690=CARTESIAN_POINT('Ctrl Pts',(0.465405512195678,-6.1126401423534,20.5342537111184));
#45691=CARTESIAN_POINT('Ctrl Pts',(0.394766161667913,-5.91134392484222,
22.0851281076538));
#45692=CARTESIAN_POINT('Ctrl Pts',(0.277822980977271,-4.61535544548857,
24.3940602366606));
#45693=CARTESIAN_POINT('Ctrl Pts',(0.138911490488638,-1.95089886648438,
26.0667560931559));
#45694=CARTESIAN_POINT('Ctrl Pts',(0.0463038301628798,0.141429157467205,
26.1955412757171));
#45695=CARTESIAN_POINT('Ctrl Pts',(0.,1.1399249411295,26.0060300274883));
#45696=CARTESIAN_POINT('',(3.4031358915606E-15,3.9853303828714,24.6362610213064));
#45697=CARTESIAN_POINT('Origin',(0.,0.,20.));
#45698=CARTESIAN_POINT('Ctrl Pts',(0.635258967439483,-6.11286903553622,
19.9998876627387));
#45699=CARTESIAN_POINT('Ctrl Pts',(0.606009106974798,-6.11244475391168,
20.6419943076294));
#45700=CARTESIAN_POINT('Ctrl Pts',(0.530455416347233,-5.85230460599341,
22.3009199263206));
#45701=CARTESIAN_POINT('Ctrl Pts',(0.408597895556788,-4.37627520273034,
24.6322128254603));
#45702=CARTESIAN_POINT('Ctrl Pts',(0.269686405068149,-1.62745906490466,
26.1612286823026));
#45703=CARTESIAN_POINT('Ctrl Pts',(0.133487106549218,1.45644183765853,26.1885630898315));
#45704=CARTESIAN_POINT('Ctrl Pts',(0.0435916381931709,3.25961188313384,
25.2594316761304));
#45705=CARTESIAN_POINT('Ctrl Pts',(2.63081657153608E-15,3.9853303828714,
24.6362610213064));
#45706=CARTESIAN_POINT('Origin',(53.8647410325606,0.,20.));
#45707=CARTESIAN_POINT('',(2.38525896743947,-6.11325364908754,20.0001583732729));
#45708=CARTESIAN_POINT('',(2.23974103256055,-6.11358099250321,20.0001166795099));
#45709=CARTESIAN_POINT('',(53.8647410325606,-6.11325,19.9999999999994));
#45710=CARTESIAN_POINT('Ctrl Pts',(2.23974103256055,-6.11358099250321,20.0001166795099));
#45711=CARTESIAN_POINT('Ctrl Pts',(2.23402197097976,-6.11369031868212,20.1256220477198));
#45712=CARTESIAN_POINT('Ctrl Pts',(2.18199907923609,-6.07925402918527,21.2672095839662));
#45713=CARTESIAN_POINT('Ctrl Pts',(2.08367235732954,-5.39798721704175,23.3868805022452));
#45714=CARTESIAN_POINT('Ctrl Pts',(1.94476086684091,-3.12038893862028,25.556293575601));
#45715=CARTESIAN_POINT('Ctrl Pts',(1.80584937635227,-0.0825561728535726,
26.3720021186908));
#45716=CARTESIAN_POINT('Ctrl Pts',(1.66693788586364,2.97538981548086,25.6352709416678));
#45717=CARTESIAN_POINT('Ctrl Pts',(1.528026395375,5.30842886408474,23.5255940754177));
#45718=CARTESIAN_POINT('Ctrl Pts',(1.38911490488636,6.34815042253135,20.5569597405651));
#45719=CARTESIAN_POINT('Ctrl Pts',(1.25020341439772,5.84124601468089,17.4526331642158));
#45720=CARTESIAN_POINT('Ctrl Pts',(1.11129192390908,3.91120805214414,14.9689283406313));
#45721=CARTESIAN_POINT('Ctrl Pts',(0.972380433420452,1.02827407433471,13.7109751703986));
#45722=CARTESIAN_POINT('Ctrl Pts',(0.833468942931815,-2.10520088120389,
13.985227291767));
#45723=CARTESIAN_POINT('Ctrl Pts',(0.694557452443171,-4.72574094137507,
15.7249208643558));
#45724=CARTESIAN_POINT('Ctrl Pts',(0.579981482319428,-5.93760230752943,
18.0188739705022));
#45725=CARTESIAN_POINT('Ctrl Pts',(0.511709342358557,-6.11279466154519,
19.5176916509335));
#45726=CARTESIAN_POINT('Ctrl Pts',(0.489741032560565,-6.11272135172475,
19.9999876119473));
#45727=CARTESIAN_POINT('Ctrl Pts',(2.38525896743947,-6.11325364908754,20.0001583732729));
#45728=CARTESIAN_POINT('Ctrl Pts',(2.37462556575888,-6.11349338758375,20.2335454665235));
#45729=CARTESIAN_POINT('Ctrl Pts',(2.31768833391541,-6.04330000224885,21.4830882729956));
#45730=CARTESIAN_POINT('Ctrl Pts',(2.21444727190907,-5.2112318370928,23.6677360978016));
#45731=CARTESIAN_POINT('Ctrl Pts',(2.07553578142043,-2.82204320093811,25.7136063473297));
#45732=CARTESIAN_POINT('Ctrl Pts',(1.93662429093179,0.254692459677778,26.3674451025059));
#45733=CARTESIAN_POINT('Ctrl Pts',(1.79771280044316,3.26937625297555,25.4699546773483));
#45734=CARTESIAN_POINT('Ctrl Pts',(1.65880130995452,5.48752727391192,23.2397947266211));
#45735=CARTESIAN_POINT('Ctrl Pts',(1.51988981946589,6.36872743946243,20.220309021366));
#45736=CARTESIAN_POINT('Ctrl Pts',(1.38097832897725,5.69828603890732,17.1471485537567));
#45737=CARTESIAN_POINT('Ctrl Pts',(1.24206683848861,3.63954565029315,14.7690408411714));
#45738=CARTESIAN_POINT('Ctrl Pts',(1.10315534799997,0.694086537873731,13.6653755651264));
#45739=CARTESIAN_POINT('Ctrl Pts',(0.964243857511333,-2.4204761475888,14.1050423605135));
#45740=CARTESIAN_POINT('Ctrl Pts',(0.8253323670227,-4.94532707163062,15.9809257548385));
#45741=CARTESIAN_POINT('Ctrl Pts',(0.715670736998751,-5.98738112992614,
18.2348148939576));
#45742=CARTESIAN_POINT('Ctrl Pts',(0.652312937137678,-6.11311641059558,
19.6255109275677));
#45743=CARTESIAN_POINT('Ctrl Pts',(0.635258967439483,-6.11286903553622,
19.9998876627387));
#45744=CARTESIAN_POINT('Origin',(53.8647410325606,0.,20.));
#45745=CARTESIAN_POINT('',(4.13525896743946,-6.11343686380434,19.9998556839975));
#45746=CARTESIAN_POINT('',(3.98974103256054,-6.1131009424828,19.999845624611));
#45747=CARTESIAN_POINT('',(53.8647410325606,-6.11325,19.9999999999994));
#45748=CARTESIAN_POINT('Ctrl Pts',(3.98974103256054,-6.11310094248279,19.999845624611));
#45749=CARTESIAN_POINT('Ctrl Pts',(3.95633459960097,-6.11239888135295,20.7331189949968));
#45750=CARTESIAN_POINT('Ctrl Pts',(3.87662433647851,-5.79731641090071,22.4833515156035));
#45751=CARTESIAN_POINT('Ctrl Pts',(3.75061024319318,-4.16456822152471,24.8234424569172));
#45752=CARTESIAN_POINT('Ctrl Pts',(3.61169875270454,-1.35007773082975,26.2278821221607));
#45753=CARTESIAN_POINT('Ctrl Pts',(3.47278726221591,1.79333824355105,26.1149949755885));
#45754=CARTESIAN_POINT('Ctrl Pts',(3.33387577172728,4.49983519042547,24.5122842181282));
#45755=CARTESIAN_POINT('Ctrl Pts',(3.19496428123863,6.11001713833909,21.8102254493376));
#45756=CARTESIAN_POINT('Ctrl Pts',(3.05605279075,6.23158824788668,18.6671333472082));
#45757=CARTESIAN_POINT('Ctrl Pts',(2.91714130026136,4.83492960625386,15.8487735173902));
#45758=CARTESIAN_POINT('Ctrl Pts',(2.77822980977273,2.26031541093747,14.041795584685));
#45759=CARTESIAN_POINT('Ctrl Pts',(2.63931831928409,-0.864989547684349,
13.6864416790982));
#45760=CARTESIAN_POINT('Ctrl Pts',(2.50040682879546,-3.77955323437126,14.8692882560822));
#45761=CARTESIAN_POINT('Ctrl Pts',(2.36721439988761,-5.69120430944527,17.2019907534407));
#45762=CARTESIAN_POINT('Ctrl Pts',(2.28032580114264,-6.11280516982525,19.109479946078));
#45763=CARTESIAN_POINT('Ctrl Pts',(2.23974103256055,-6.11358099250321,20.0001166795099));
#45764=CARTESIAN_POINT('Ctrl Pts',(4.13525896743946,-6.11343686380434,19.9998556839975));
#45765=CARTESIAN_POINT('Ctrl Pts',(4.09693819438009,-6.11259463033327,20.8408660932363));
#45766=CARTESIAN_POINT('Ctrl Pts',(4.01231359115783,-5.72621975022473,22.6988376413813));
#45767=CARTESIAN_POINT('Ctrl Pts',(3.8813851577727,-3.90353405789533,25.0370276152856));
#45768=CARTESIAN_POINT('Ctrl Pts',(3.74247366728407,-1.01867885543911,26.2905896963458));
#45769=CARTESIAN_POINT('Ctrl Pts',(3.60356217679543,2.11436163853657,26.0115472384233));
#45770=CARTESIAN_POINT('Ctrl Pts',(3.46465068630679,4.73227073773,24.2678846051763));
#45771=CARTESIAN_POINT('Ctrl Pts',(3.32573919581815,6.19723552447633,21.4844181326321));
#45772=CARTESIAN_POINT('Ctrl Pts',(3.18682770532951,6.15234006719685,18.3392962227209));
#45773=CARTESIAN_POINT('Ctrl Pts',(3.04791621484088,4.60852244721424,15.5987790112615));
#45774=CARTESIAN_POINT('Ctrl Pts',(2.90900472435224,1.94190986497335,13.9305509792932));
#45775=CARTESIAN_POINT('Ctrl Pts',(2.77009323386361,-1.19781891413772,13.7410499932924));
#45776=CARTESIAN_POINT('Ctrl Pts',(2.63118174337496,-4.04571770703044,15.0764450267472));
#45777=CARTESIAN_POINT('Ctrl Pts',(2.50290365456693,-5.76539070545534,17.4173429185103));
#45778=CARTESIAN_POINT('Ctrl Pts',(2.42092939592176,-6.11244943091349,19.2172463881382));
#45779=CARTESIAN_POINT('Ctrl Pts',(2.38525896743947,-6.11325364908754,20.0001583732729));
#45780=CARTESIAN_POINT('Origin',(53.8647410325606,0.,20.));
#45781=CARTESIAN_POINT('',(5.88525896743946,-6.11277390858896,20.0000683331812));
#45782=CARTESIAN_POINT('',(5.73974103256054,-6.1129851143326,20.0001404084395));
#45783=CARTESIAN_POINT('',(53.8647410325606,-6.11325,19.9999999999994));
#45784=CARTESIAN_POINT('Ctrl Pts',(5.73974103256054,-6.1129851143326,20.0001404084395));
#45785=CARTESIAN_POINT('Ctrl Pts',(5.72495105838506,-6.11325962756252,20.3247989551979));
#45786=CARTESIAN_POINT('Ctrl Pts',(5.6638572540467,-6.00826961576545,21.6657090484576));
#45787=CARTESIAN_POINT('Ctrl Pts',(5.55645961954546,-5.04185590001004,23.897295817673));
#45788=CARTESIAN_POINT('Ctrl Pts',(5.41754812905682,-2.56349596308158,25.8341849520033));
#45789=CARTESIAN_POINT('Ctrl Pts',(5.27863663856818,0.539419975483812,26.3496654791388));
#45790=CARTESIAN_POINT('Ctrl Pts',(5.13972514807955,3.51091460972764,25.3181485697674));
#45791=CARTESIAN_POINT('Ctrl Pts',(5.00081365759091,5.62702939460967,22.9909473079805));
#45792=CARTESIAN_POINT('Ctrl Pts',(4.86190216710228,6.37220580845331,19.9350481591359));
#45793=CARTESIAN_POINT('Ctrl Pts',(4.72299067661364,5.56489318441634,16.8949735181558));
#45794=CARTESIAN_POINT('Ctrl Pts',(4.584079186125,3.40178071249615,14.6113903842451));
#45795=CARTESIAN_POINT('Ctrl Pts',(4.44516769563636,0.409877171332637,13.6406583429304));
#45796=CARTESIAN_POINT('Ctrl Pts',(4.30625620514773,-2.68188658064232,14.2192811886858));
#45797=CARTESIAN_POINT('Ctrl Pts',(4.16734471465908,-5.12025029463462,16.2062864463399));
#45798=CARTESIAN_POINT('Ctrl Pts',(4.06183965713003,-6.02474970735384,18.4174444764408));
#45799=CARTESIAN_POINT('Ctrl Pts',(4.00263842976385,-6.1133719909142,19.7167469194031));
#45800=CARTESIAN_POINT('Ctrl Pts',(3.98974103256054,-6.11310094248279,19.999845624611));
#45801=CARTESIAN_POINT('Ctrl Pts',(5.88525896743946,-6.11277390858896,20.0000683331812));
#45802=CARTESIAN_POINT('Ctrl Pts',(5.86555465316417,-6.11294380838857,20.4326456386692));
#45803=CARTESIAN_POINT('Ctrl Pts',(5.79954650872601,-5.96128629022551,21.8816334848052));
#45804=CARTESIAN_POINT('Ctrl Pts',(5.68723453412497,-4.82859400298248,24.1585941485866));
#45805=CARTESIAN_POINT('Ctrl Pts',(5.54832304363634,-2.25122745380935,25.9616440928248));
#45806=CARTESIAN_POINT('Ctrl Pts',(5.4094115531477,0.874615721648888,26.3122319885871));
#45807=CARTESIAN_POINT('Ctrl Pts',(5.27050006265906,3.78737235203403,25.1249425367847));
#45808=CARTESIAN_POINT('Ctrl Pts',(5.13158857217043,5.77739449523354,22.6890403836206));
#45809=CARTESIAN_POINT('Ctrl Pts',(4.99267708168179,6.35984414454672,19.5979952794158));
#45810=CARTESIAN_POINT('Ctrl Pts',(4.85376559119316,5.39281648351639,16.604892385592));
#45811=CARTESIAN_POINT('Ctrl Pts',(4.71485410070452,3.11191279185723,14.4389547642397));
#45812=CARTESIAN_POINT('Ctrl Pts',(4.57594261021589,0.0728398505813112,
13.6278794978073));
#45813=CARTESIAN_POINT('Ctrl Pts',(4.43703111972725,-2.98397938969178,14.3692724857092));
#45814=CARTESIAN_POINT('Ctrl Pts',(4.29811962923861,-5.31379836804421,16.4825048341088));
#45815=CARTESIAN_POINT('Ctrl Pts',(4.19752891180935,-6.06341926380413,18.6333427654839));
#45816=CARTESIAN_POINT('Ctrl Pts',(4.14324202454297,-6.11361231949996,19.8246547789638));
#45817=CARTESIAN_POINT('Ctrl Pts',(4.13525896743946,-6.11343686380434,19.9998556839975));
#45818=CARTESIAN_POINT('Origin',(53.8647410325606,0.,20.));
#45819=CARTESIAN_POINT('',(7.63525896743946,-6.11376652953962,20.0000252316214));
#45820=CARTESIAN_POINT('',(7.48974103256053,-6.11368021756426,19.9999161056822));
#45821=CARTESIAN_POINT('',(53.8647410325606,-6.11325,19.9999999999994));
#45822=CARTESIAN_POINT('Ctrl Pts',(7.48974103256053,-6.11368021756426,19.9999161056822));
#45823=CARTESIAN_POINT('Ctrl Pts',(7.44726368700626,-6.11305136260232,20.9320417877776));
#45824=CARTESIAN_POINT('Ctrl Pts',(7.35848251128911,-5.66082090355657,22.8808510542445));
#45825=CARTESIAN_POINT('Ctrl Pts',(7.2233975054091,-3.67418420606118,25.206687625242));
#45826=CARTESIAN_POINT('Ctrl Pts',(7.08448601492046,-0.73611510378342,26.3298783685707));
#45827=CARTESIAN_POINT('Ctrl Pts',(6.94557452443182,2.38129701778703,25.9108924977533));
#45828=CARTESIAN_POINT('Ctrl Pts',(6.80666303394318,4.91854308270761,24.0518094168491));
#45829=CARTESIAN_POINT('Ctrl Pts',(6.66775154345454,6.2574624695857,21.2055658624248));
#45830=CARTESIAN_POINT('Ctrl Pts',(6.5288400529659,6.07184825208871,18.0656048980302));
#45831=CARTESIAN_POINT('Ctrl Pts',(6.38992856247727,4.40692245326515,15.3969292751659));
#45832=CARTESIAN_POINT('Ctrl Pts',(6.25101707198863,1.66831840155036,13.8497203870096));
#45833=CARTESIAN_POINT('Ctrl Pts',(6.11210558150001,-1.47674553359532,13.8009316638769));
#45834=CARTESIAN_POINT('Ctrl Pts',(5.97319409101137,-4.26202334105436,15.2624497208763));
#45835=CARTESIAN_POINT('Ctrl Pts',(5.84907257469821,-5.82293180962636,17.5996983337315));
#45836=CARTESIAN_POINT('Ctrl Pts',(5.77125488854794,-6.11240019306826,19.3083716084245));
#45837=CARTESIAN_POINT('Ctrl Pts',(5.73974103256054,-6.1129851143326,20.0001404084395));
#45838=CARTESIAN_POINT('Ctrl Pts',(7.63525896743946,-6.11376652953962,20.0000252316214));
#45839=CARTESIAN_POINT('Ctrl Pts',(7.63417111194827,-6.1137720723984,20.0238962246036));
#45840=CARTESIAN_POINT('Ctrl Pts',(7.5867794262942,-6.10780882306453,21.0638170421152));
#45841=CARTESIAN_POINT('Ctrl Pts',(7.49308391047725,-5.56015202049796,23.1135084466321));
#45842=CARTESIAN_POINT('Ctrl Pts',(7.35417241998862,-3.39355996620412,25.3937905126241));
#45843=CARTESIAN_POINT('Ctrl Pts',(7.21526092949997,-0.400179699901651,
26.3599592409137));
#45844=CARTESIAN_POINT('Ctrl Pts',(7.07634943901134,2.69069813882,25.7766226174165));
#45845=CARTESIAN_POINT('Ctrl Pts',(6.93743794852271,5.12602914017768,23.7859015560823));
#45846=CARTESIAN_POINT('Ctrl Pts',(6.79852645803408,6.31248270612288,20.8728043441669));
#45847=CARTESIAN_POINT('Ctrl Pts',(6.65961496754543,5.96099784106742,17.7470619011862));
#45848=CARTESIAN_POINT('Ctrl Pts',(6.5207034770568,4.15720837674583,15.1702128565938));
#45849=CARTESIAN_POINT('Ctrl Pts',(6.38179198656816,1.34057961829449,13.7700664830746));
#45850=CARTESIAN_POINT('Ctrl Pts',(6.24288049607952,-1.80266055610438,13.8877467119104));
#45851=CARTESIAN_POINT('Ctrl Pts',(6.10396900559088,-4.50671046633138,15.4945825819403));
#45852=CARTESIAN_POINT('Ctrl Pts',(5.98476182937753,-5.88495397728115,17.8154640682276));
#45853=CARTESIAN_POINT('Ctrl Pts',(5.91185848332706,-6.11254455514097,19.416117694291));
#45854=CARTESIAN_POINT('Ctrl Pts',(5.88525896743946,-6.11277390858896,20.0000683331812));
#45855=CARTESIAN_POINT('Origin',(53.8647410325606,0.,20.));
#45856=CARTESIAN_POINT('',(9.38525896743945,-6.11284857941777,19.9998944676288));
#45857=CARTESIAN_POINT('',(9.23974103256053,-6.11272951804558,19.9999855091883));
#45858=CARTESIAN_POINT('',(53.8647410325606,-6.11325,19.9999999999994));
#45859=CARTESIAN_POINT('Ctrl Pts',(9.23974103256053,-6.11272951804558,19.9999855091883));
#45860=CARTESIAN_POINT('Ctrl Pts',(9.21588014579035,-6.11268627364501,20.523824732368));
#45861=CARTESIAN_POINT('Ctrl Pts',(9.14571542885729,-5.91674747053061,22.0642447887842));
#45862=CARTESIAN_POINT('Ctrl Pts',(9.02924688176137,-4.63763254324486,24.3705365804159));
#45863=CARTESIAN_POINT('Ctrl Pts',(8.89033539127272,-1.98215097657166,26.0564265960212));
#45864=CARTESIAN_POINT('Ctrl Pts',(8.7514239007841,1.15625090922707,26.2667622774308));
#45865=CARTESIAN_POINT('Ctrl Pts',(8.61251241029546,4.01295020795098,24.9502986006324));
#45866=CARTESIAN_POINT('Ctrl Pts',(8.47360091980683,5.8919564762427,22.4277715067483));
#45867=CARTESIAN_POINT('Ctrl Pts',(8.33468942931819,6.33547900216983,19.3137555683411));
#45868=CARTESIAN_POINT('Ctrl Pts',(8.19577793882954,5.23546040650557,16.3669324340401));
#45869=CARTESIAN_POINT('Ctrl Pts',(8.05686644834092,2.85990314594527,14.3052498208675));
#45870=CARTESIAN_POINT('Ctrl Pts',(7.91795495785227,-0.212425125618811,
13.6310046967419));
#45871=CARTESIAN_POINT('Ctrl Pts',(7.77904346736364,-3.23299931252101,14.5084664207386));
#45872=CARTESIAN_POINT('Ctrl Pts',(7.64013197687499,-5.46590339851313,16.7238550634869));
#45873=CARTESIAN_POINT('Ctrl Pts',(7.54369783194064,-6.09154300913412,18.8159145025665));
#45874=CARTESIAN_POINT('Ctrl Pts',(7.49356751716914,-6.11373686667455,19.9159474741849));
#45875=CARTESIAN_POINT('Ctrl Pts',(7.48974103256053,-6.11368021756426,19.9999161056822));
#45876=CARTESIAN_POINT('Ctrl Pts',(9.38525896743944,-6.11284857941777,19.9998944676288));
#45877=CARTESIAN_POINT('Ctrl Pts',(9.35648374056947,-6.11245938709689,20.6315873376648));
#45878=CARTESIAN_POINT('Ctrl Pts',(9.28140468353662,-5.85828893938936,22.2800786383337));
#45879=CARTESIAN_POINT('Ctrl Pts',(9.16002179634088,-4.39989835807759,24.6097852202552));
#45880=CARTESIAN_POINT('Ctrl Pts',(9.02111030585225,-1.65893824958895,26.152816365076));
#45881=CARTESIAN_POINT('Ctrl Pts',(8.88219881536361,1.48619641390095,26.1968093046023));
#45882=CARTESIAN_POINT('Ctrl Pts',(8.74328732487498,4.26924238941132,24.7310458419625));
#45883=CARTESIAN_POINT('Ctrl Pts',(8.60437583438633,6.01215372256228,22.1126364937154));
#45884=CARTESIAN_POINT('Ctrl Pts',(8.4654643438977,6.29029711994617,18.9795160554453));
#45885=CARTESIAN_POINT('Ctrl Pts',(8.32655285340906,5.03590726004376,16.0950206906393));
#45886=CARTESIAN_POINT('Ctrl Pts',(8.18764136292043,2.55459676198038,14.1619129227137));
#45887=CARTESIAN_POINT('Ctrl Pts',(8.04872987243179,-0.549101585502231,
13.6511644542408));
#45888=CARTESIAN_POINT('Ctrl Pts',(7.90981838194317,-3.51901985465715,14.6872112218886));
#45889=CARTESIAN_POINT('Ctrl Pts',(7.7719947469457,-5.61503946859896,16.9993862869652));
#45890=CARTESIAN_POINT('Ctrl Pts',(7.68047494211115,-6.11353614437879,19.0078436203562));
#45891=CARTESIAN_POINT('Ctrl Pts',(7.63525896743946,-6.11376652953962,20.0000252316214));
#45892=CARTESIAN_POINT('Origin',(53.8647410325606,0.,20.));
#45893=CARTESIAN_POINT('',(11.1352589674394,-6.11328663918834,20.0001573543196));
#45894=CARTESIAN_POINT('',(10.9897410325605,-6.11360815273101,20.0001092168757));
#45895=CARTESIAN_POINT('',(53.8647410325606,-6.11325,19.9999999999994));
#45896=CARTESIAN_POINT('Ctrl Pts',(10.9897410325605,-6.11360815273101,20.0001092168757));
#45897=CARTESIAN_POINT('Ctrl Pts',(10.9844966045744,-6.11370363815739,20.1151972238524));
#45898=CARTESIAN_POINT('Ctrl Pts',(10.9329483464255,-6.08241679304912,21.2463623732547));
#45899=CARTESIAN_POINT('Ctrl Pts',(10.8350962581136,-5.41523157606947,23.3592398819462));
#45900=CARTESIAN_POINT('Ctrl Pts',(10.696184767625,-3.14875378158332,25.5402685160452));
#45901=CARTESIAN_POINT('Ctrl Pts',(10.5572732771364,-0.115131002167762,
26.3714967204933));
#45902=CARTESIAN_POINT('Ctrl Pts',(10.4183617866477,2.94654165889923,25.6504086453361));
#45903=CARTESIAN_POINT('Ctrl Pts',(10.2794502961591,5.29033518005657,23.5526862075862));
#45904=CARTESIAN_POINT('Ctrl Pts',(10.1405388056704,6.34522064949098,20.5894069190218));
#45905=CARTESIAN_POINT('Ctrl Pts',(10.0016273151818,5.854191596171,17.4825277832241));
#45906=CARTESIAN_POINT('Ctrl Pts',(9.86271582469318,3.9368796273414,14.9889916776419));
#45907=CARTESIAN_POINT('Ctrl Pts',(9.72380433420454,1.06040804430175,13.716309970527));
#45908=CARTESIAN_POINT('Ctrl Pts',(9.58489284371591,-2.07441549941601,13.974551805658));
#45909=CARTESIAN_POINT('Ctrl Pts',(9.44598135322726,-4.70383990511773,15.7008005682523));
#45910=CARTESIAN_POINT('Ctrl Pts',(9.33093074950883,-5.93244129797807,17.998045990015));
#45911=CARTESIAN_POINT('Ctrl Pts',(9.26218397595324,-6.1127701926292,19.5072756553621));
#45912=CARTESIAN_POINT('Ctrl Pts',(9.23974103256053,-6.11272951804558,19.9999855091883));
#45913=CARTESIAN_POINT('Ctrl Pts',(11.1352589674394,-6.11328663918834,20.0001573543196));
#45914=CARTESIAN_POINT('Ctrl Pts',(11.1251001993536,-6.11351667627268,20.2231234942924));
#45915=CARTESIAN_POINT('Ctrl Pts',(11.0686376011048,-6.04702917925912,21.4622364723876));
#45916=CARTESIAN_POINT('Ctrl Pts',(10.9658711726931,-5.22991444725156,23.6410465820594));
#45917=CARTESIAN_POINT('Ctrl Pts',(10.8269596822045,-2.85121621531744,25.699104441209));
#45918=CARTESIAN_POINT('Ctrl Pts',(10.6880481917159,0.222136591808738,26.3686639629421));
#45919=CARTESIAN_POINT('Ctrl Pts',(10.5491367012273,3.24136926627416,25.486597362478));
#45920=CARTESIAN_POINT('Ctrl Pts',(10.4102252107386,5.47089263051329,23.267806475863));
#45921=CARTESIAN_POINT('Ctrl Pts',(10.27131372025,6.36751792278091,20.2528652632554));
#45922=CARTESIAN_POINT('Ctrl Pts',(10.1324022297613,5.71279630774815,17.1763173541497));
#45923=CARTESIAN_POINT('Ctrl Pts',(9.99349073927272,3.66624054453745,14.7877158934027));
#45924=CARTESIAN_POINT('Ctrl Pts',(9.85457924878407,0.726462178868265,13.6690065518142));
#45925=CARTESIAN_POINT('Ctrl Pts',(9.71566775829543,-2.39030742076759,14.0927454962123));
#45926=CARTESIAN_POINT('Ctrl Pts',(9.5767562678068,-4.92471571892393,15.9556953099351));
#45927=CARTESIAN_POINT('Ctrl Pts',(9.46662000418813,-5.98283846110334,18.2139615092778));
#45928=CARTESIAN_POINT('Ctrl Pts',(9.40278757073235,-6.11308565827133,19.6150949394844));
#45929=CARTESIAN_POINT('Ctrl Pts',(9.38525896743944,-6.11284857941777,19.9998944676288));
#45930=CARTESIAN_POINT('Origin',(53.8647410325606,0.,20.));
#45931=CARTESIAN_POINT('',(12.8852589674394,-6.11340458852378,19.9998516759371));
#45932=CARTESIAN_POINT('',(12.7397410325605,-6.11307060053939,19.9998482593178));
#45933=CARTESIAN_POINT('',(53.8647410325606,-6.11325,19.9999999999994));
#45934=CARTESIAN_POINT('Ctrl Pts',(12.7397410325605,-6.11307060053939,19.9998482593178));
#45935=CARTESIAN_POINT('Ctrl Pts',(12.7068092331956,-6.11239576113666,20.7227136938253));
#45936=CARTESIAN_POINT('Ctrl Pts',(12.6275736036679,-5.80383176099062,22.462526520406));
#45937=CARTESIAN_POINT('Ctrl Pts',(12.5020341439773,-4.1891728722864,24.8020887385612));
#45938=CARTESIAN_POINT('Ctrl Pts',(12.3631226534886,-1.38189913347912,26.2208986804004));
#45939=CARTESIAN_POINT('Ctrl Pts',(12.224211163,1.76205287980219,26.124083217568));
#45940=CARTESIAN_POINT('Ctrl Pts',(12.0852996725114,4.4767080589433,24.5352299348445));
#45941=CARTESIAN_POINT('Ctrl Pts',(11.9463881820227,6.1006828055596,21.8414382728907));
#45942=CARTESIAN_POINT('Ctrl Pts',(11.8074766915341,6.23832087945686,18.6990087579656));
#45943=CARTESIAN_POINT('Ctrl Pts',(11.6685652010455,4.85608890030431,15.8735455655904));
#45944=CARTESIAN_POINT('Ctrl Pts',(11.5296537105568,2.29074623525794,14.0534289466476));
#45945=CARTESIAN_POINT('Ctrl Pts',(11.3907422200682,-0.832701193775514,
13.6821020640721));
#45946=CARTESIAN_POINT('Ctrl Pts',(11.2518307295795,-3.75327390186831,14.8500329491858));
#45947=CARTESIAN_POINT('Ctrl Pts',(11.118163667077,-5.68368017920984,17.1812096389043));
#45948=CARTESIAN_POINT('Ctrl Pts',(11.0308004347373,-6.11286058320882,19.0990681926252));
#45949=CARTESIAN_POINT('Ctrl Pts',(10.9897410325605,-6.11360815273101,20.0001092168757));
#45950=CARTESIAN_POINT('Ctrl Pts',(12.8852589674394,-6.11340458852378,19.9998516759371));
#45951=CARTESIAN_POINT('Ctrl Pts',(12.8474128279748,-6.11256107075738,20.8304581458768));
#45952=CARTESIAN_POINT('Ctrl Pts',(12.7632628583472,-5.73337822611735,22.6780379247862));
#45953=CARTESIAN_POINT('Ctrl Pts',(12.6328090585568,-3.92923403963699,25.0170056009591));
#45954=CARTESIAN_POINT('Ctrl Pts',(12.4938975680681,-1.05082517123617,26.285299658552));
#45955=CARTESIAN_POINT('Ctrl Pts',(12.3549860775795,2.0836009395627,26.0222780127582));
#45956=CARTESIAN_POINT('Ctrl Pts',(12.2160745870909,4.71039002242726,24.2920218050372));
#45957=CARTESIAN_POINT('Ctrl Pts',(12.0771630966022,6.1895656895012,21.5160811039145));
#45958=CARTESIAN_POINT('Ctrl Pts',(11.9382516061136,6.1607497487956,18.370770773951));
#45959=CARTESIAN_POINT('Ctrl Pts',(11.799340115625,4.63096275699136,15.6223968565371));
#45960=CARTESIAN_POINT('Ctrl Pts',(11.6604286251363,1.97291356977519,13.9405579972662));
#45961=CARTESIAN_POINT('Ctrl Pts',(11.5215171346477,-1.1658053857806,13.7350081292326));
#45962=CARTESIAN_POINT('Ctrl Pts',(11.3826056441591,-4.02049395435078,15.0558262873028));
#45963=CARTESIAN_POINT('Ctrl Pts',(11.2538529217563,-5.75851899348006,17.3965308011831));
#45964=CARTESIAN_POINT('Ctrl Pts',(11.1714040295164,-6.11246816350081,19.2068402018603));
#45965=CARTESIAN_POINT('Ctrl Pts',(11.1352589674394,-6.11328663918834,20.0001573543196));
#45966=CARTESIAN_POINT('Origin',(53.8647410325606,0.,20.));
#45967=CARTESIAN_POINT('',(14.6352589674394,-6.11278735830072,20.0000770013196));
#45968=CARTESIAN_POINT('',(14.4897410325605,-6.11301278051747,20.0001447615033));
#45969=CARTESIAN_POINT('',(53.8647410325606,-6.11325,19.9999999999994));
#45970=CARTESIAN_POINT('Ctrl Pts',(14.4897410325605,-6.11301278051747,20.0001447615033));
#45971=CARTESIAN_POINT('Ctrl Pts',(14.4754256919797,-6.11328857136773,20.3143804240189));
#45972=CARTESIAN_POINT('Ctrl Pts',(14.4148065212361,-6.01248627071629,21.6448549593419));
#45973=CARTESIAN_POINT('Ctrl Pts',(14.3078835203295,-5.06171431056786,23.8714692101462));
#45974=CARTESIAN_POINT('Ctrl Pts',(14.1689720298409,-2.59328879522498,25.8210032495677));
#45975=CARTESIAN_POINT('Ctrl Pts',(14.0300605393523,0.506951282871708,26.3523401989906));
#45976=CARTESIAN_POINT('Ctrl Pts',(13.8911490488636,3.48368054963307,25.3360280579309));
#45977=CARTESIAN_POINT('Ctrl Pts',(13.752237558375,5.6116651230563,23.0196755046844));
#45978=CARTESIAN_POINT('Ctrl Pts',(13.6133260678864,6.37245459172572,19.967625885163));
#45979=CARTESIAN_POINT('Ctrl Pts',(13.4744145773977,5.58069441033177,16.9234637162209));
#45980=CARTESIAN_POINT('Ctrl Pts',(13.3355030869091,3.42928465762181,14.6288518598053));
#45981=CARTESIAN_POINT('Ctrl Pts',(13.1965915964205,0.442382926346631,13.6428368784973));
#45982=CARTESIAN_POINT('Ctrl Pts',(13.0576801059318,-2.65229853840607,14.205646017882));
#45983=CARTESIAN_POINT('Ctrl Pts',(12.9187686154432,-5.10078863240939,16.1801595668928));
#45984=CARTESIAN_POINT('Ctrl Pts',(12.8127889243194,-6.02070026988043,18.3965909557952));
#45985=CARTESIAN_POINT('Ctrl Pts',(12.7531130633585,-6.11334462058844,19.7063271326415));
#45986=CARTESIAN_POINT('Ctrl Pts',(12.7397410325605,-6.11307060053939,19.9998482593178));
#45987=CARTESIAN_POINT('Ctrl Pts',(14.6352589674394,-6.11278735830072,20.0000770013196));
#45988=CARTESIAN_POINT('Ctrl Pts',(14.6160292867589,-6.11297471112037,20.4222318127276));
#45989=CARTESIAN_POINT('Ctrl Pts',(14.5504957759154,-5.96609040238597,21.8607796245411));
#45990=CARTESIAN_POINT('Ctrl Pts',(14.4386584349091,-4.84979104615329,24.133854393535));
#45991=CARTESIAN_POINT('Ctrl Pts',(14.2997469444204,-2.28167598106183,25.950057147267));
#45992=CARTESIAN_POINT('Ctrl Pts',(14.1608354539318,0.842334021367499,26.3166208319594));
#45993=CARTESIAN_POINT('Ctrl Pts',(14.0219239634432,3.7611224139311,25.1442378955218));
#45994=CARTESIAN_POINT('Ctrl Pts',(13.8830124729545,5.76357170928461,22.7185412430624));
#45995=CARTESIAN_POINT('Ctrl Pts',(13.7441009824659,6.36181621799531,19.6305142130623));
#45996=CARTESIAN_POINT('Ctrl Pts',(13.6051894919773,5.41010295127669,16.6325066600089));
#45997=CARTESIAN_POINT('Ctrl Pts',(13.4662780014886,3.14030207437455,14.4549365900852));
#45998=CARTESIAN_POINT('Ctrl Pts',(13.327366511,0.105415339819669,13.6283351512789));
#45999=CARTESIAN_POINT('Ctrl Pts',(13.1884550205113,-2.95515420605895,14.354090953911));
#46000=CARTESIAN_POINT('Ctrl Pts',(13.0495435300227,-5.29574629859371,16.4553848616206));
#46001=CARTESIAN_POINT('Ctrl Pts',(12.9484781789987,-6.05994210690123,18.6124928036776));
#46002=CARTESIAN_POINT('Ctrl Pts',(12.8937166581377,-6.11359309420672,19.8142313533877));
#46003=CARTESIAN_POINT('Ctrl Pts',(12.8852589674394,-6.11340458852378,19.9998516759371));
#46004=CARTESIAN_POINT('Origin',(53.8647410325606,0.,20.));
#46005=CARTESIAN_POINT('',(16.3852589674394,-6.1137723837536,20.0000142741886));
#46006=CARTESIAN_POINT('',(16.2397410325605,-6.11365777682639,19.9999071565179));
#46007=CARTESIAN_POINT('',(53.8647410325606,-6.11325,19.9999999999994));
#46008=CARTESIAN_POINT('Ctrl Pts',(16.2397410325605,-6.11365777682639,19.9999071565179));
#46009=CARTESIAN_POINT('Ctrl Pts',(16.197738320601,-6.11298318269978,20.9216272610411));
#46010=CARTESIAN_POINT('Ctrl Pts',(16.1094317784785,-5.66853645373843,22.8600809899514));
#46011=CARTESIAN_POINT('Ctrl Pts',(15.9748214061932,-3.70075454447885,25.1878359080099));
#46012=CARTESIAN_POINT('Ctrl Pts',(15.8359099157046,-0.768465969166765,
26.3260323790785));
#46013=CARTESIAN_POINT('Ctrl Pts',(15.6969984252159,2.35104741164878,25.9229892516446));
#46014=CARTESIAN_POINT('Ctrl Pts',(15.5580869347273,4.89776458282526,24.0769017278002));
#46015=CARTESIAN_POINT('Ctrl Pts',(15.4191754442386,6.25121743493832,21.2375403783475));
#46016=CARTESIAN_POINT('Ctrl Pts',(15.28026395375,6.08165818843483,18.096671524418));
#46017=CARTESIAN_POINT('Ctrl Pts',(15.1413524632613,4.43039732188061,15.4195191107057));
#46018=CARTESIAN_POINT('Ctrl Pts',(15.0024409727728,1.69973891506645,13.8583297689044));
#46019=CARTESIAN_POINT('Ctrl Pts',(14.8635294822841,-1.44503449559759,13.7934630498602));
#46020=CARTESIAN_POINT('Ctrl Pts',(14.7246179917955,-4.23774768077446,15.2407227228278));
#46021=CARTESIAN_POINT('Ctrl Pts',(14.6000218418876,-5.81659899729983,17.5788677726848));
#46022=CARTESIAN_POINT('Ctrl Pts',(14.5217295221426,-6.11239650927398,19.2979662726303));
#46023=CARTESIAN_POINT('Ctrl Pts',(14.4897410325605,-6.11301278051747,20.0001447615033));
#46024=CARTESIAN_POINT('Ctrl Pts',(16.3852589674394,-6.1137723837536,20.0000142741886));
#46025=CARTESIAN_POINT('Ctrl Pts',(16.384645745543,-6.11377420047576,20.0134702661335));
#46026=CARTESIAN_POINT('Ctrl Pts',(16.3377286934836,-6.11044645114222,21.0429751237547));
#46027=CARTESIAN_POINT('Ctrl Pts',(16.2445078112613,-5.57599667105201,23.0850423761618));
#46028=CARTESIAN_POINT('Ctrl Pts',(16.1055963207727,-3.42109050526117,25.3763709966026));
#46029=CARTESIAN_POINT('Ctrl Pts',(15.9666848302841,-0.432688738940727,
26.3578302740393));
#46030=CARTESIAN_POINT('Ctrl Pts',(15.8277733397954,2.66113092256575,25.7903028894231));
#46031=CARTESIAN_POINT('Ctrl Pts',(15.6888618493068,5.10660734001576,23.8120580810363));
#46032=CARTESIAN_POINT('Ctrl Pts',(15.5499503588182,6.30793814220377,20.9050644907565));
#46033=CARTESIAN_POINT('Ctrl Pts',(15.4110388683295,5.97243772585063,17.7775659854265));
#46034=CARTESIAN_POINT('Ctrl Pts',(15.2721273778409,4.1818455598703,15.1915290318346));
#46035=CARTESIAN_POINT('Ctrl Pts',(15.1332158873523,1.37241163250246,13.777001394081));
#46036=CARTESIAN_POINT('Ctrl Pts',(14.9943043968636,-1.77138908698832,13.8786107752573));
#46037=CARTESIAN_POINT('Ctrl Pts',(14.855392906375,-4.48361835037166,15.4716016267882));
#46038=CARTESIAN_POINT('Ctrl Pts',(14.7357110965669,-5.87924374865939,17.7946193487845));
#46039=CARTESIAN_POINT('Ctrl Pts',(14.6623331169217,-6.11252357762077,19.4057102690483));
#46040=CARTESIAN_POINT('Ctrl Pts',(14.6352589674394,-6.11278735830072,20.0000770013196));
#46041=CARTESIAN_POINT('Origin',(53.8647410325606,0.,20.));
#46042=CARTESIAN_POINT('',(18.1352589674394,-6.11282951797325,19.9999019817517));
#46043=CARTESIAN_POINT('',(17.9897410325605,-6.11272775120567,19.9999952045773));
#46044=CARTESIAN_POINT('',(53.8647410325606,-6.11325,19.9999999999994));
#46045=CARTESIAN_POINT('Ctrl Pts',(17.9897410325605,-6.11272775120567,19.9999952045773));
#46046=CARTESIAN_POINT('Ctrl Pts',(17.966354779385,-6.11271372992993,20.5134147996941));
#46047=CARTESIAN_POINT('Ctrl Pts',(17.8966646960467,-5.92205872661351,22.0433945389182));
#46048=CARTESIAN_POINT('Ctrl Pts',(17.7806707825455,-4.65991560350942,24.3467703154281));
#46049=CARTESIAN_POINT('Ctrl Pts',(17.6417592920568,-2.01308758044197,26.0462140220462));
#46050=CARTESIAN_POINT('Ctrl Pts',(17.5028478015682,1.12419798509589,26.2725915296011));
#46051=CARTESIAN_POINT('Ctrl Pts',(17.3639363110796,3.98759016100821,24.9707494721368));
#46052=CARTESIAN_POINT('Ctrl Pts',(17.2250248205909,5.87946788829534,22.4578614601765));
#46053=CARTESIAN_POINT('Ctrl Pts',(17.0861133301023,6.33890452382744,19.3461536535871));
#46054=CARTESIAN_POINT('Ctrl Pts',(16.9472018396136,5.25396546258616,16.3937453605064));
#46055=CARTESIAN_POINT('Ctrl Pts',(16.808290349125,2.88897926676432,14.3199450352023));
#46056=CARTESIAN_POINT('Ctrl Pts',(16.6693788586364,-0.179861885588608,
13.630001938067));
#46057=CARTESIAN_POINT('Ctrl Pts',(16.5304673681478,-3.2048824812767,14.4920099956406));
#46058=CARTESIAN_POINT('Ctrl Pts',(16.3915558776591,-5.44908320556687,16.6959543245097));
#46059=CARTESIAN_POINT('Ctrl Pts',(16.29464709913,-6.08854185718405,18.7950688508708));
#46060=CARTESIAN_POINT('Ctrl Pts',(16.2440421507638,-6.11372685591539,19.9055221291));
#46061=CARTESIAN_POINT('Ctrl Pts',(16.2397410325605,-6.11365777682639,19.9999071565179));
#46062=CARTESIAN_POINT('Ctrl Pts',(18.1352589674394,-6.11282951797326,19.9999019817517));
#46063=CARTESIAN_POINT('Ctrl Pts',(18.1069583741642,-6.11247543877291,20.6211809276915));
#46064=CARTESIAN_POINT('Ctrl Pts',(18.032353950726,-5.86421293859169,22.2592379783294));
#46065=CARTESIAN_POINT('Ctrl Pts',(17.911445697125,-4.42340764526233,24.5872312065266));
#46066=CARTESIAN_POINT('Ctrl Pts',(17.7725342066364,-1.6903718544226,26.1442549045489));
#46067=CARTESIAN_POINT('Ctrl Pts',(17.6336227161477,1.45449680133364,26.2043262642456));
#46068=CARTESIAN_POINT('Ctrl Pts',(17.4947112256591,4.24499988768104,24.7528098312351));
#46069=CARTESIAN_POINT('Ctrl Pts',(17.3557997351704,6.00127464093126,22.1433450544447));
#46070=CARTESIAN_POINT('Ctrl Pts',(17.2168882446818,6.29543197779222,19.0116875234582));
#46071=CARTESIAN_POINT('Ctrl Pts',(17.0779767541932,5.05580502895429,16.1208169871096));
#46072=CARTESIAN_POINT('Ctrl Pts',(16.9390652637045,2.5844096594071,14.1750491804084));
#46073=CARTESIAN_POINT('Ctrl Pts',(16.8001537732159,-0.516637009270994,
13.6484402278693));
#46074=CARTESIAN_POINT('Ctrl Pts',(16.6612422827273,-3.49181308971526,14.6692902269219));
#46075=CARTESIAN_POINT('Ctrl Pts',(16.5229440141351,-5.6068847690672,16.9786451178929));
#46076=CARTESIAN_POINT('Ctrl Pts',(16.4309495757058,-6.11363702143042,18.9974204980683));
#46077=CARTESIAN_POINT('Ctrl Pts',(16.3852589674394,-6.1137723837536,20.0000142741886));
#46078=CARTESIAN_POINT('Origin',(53.8647410325606,0.,20.));
#46079=CARTESIAN_POINT('',(19.8852589674394,-6.11331970325597,20.000155680082));
#46080=CARTESIAN_POINT('',(19.7397410325605,-6.11363390149491,20.0001012241782));
#46081=CARTESIAN_POINT('',(53.8647410325606,-6.11325,19.9999999999994));
#46082=CARTESIAN_POINT('Ctrl Pts',(19.7397410325605,-6.11363390149491,20.0001012241782));
#46083=CARTESIAN_POINT('Ctrl Pts',(19.7349712381691,-6.11371586791688,20.104772207252));
#46084=CARTESIAN_POINT('Ctrl Pts',(19.6838976136149,-6.08552537520897,21.2255156751894));
#46085=CARTESIAN_POINT('Ctrl Pts',(19.5865201588977,-5.43233438289444,23.3315114826968));
#46086=CARTESIAN_POINT('Ctrl Pts',(19.4476086684091,-3.17703636502164,25.5240986180776));
#46087=CARTESIAN_POINT('Ctrl Pts',(19.3086971779205,-0.14770274975791,26.3708248684634));
#46088=CARTESIAN_POINT('Ctrl Pts',(19.1697856874318,2.91761634788927,25.6653985255625));
#46089=CARTESIAN_POINT('Ctrl Pts',(19.0308741969432,5.27210350868496,23.5796857684201));
#46090=CARTESIAN_POINT('Ctrl Pts',(18.8919627064546,6.34212448150116,20.6218381365444));
#46091=CARTESIAN_POINT('Ctrl Pts',(18.7530512159659,5.86698526483596,17.5124892946733));
#46092=CARTESIAN_POINT('Ctrl Pts',(18.6141397254773,3.96244615387019,15.0091838258059));
#46093=CARTESIAN_POINT('Ctrl Pts',(18.4752282349886,1.09251854134113,13.7218132519219));
#46094=CARTESIAN_POINT('Ctrl Pts',(18.3363167445,-2.0435842560608,13.9640254311919));
#46095=CARTESIAN_POINT('Ctrl Pts',(18.1974052540114,-4.68179946933745,15.6768091256771));
#46096=CARTESIAN_POINT('Ctrl Pts',(18.0818800166982,-5.92724600164252,17.9771945968397));
#46097=CARTESIAN_POINT('Ctrl Pts',(18.0126586095479,-6.11274149148563,19.4968648822612));
#46098=CARTESIAN_POINT('Ctrl Pts',(17.9897410325605,-6.11272775120567,19.9999952045773));
#46099=CARTESIAN_POINT('Ctrl Pts',(19.8852589674394,-6.11331970325597,20.000155680082));
#46100=CARTESIAN_POINT('Ctrl Pts',(19.8755748329482,-6.11353913440155,20.2127011814972));
#46101=CARTESIAN_POINT('Ctrl Pts',(19.8195868682942,-6.05070320076175,21.4413850412945));
#46102=CARTESIAN_POINT('Ctrl Pts',(19.7172950734772,-5.24846036724355,23.6142619041474));
#46103=CARTESIAN_POINT('Ctrl Pts',(19.5783835829886,-2.8803147101225,25.6844535805079));
#46104=CARTESIAN_POINT('Ctrl Pts',(19.4394720925,0.189574918792307,26.3697163742558));
#46105=CARTESIAN_POINT('Ctrl Pts',(19.3005606020113,3.21327756126488,25.5030966421251));
#46106=CARTESIAN_POINT('Ctrl Pts',(19.1616491115227,5.45411500140619,23.2957328304541));
#46107=CARTESIAN_POINT('Ctrl Pts',(19.0227376210341,6.36614197849088,20.2854148699583));
#46108=CARTESIAN_POINT('Ctrl Pts',(18.8838261305454,5.72715727574455,17.2055600065159));
#46109=CARTESIAN_POINT('Ctrl Pts',(18.7449146400568,3.69283959787427,14.8065270730783));
#46110=CARTESIAN_POINT('Ctrl Pts',(18.6060031495682,0.758818871062057,13.6728032068524));
#46111=CARTESIAN_POINT('Ctrl Pts',(18.4670916590795,-2.36007629553962,14.0806026305434));
#46112=CARTESIAN_POINT('Ctrl Pts',(18.3281801685909,-4.90397550508568,15.9305713443019));
#46113=CARTESIAN_POINT('Ctrl Pts',(18.2175692713775,-5.9782391292396,18.1931071368928));
#46114=CARTESIAN_POINT('Ctrl Pts',(18.153262204327,-6.11305476313539,19.6046794530843));
#46115=CARTESIAN_POINT('Ctrl Pts',(18.1352589674394,-6.11282951797326,19.9999019817517));
#46116=CARTESIAN_POINT('Origin',(53.8647410325606,0.,20.));
#46117=CARTESIAN_POINT('',(21.6352589674394,-6.11337192102228,19.9998483128521));
#46118=CARTESIAN_POINT('',(21.4897410325605,-6.11304106492475,19.9998514866922));
#46119=CARTESIAN_POINT('',(53.8647410325606,-6.11325,19.9999999999994));
#46120=CARTESIAN_POINT('Ctrl Pts',(21.4897410325605,-6.11304106492475,19.9998514866922));
#46121=CARTESIAN_POINT('Ctrl Pts',(21.4572838667903,-6.11239501336448,20.7123084151566));
#46122=CARTESIAN_POINT('Ctrl Pts',(21.3785228708573,-5.81028586147664,22.441699581993));
#46123=CARTESIAN_POINT('Ctrl Pts',(21.2534580447614,-4.21366803405649,24.7806095119438));
#46124=CARTESIAN_POINT('Ctrl Pts',(21.1145465542727,-1.41368441857138,26.2137526480868));
#46125=CARTESIAN_POINT('Ctrl Pts',(20.9756350637841,1.73072146273936,26.1330113994131));
#46126=CARTESIAN_POINT('Ctrl Pts',(20.8367235732955,4.453463923361,24.5580571179221));
#46127=CARTESIAN_POINT('Ctrl Pts',(20.6978120828068,6.09118902430437,21.8726029683601));
#46128=CARTESIAN_POINT('Ctrl Pts',(20.5589005923182,6.2448904649721,18.7309181715043));
#46129=CARTESIAN_POINT('Ctrl Pts',(20.4199891018296,4.87712127505025,15.8984254638773));
#46130=CARTESIAN_POINT('Ctrl Pts',(20.2810776113409,2.32111718758555,14.0652177286431));
#46131=CARTESIAN_POINT('Ctrl Pts',(20.1421661208523,-0.800391074992589,
13.6779275760247));
#46132=CARTESIAN_POINT('Ctrl Pts',(20.0032546303637,-3.72689647556414,14.8309122403131));
#46133=CARTESIAN_POINT('Ctrl Pts',(19.8691129342664,-5.67609213148412,17.1604321151321));
#46134=CARTESIAN_POINT('Ctrl Pts',(19.781275068332,-6.11292016081293,19.0886555729594));
#46135=CARTESIAN_POINT('Ctrl Pts',(19.7397410325605,-6.11363390149491,20.0001012241782));
#46136=CARTESIAN_POINT('Ctrl Pts',(21.6352589674394,-6.11337192102228,19.9998483128521));
#46137=CARTESIAN_POINT('Ctrl Pts',(21.5978874615695,-6.11253093386954,20.8200506714862));
#46138=CARTESIAN_POINT('Ctrl Pts',(21.5142121255366,-5.74047386468237,22.6572353299736));
#46139=CARTESIAN_POINT('Ctrl Pts',(21.3842329593409,-3.95483132620118,24.9968524612595));
#46140=CARTESIAN_POINT('Ctrl Pts',(21.2453214688522,-1.08294402247514,26.2798453470195));
#46141=CARTESIAN_POINT('Ctrl Pts',(21.1064099783636,2.05278578321474,26.0328513877377));
#46142=CARTESIAN_POINT('Ctrl Pts',(20.967498487875,4.68838619551153,24.3160468278314));
#46143=CARTESIAN_POINT('Ctrl Pts',(20.8285869973864,6.18173408290928,21.5477044506284));
#46144=CARTESIAN_POINT('Ctrl Pts',(20.6896755068977,6.16899841191383,18.4022879070052));
#46145=CARTESIAN_POINT('Ctrl Pts',(20.5507640164091,4.65328203108421,15.646129115662));
#46146=CARTESIAN_POINT('Ctrl Pts',(20.4118525259204,2.00386571014259,13.9507233858905));
#46147=CARTESIAN_POINT('Ctrl Pts',(20.2729410354318,-1.13376138770991,13.7291300082018));
#46148=CARTESIAN_POINT('Ctrl Pts',(20.1340295449432,-3.99516512133005,15.0353367695678));
#46149=CARTESIAN_POINT('Ctrl Pts',(20.0048021889457,-5.75158500211091,17.3757212187838));
#46150=CARTESIAN_POINT('Ctrl Pts',(19.9218786631111,-6.1124899438408,19.1964337175973));
#46151=CARTESIAN_POINT('Ctrl Pts',(19.8852589674394,-6.11331970325597,20.000155680082));
#46152=CARTESIAN_POINT('Origin',(53.8647410325606,0.,20.));
#46153=CARTESIAN_POINT('',(23.3852589674394,-6.11280242905631,20.0000853877862));
#46154=CARTESIAN_POINT('',(23.2397410325605,-6.11304143026726,20.0001485574224));
#46155=CARTESIAN_POINT('',(53.8647410325606,-6.11325,19.9999999999994));
#46156=CARTESIAN_POINT('Ctrl Pts',(23.2397410325605,-6.11304143026726,20.0001485574224));
#46157=CARTESIAN_POINT('Ctrl Pts',(23.2259003255744,-6.11331703329572,20.3039614647346));
#46158=CARTESIAN_POINT('Ctrl Pts',(23.1657557884255,-6.01664684285281,21.6240010332314));
#46159=CARTESIAN_POINT('Ctrl Pts',(23.0593074211136,-5.08144042723737,23.8455414171941));
#46160=CARTESIAN_POINT('Ctrl Pts',(22.920395930625,-2.62301384869953,25.8076694083296));
#46161=CARTESIAN_POINT('Ctrl Pts',(22.7814844401364,0.474469340488402,26.3548488929206));
#46162=CARTESIAN_POINT('Ctrl Pts',(22.6425729496477,3.45635543942831,25.353768082692));
#46163=CARTESIAN_POINT('Ctrl Pts',(22.5036614591591,5.59615418399987,23.0483247785986));
#46164=CARTESIAN_POINT('Ctrl Pts',(22.3647499686705,6.37253682336279,20.0002044573261));
#46165=CARTESIAN_POINT('Ctrl Pts',(22.2258384781818,5.59634977820039,16.9520343231995));
#46166=CARTESIAN_POINT('Ctrl Pts',(22.0869269876932,3.45669897433838,14.6464537166729));
#46167=CARTESIAN_POINT('Ctrl Pts',(21.9480154972045,0.474877119159393,13.6451815660385));
#46168=CARTESIAN_POINT('Ctrl Pts',(21.8091040067159,-2.62264117521137,14.1921622893711));
#46169=CARTESIAN_POINT('Ctrl Pts',(21.6701925162273,-5.08119365504295,16.1541325234911));
#46170=CARTESIAN_POINT('Ctrl Pts',(21.5637381915088,-6.01659496814579,18.3757372179489));
#46171=CARTESIAN_POINT('Ctrl Pts',(21.5035876969532,-6.1133166792282,19.6959077581311));
#46172=CARTESIAN_POINT('Ctrl Pts',(21.4897410325605,-6.11304106492475,19.9998514866922));
#46173=CARTESIAN_POINT('Ctrl Pts',(23.3852589674394,-6.11280242905631,20.0000853877862));
#46174=CARTESIAN_POINT('Ctrl Pts',(23.3665039203536,-6.11300568882329,20.4118175234676));
#46175=CARTESIAN_POINT('Ctrl Pts',(23.3014450431048,-5.97083721962065,21.8399255703595));
#46176=CARTESIAN_POINT('Ctrl Pts',(23.1900823356932,-4.87086133430093,24.109006595311));
#46177=CARTESIAN_POINT('Ctrl Pts',(23.0511708452045,-2.31206487401468,25.9383146899305));
#46178=CARTESIAN_POINT('Ctrl Pts',(22.9122593547159,0.810030305690605,26.3208445829778));
#46179=CARTESIAN_POINT('Ctrl Pts',(22.7733478642273,3.73477417444681,25.1633988035191));
#46180=CARTESIAN_POINT('Ctrl Pts',(22.6344363737386,5.74959828557432,22.7479710502147));
#46181=CARTESIAN_POINT('Ctrl Pts',(22.49552488325,6.36362201785506,19.6630428036569));
#46182=CARTESIAN_POINT('Ctrl Pts',(22.3566133927613,5.42724801959969,16.6602089478459));
#46183=CARTESIAN_POINT('Ctrl Pts',(22.2177019022727,3.16860928138414,14.4710633427192));
#46184=CARTESIAN_POINT('Ctrl Pts',(22.0787904117841,0.137988073903447,13.628957335745));
#46185=CARTESIAN_POINT('Ctrl Pts',(21.9398789212955,-2.9262517859769,14.3390569846214));
#46186=CARTESIAN_POINT('Ctrl Pts',(21.8009674308068,-5.27755581855221,16.4283575318402));
#46187=CARTESIAN_POINT('Ctrl Pts',(21.6994274461882,-6.05641014667787,18.5916424107086));
#46188=CARTESIAN_POINT('Ctrl Pts',(21.6441912917324,-6.11357292897739,19.8038082207395));
#46189=CARTESIAN_POINT('Ctrl Pts',(21.6352589674394,-6.11337192102228,19.9998483128521));
#46190=CARTESIAN_POINT('Origin',(53.8647410325606,0.,20.));
#46191=CARTESIAN_POINT('',(25.1352589674394,-6.11377511406864,20.0000032316134));
#46192=CARTESIAN_POINT('',(24.9897410325605,-6.11363358775036,19.9998986723535));
#46193=CARTESIAN_POINT('',(53.8647410325606,-6.11325,19.9999999999994));
#46194=CARTESIAN_POINT('Ctrl Pts',(24.9897410325605,-6.11363358775036,19.9998986723535));
#46195=CARTESIAN_POINT('Ctrl Pts',(24.9482129541956,-6.11291938677644,20.9112137264931));
#46196=CARTESIAN_POINT('Ctrl Pts',(24.8603810456679,-5.6761877702843,22.8393071165725));
#46197=CARTESIAN_POINT('Ctrl Pts',(24.7262453069773,-3.72722815930074,25.1688486005525));
#46198=CARTESIAN_POINT('Ctrl Pts',(24.5873338164887,-0.800796749783299,
26.3220210512505));
#46199=CARTESIAN_POINT('Ctrl Pts',(24.448422326,2.32073635810671,25.9349312012086));
#46200=CARTESIAN_POINT('Ctrl Pts',(24.3095108355114,4.87685807407465,24.1018874841042));
#46201=CARTESIAN_POINT('Ctrl Pts',(24.1705993450227,6.24480901733213,21.2694825496889));
#46202=CARTESIAN_POINT('Ctrl Pts',(24.0316878545341,6.09130917345336,18.1277878965458));
#46203=CARTESIAN_POINT('Ctrl Pts',(23.8927763640454,4.45375639682368,15.4422286625293));
#46204=CARTESIAN_POINT('Ctrl Pts',(23.7538648735569,1.73111500389623,13.8670996706124));
#46205=CARTESIAN_POINT('Ctrl Pts',(23.6149533830682,-1.41328568991475,13.7861566510251));
#46206=CARTESIAN_POINT('Ctrl Pts',(23.4760418925796,-4.21336126194841,15.2191201141181));
#46207=CARTESIAN_POINT('Ctrl Pts',(23.3509711090769,-5.81020523120089,17.558038995093));
#46208=CARTESIAN_POINT('Ctrl Pts',(23.2722041557373,-6.11239500844286,19.2875609820401));
#46209=CARTESIAN_POINT('Ctrl Pts',(23.2397410325605,-6.11304143026726,20.0001485574224));
#46210=CARTESIAN_POINT('Ctrl Pts',(25.1352589674394,-6.11377504588096,20.0000032311938));
#46211=CARTESIAN_POINT('Ctrl Pts',(25.1351203791376,-6.11377514153906,20.0030442848715));
#46212=CARTESIAN_POINT('Ctrl Pts',(25.088677960673,-6.11303068323524,21.0221337688692));
#46213=CARTESIAN_POINT('Ctrl Pts',(24.9959317120454,-5.59169558634022,23.0564956744613));
#46214=CARTESIAN_POINT('Ctrl Pts',(24.8570202215568,-3.44853163007304,25.358810962768));
#46215=CARTESIAN_POINT('Ctrl Pts',(24.7181087310682,-0.465186469148229,
26.3555351377534));
#46216=CARTESIAN_POINT('Ctrl Pts',(24.5791972405795,2.63149415450833,25.8038318250175));
#46217=CARTESIAN_POINT('Ctrl Pts',(24.4402857500909,5.08705207263311,23.8381149733452));
#46218=CARTESIAN_POINT('Ctrl Pts',(24.3013742596023,6.30322871286294,20.9373009824156));
#46219=CARTESIAN_POINT('Ctrl Pts',(24.1624627691136,5.98372151391236,17.8081281556077));
#46220=CARTESIAN_POINT('Ctrl Pts',(24.023551278625,4.20637344551665,15.2129708821494));
#46221=CARTESIAN_POINT('Ctrl Pts',(23.8846397881363,1.40420777710976,13.784098950514));
#46222=CARTESIAN_POINT('Ctrl Pts',(23.7457282976477,-1.74007132052403,13.8696348283494));
#46223=CARTESIAN_POINT('Ctrl Pts',(23.6068168071591,-4.46040904974499,15.4487390266817));
#46224=CARTESIAN_POINT('Ctrl Pts',(23.4866603637563,-5.87347405505967,17.7737756783798));
#46225=CARTESIAN_POINT('Ctrl Pts',(23.4128077505164,-6.11250386626396,19.3953031529145));
#46226=CARTESIAN_POINT('Ctrl Pts',(23.3852589674394,-6.11280242905631,20.0000853877862));
#46227=CARTESIAN_POINT('Origin',(53.8647410325606,0.,20.));
#46228=CARTESIAN_POINT('',(26.8852589674394,-6.11281196393338,19.9999098576029));
#46229=CARTESIAN_POINT('',(26.7397410325605,-6.11272776236879,20.0000049172972));
#46230=CARTESIAN_POINT('',(53.8647410325606,-6.11325,19.9999999999994));
#46231=CARTESIAN_POINT('Ctrl Pts',(26.7397410325605,-6.11272776236879,20.0000049172972));
#46232=CARTESIAN_POINT('Ctrl Pts',(26.7168294129797,-6.11274184821953,20.5030044486427));
#46233=CARTESIAN_POINT('Ctrl Pts',(26.6476139632361,-5.92731157177153,22.0225436883079));
#46234=CARTESIAN_POINT('Ctrl Pts',(26.5320946833296,-4.68207687136995,24.3228904424587));
#46235=CARTESIAN_POINT('Ctrl Pts',(26.3931831928409,-2.04397156988813,26.0358434231188));
#46236=CARTESIAN_POINT('Ctrl Pts',(26.2542717023523,1.09211567872115,26.2782568401754));
#46237=CARTESIAN_POINT('Ctrl Pts',(26.1153602118636,3.96212589368178,24.9910704272264));
#46238=CARTESIAN_POINT('Ctrl Pts',(25.976448721375,5.86682563350311,22.4878871744893));
#46239=CARTESIAN_POINT('Ctrl Pts',(25.8375372308864,6.34216437072042,19.3785688278802));
#46240=CARTESIAN_POINT('Ctrl Pts',(25.6986257403977,5.27233320006711,16.4206525407014));
#46241=CARTESIAN_POINT('Ctrl Pts',(25.5597142499091,2.91797988069426,14.3347887044894));
#46242=CARTESIAN_POINT('Ctrl Pts',(25.4208027594205,-0.147293944655354,
13.6291656668231));
#46243=CARTESIAN_POINT('Ctrl Pts',(25.2818912689318,-3.17668188663938,14.4756975283739));
#46244=CARTESIAN_POINT('Ctrl Pts',(25.1429797784432,-5.43212059438828,16.6681399406727));
#46245=CARTESIAN_POINT('Ctrl Pts',(25.0455963663194,-6.08548669297453,18.7742226688102));
#46246=CARTESIAN_POINT('Ctrl Pts',(24.9945167843585,-6.11371572125424,19.8950969410976));
#46247=CARTESIAN_POINT('Ctrl Pts',(24.9897410325605,-6.11363358775036,19.9998986723535));
#46248=CARTESIAN_POINT('Ctrl Pts',(26.8852589674394,-6.11281196393338,19.9999098576029));
#46249=CARTESIAN_POINT('Ctrl Pts',(26.8574330077589,-6.11249297390719,20.6107742611335));
#46250=CARTESIAN_POINT('Ctrl Pts',(26.7833032179154,-5.87007710988381,22.2383961010393));
#46251=CARTESIAN_POINT('Ctrl Pts',(26.6628695979091,-4.44680132145817,24.5645573000867));
#46252=CARTESIAN_POINT('Ctrl Pts',(26.5239581074204,-1.7217612793893,26.135532856655));
#46253=CARTESIAN_POINT('Ctrl Pts',(26.3850466169318,1.42275917377253,26.2116810664862));
#46254=CARTESIAN_POINT('Ctrl Pts',(26.2461351264432,4.22064643785949,24.7744496002033));
#46255=CARTESIAN_POINT('Ctrl Pts',(26.1072236359545,5.99023870889178,22.1739975963169));
#46256=CARTESIAN_POINT('Ctrl Pts',(25.968312145466,6.30040229708003,19.0438848221863));
#46257=CARTESIAN_POINT('Ctrl Pts',(25.8294006549772,5.07557065842261,16.1467146706146));
#46258=CARTESIAN_POINT('Ctrl Pts',(25.6904891644886,2.61415501023178,14.18833768008));
#46259=CARTESIAN_POINT('Ctrl Pts',(25.551577674,-0.484158930120513,13.6458820070224));
#46260=CARTESIAN_POINT('Ctrl Pts',(25.4126661835113,-3.46451506210964,14.6515085563579));
#46261=CARTESIAN_POINT('Ctrl Pts',(25.2738932813245,-5.5986645637313,16.9579086962675));
#46262=CARTESIAN_POINT('Ctrl Pts',(25.1814242093005,-6.11374318114547,18.9869958074943));
#46263=CARTESIAN_POINT('Ctrl Pts',(25.1352589674394,-6.11377504588096,20.0000032311938));
#46264=CARTESIAN_POINT('Origin',(53.8647410325606,0.,20.));
#46265=CARTESIAN_POINT('',(28.6352589674394,-6.11335271655686,20.0001533502409));
#46266=CARTESIAN_POINT('',(28.4897410325605,-6.1136580696871,20.0000927339656));
#46267=CARTESIAN_POINT('',(53.8647410325606,-6.11325,19.9999999999994));
#46268=CARTESIAN_POINT('Ctrl Pts',(28.4897410325605,-6.1136580696871,20.0000927339656));
#46269=CARTESIAN_POINT('Ctrl Pts',(28.4854458717638,-6.11372698856088,20.0943470171741));
#46270=CARTESIAN_POINT('Ctrl Pts',(28.4348468808043,-6.0885798609534,21.2046694997386));
#46271=CARTESIAN_POINT('Ctrl Pts',(28.3379440596818,-5.4492952092373,23.3036960104557));
#46272=CARTESIAN_POINT('Ctrl Pts',(28.1990325691932,-3.2052359128581,25.5077843412612));
#46273=CARTESIAN_POINT('Ctrl Pts',(28.0601210787046,-0.180270636962042,
26.3699865073929));
#46274=CARTESIAN_POINT('Ctrl Pts',(27.9212095882159,2.88861478152641,25.6802403339));
#46275=CARTESIAN_POINT('Ctrl Pts',(27.7822980977273,5.2537340446546,23.6065917699339));
#46276=CARTESIAN_POINT('Ctrl Pts',(27.6433866072386,6.33886255458932,20.6542531015921));
#46277=CARTESIAN_POINT('Ctrl Pts',(27.50447511675,5.87962559290408,17.5425158201557));
#46278=CARTESIAN_POINT('Ctrl Pts',(27.3655636262614,3.98790911718367,15.0295064148517));
#46279=CARTESIAN_POINT('Ctrl Pts',(27.2266521357728,1.12460048411671,13.7274806211505));
#46280=CARTESIAN_POINT('Ctrl Pts',(27.0877406452841,-2.01269960121476,13.953656814058));
#46281=CARTESIAN_POINT('Ctrl Pts',(26.9488291547955,-4.65963666919246,15.6529306748069));
#46282=CARTESIAN_POINT('Ctrl Pts',(26.8328292838876,-5.92199242415093,17.9563437534471));
#46283=CARTESIAN_POINT('Ctrl Pts',(26.7631332431426,-6.11271338105516,19.4864545365197));
#46284=CARTESIAN_POINT('Ctrl Pts',(26.7397410325605,-6.11272776236879,20.0000049172972));
#46285=CARTESIAN_POINT('Ctrl Pts',(28.6352589674394,-6.11335271655686,20.0001533502409));
#46286=CARTESIAN_POINT('Ctrl Pts',(28.6260494665429,-6.1135607294616,20.202278540951));
#46287=CARTESIAN_POINT('Ctrl Pts',(28.5705361354836,-6.05432216663628,21.4205339982837));
#46288=CARTESIAN_POINT('Ctrl Pts',(28.4687189742614,-5.26686911251823,23.587382763227));
#46289=CARTESIAN_POINT('Ctrl Pts',(28.3298074837727,-2.90933792449704,25.6696541498914));
#46290=CARTESIAN_POINT('Ctrl Pts',(28.1908959932841,0.157008291011193,26.3706023055007));
#46291=CARTESIAN_POINT('Ctrl Pts',(28.0519845027954,3.18510187344724,25.5194520918348));
#46292=CARTESIAN_POINT('Ctrl Pts',(27.9130730123068,5.43719482255474,23.3235730471709));
#46293=CARTESIAN_POINT('Ctrl Pts',(27.7741615218181,6.36459964755315,20.3179570170062));
#46294=CARTESIAN_POINT('Ctrl Pts',(27.6352500313296,5.74136855771394,17.2348756948754));
#46295=CARTESIAN_POINT('Ctrl Pts',(27.4963385408409,3.71934213448194,14.8254739903094));
#46296=CARTESIAN_POINT('Ctrl Pts',(27.3574270503523,0.791155730627478,13.6767652306598));
#46297=CARTESIAN_POINT('Ctrl Pts',(27.2185155598636,-2.3297834869271,14.0686144753238));
#46298=CARTESIAN_POINT('Ctrl Pts',(27.079604069375,-4.88310712004916,15.905553737998));
#46299=CARTESIAN_POINT('Ctrl Pts',(26.9685185385669,-5.97358281620434,18.172252857223));
#46300=CARTESIAN_POINT('Ctrl Pts',(26.9037368379217,-6.11302378974126,19.5942644293674));
#46301=CARTESIAN_POINT('Ctrl Pts',(26.8852589674394,-6.11281196393338,19.9999098576029));
#46302=CARTESIAN_POINT('Origin',(53.8647410325606,0.,20.));
#46303=CARTESIAN_POINT('',(30.3852589674394,-6.11333899670695,19.9998456009343));
#46304=CARTESIAN_POINT('',(30.2397410325605,-6.11301242699033,19.9998552897238));
#46305=CARTESIAN_POINT('',(53.8647410325606,-6.11325,19.9999999999994));
#46306=CARTESIAN_POINT('Ctrl Pts',(30.2397410325605,-6.11301242699033,19.9998552897238));
#46307=CARTESIAN_POINT('Ctrl Pts',(30.207758500385,-6.1123965421807,20.7019031242023));
#46308=CARTESIAN_POINT('Ctrl Pts',(30.1294721380467,-5.81667886159044,22.4208707815258));
#46309=CARTESIAN_POINT('Ctrl Pts',(30.0048819455455,-4.23805306663042,24.7590053384444));
#46310=CARTESIAN_POINT('Ctrl Pts',(29.8659704550568,-1.4454327553499,26.2064442120009));
#46311=CARTESIAN_POINT('Ctrl Pts',(29.7270589645682,1.69934481122473,26.1417792877538));
#46312=CARTESIAN_POINT('Ctrl Pts',(29.5881474740796,4.43010339123342,24.5807651707875));
#46313=CARTESIAN_POINT('Ctrl Pts',(29.4492359835909,6.08153604262198,21.9037187211369));
#46314=CARTESIAN_POINT('Ctrl Pts',(29.3103244931023,6.2512968328913,18.762860753997));
#46315=CARTESIAN_POINT('Ctrl Pts',(29.1714130026136,4.89802618046513,15.9234125616644));
#46316=CARTESIAN_POINT('Ctrl Pts',(29.032501512125,2.35142747477107,14.0771616231904));
#46317=CARTESIAN_POINT('Ctrl Pts',(28.8935900216364,-0.76806003704259,13.673918322815));
#46318=CARTESIAN_POINT('Ctrl Pts',(28.7546785311478,-3.70042164241411,14.8119266316608));
#46319=CARTESIAN_POINT('Ctrl Pts',(28.6200622014558,-5.66844000970638,17.1396582888592));
#46320=CARTESIAN_POINT('Ctrl Pts',(28.5317497019267,-6.11298401106189,19.0782420263708));
#46321=CARTESIAN_POINT('Ctrl Pts',(28.4897410325605,-6.1136580696871,20.0000927339656));
#46322=CARTESIAN_POINT('Ctrl Pts',(30.3852589674394,-6.11333899670695,19.9998456009343));
#46323=CARTESIAN_POINT('Ctrl Pts',(30.3483620951642,-6.11250411389834,20.8096436190909));
#46324=CARTESIAN_POINT('Ctrl Pts',(30.265161392726,-5.74750682244695,22.6364299549355));
#46325=CARTESIAN_POINT('Ctrl Pts',(30.135656860125,-3.98032524857262,24.9765687229126));
#46326=CARTESIAN_POINT('Ctrl Pts',(29.9967453696363,-1.11503456969162,26.2742269043038));
#46327=CARTESIAN_POINT('Ctrl Pts',(29.8578338791477,2.02191697488329,26.0432670870131));
#46328=CARTESIAN_POINT('Ctrl Pts',(29.7189223886591,4.6662598320792,24.3399590456387));
#46329=CARTESIAN_POINT('Ctrl Pts',(29.5800108981704,6.17374090938801,21.5792873462565));
#46330=CARTESIAN_POINT('Ctrl Pts',(29.4410994076818,6.17708584096459,18.4338467981542));
#46331=CARTESIAN_POINT('Ctrl Pts',(29.3021879171932,4.6754796861493,15.6699751683504));
#46332=CARTESIAN_POINT('Ctrl Pts',(29.1632764267045,2.03476547711032,13.9610468795116));
#46333=CARTESIAN_POINT('Ctrl Pts',(29.0243649362159,-1.10168775744487,13.7234157837727));
#46334=CARTESIAN_POINT('Ctrl Pts',(28.8854534457272,-3.96973186994514,15.0149770091765));
#46335=CARTESIAN_POINT('Ctrl Pts',(28.7557514561351,-5.74458857655193,17.3549142648056));
#46336=CARTESIAN_POINT('Ctrl Pts',(28.6723532967058,-6.11251487536801,19.1860268887194));
#46337=CARTESIAN_POINT('Ctrl Pts',(28.6352589674394,-6.11335271655686,20.0001533502409));
#46338=CARTESIAN_POINT('Origin',(53.8647410325606,0.,20.));
#46339=CARTESIAN_POINT('',(32.1352589674394,-6.11281908049607,20.0000934609265));
#46340=CARTESIAN_POINT('',(31.9897410325605,-6.1130709765779,20.0001517774591));
#46341=CARTESIAN_POINT('',(53.8647410325606,-6.11325,19.9999999999994));
#46342=CARTESIAN_POINT('Ctrl Pts',(31.9897410325605,-6.1130709765779,20.0001517774591));
#46343=CARTESIAN_POINT('Ctrl Pts',(31.9763749591691,-6.113344967759,20.2935420849967));
#46344=CARTESIAN_POINT('Ctrl Pts',(31.9167050556149,-6.02075144272683,21.6031472979479));
#46345=CARTESIAN_POINT('Ctrl Pts',(31.8107313218978,-5.10103373445315,23.8195131164703));
#46346=CARTESIAN_POINT('Ctrl Pts',(31.6718198314091,-2.65267034660569,25.7941837767848));
#46347=CARTESIAN_POINT('Ctrl Pts',(31.5329083409205,0.441974997287937,26.357191495361));
#46348=CARTESIAN_POINT('Ctrl Pts',(31.3939968504318,3.4289399932875,25.3713681803941));
#46349=CARTESIAN_POINT('Ctrl Pts',(31.2550853599432,5.58049698283711,23.0768943809405));
#46350=CARTESIAN_POINT('Ctrl Pts',(31.1161738694545,6.37245250121533,20.0327830241454));
#46351=CARTESIAN_POINT('Ctrl Pts',(30.977262378966,5.6118588788506,16.9806845923648));
#46352=CARTESIAN_POINT('Ctrl Pts',(30.8383508884773,3.48402294614019,14.6641954948025));
#46353=CARTESIAN_POINT('Ctrl Pts',(30.6994393979887,0.507358900497252,13.6476923442733));
#46354=CARTESIAN_POINT('Ctrl Pts',(30.5605279075,-2.59291526618855,14.1788303555657));
#46355=CARTESIAN_POINT('Ctrl Pts',(30.4216164170114,-5.06146587467247,16.1282059963831));
#46356=CARTESIAN_POINT('Ctrl Pts',(30.3146874586982,-6.01243369276824,18.3548832896175));
#46357=CARTESIAN_POINT('Ctrl Pts',(30.2540623305479,-6.11328821096629,19.685488804174));
#46358=CARTESIAN_POINT('Ctrl Pts',(30.2397410325605,-6.11301242699033,19.9998552897238));
#46359=CARTESIAN_POINT('Ctrl Pts',(32.1352589674394,-6.11281908049607,20.0000934609265));
#46360=CARTESIAN_POINT('Ctrl Pts',(32.1169785539483,-6.11303668109335,20.4014027704384));
#46361=CARTESIAN_POINT('Ctrl Pts',(32.0523943102942,-5.97552686421729,21.819071362413));
#46362=CARTESIAN_POINT('Ctrl Pts',(31.9415062364773,-4.8918043167284,24.0840514033414));
#46363=CARTESIAN_POINT('Ctrl Pts',(31.8025947459886,-2.34239333841841,25.9264170277183));
#46364=CARTESIAN_POINT('Ctrl Pts',(31.6636832554999,0.777705418913837,26.3249031312495));
#46365=CARTESIAN_POINT('Ctrl Pts',(31.5247717650114,3.70832832222358,25.1824247599837));
#46366=CARTESIAN_POINT('Ctrl Pts',(31.3858602745226,5.73547458931472,22.7773290358944));
#46367=CARTESIAN_POINT('Ctrl Pts',(31.2469487840341,6.36526149692924,19.6955802010263));
#46368=CARTESIAN_POINT('Ctrl Pts',(31.1080372935454,5.44425124037868,16.6879985250709));
#46369=CARTESIAN_POINT('Ctrl Pts',(30.9691258030568,3.19683367304369,14.48733460065));
#46370=CARTESIAN_POINT('Ctrl Pts',(30.8302143125682,0.170557201505726,13.629746034944));
#46371=CARTESIAN_POINT('Ctrl Pts',(30.6913028220795,-2.8972728848445,14.3241709707707));
#46372=CARTESIAN_POINT('Ctrl Pts',(30.5523913315909,-5.25922740334937,16.4014235511586));
#46373=CARTESIAN_POINT('Ctrl Pts',(30.4503767133775,-6.0528232864935,18.5707916024673));
#46374=CARTESIAN_POINT('Ctrl Pts',(30.3946659253271,-6.11355185234856,19.7933853948378));
#46375=CARTESIAN_POINT('Ctrl Pts',(30.3852589674394,-6.11333899670695,19.9998456009343));
#46376=CARTESIAN_POINT('Origin',(53.8647410325606,0.,20.));
#46377=CARTESIAN_POINT('',(33.8852589674394,-6.11377473629356,19.9999921625065));
#46378=CARTESIAN_POINT('',(33.7397410325605,-6.11360782021149,19.9998906860949));
#46379=CARTESIAN_POINT('',(53.8647410325606,-6.11325,19.9999999999994));
#46380=CARTESIAN_POINT('Ctrl Pts',(33.7397410325605,-6.11360782021148,19.9998906860949));
#46381=CARTESIAN_POINT('Ctrl Pts',(33.6986875877904,-6.11285986208749,20.9008011180488));
#46382=CARTESIAN_POINT('Ctrl Pts',(33.6113303128573,-5.68377501480363,22.8185295471014));
#46383=CARTESIAN_POINT('Ctrl Pts',(33.4776692077614,-3.75360435860782,25.1497261991253));
#46384=CARTESIAN_POINT('Ctrl Pts',(33.3387577172728,-0.833106600630097,
26.3178444899273));
#46385=CARTESIAN_POINT('Ctrl Pts',(33.1998462267841,2.29036464937583,25.9467180343284));
#46386=CARTESIAN_POINT('Ctrl Pts',(33.0609347362955,4.855824102872,24.1267660327289));
#46387=CARTESIAN_POINT('Ctrl Pts',(32.9220232458069,6.2382373842586,21.301391541603));
#46388=CARTESIAN_POINT('Ctrl Pts',(32.7831117553182,6.10080095490451,18.1589532011506));
#46389=CARTESIAN_POINT('Ctrl Pts',(32.6442002648296,4.47699906757734,15.4650573370957));
#46390=CARTESIAN_POINT('Ctrl Pts',(32.5052887743409,1.76244584798862,13.8760298629218));
#46391=CARTESIAN_POINT('Ctrl Pts',(32.3663772838523,-1.38149994633938,13.779012658333));
#46392=CARTESIAN_POINT('Ctrl Pts',(32.2274657933637,-4.18886472194398,15.197642459357));
#46393=CARTESIAN_POINT('Ctrl Pts',(32.1019203762664,-5.8037503628612,17.5372120805641));
#46394=CARTESIAN_POINT('Ctrl Pts',(32.022678789332,-6.11239578539673,19.2771557033073));
#46395=CARTESIAN_POINT('Ctrl Pts',(31.9897410325605,-6.1130709765779,20.0001517774591));
#46396=CARTESIAN_POINT('Ctrl Pts',(33.8852589674394,-6.11377433895741,19.9999921684411));
#46397=CARTESIAN_POINT('Ctrl Pts',(33.8392911825694,-6.11369836731836,21.0086671186757));
#46398=CARTESIAN_POINT('Ctrl Pts',(33.7470195675366,-5.6020923000678,23.0334651258696));
#46399=CARTESIAN_POINT('Ctrl Pts',(33.6084441223409,-3.47588262343321,25.341110870073));
#46400=CARTESIAN_POINT('Ctrl Pts',(33.4695326318522,-0.497672041157185,
26.3530738920422));
#46401=CARTESIAN_POINT('Ctrl Pts',(33.3306211413636,2.60178860923987,25.8172090706048));
#46402=CARTESIAN_POINT('Ctrl Pts',(33.191709650875,5.0673638491298,23.8640715519811));
#46403=CARTESIAN_POINT('Ctrl Pts',(33.0527981603864,6.29835454118703,20.9695129766052));
#46404=CARTESIAN_POINT('Ctrl Pts',(32.9138866698977,5.99484891033732,17.8387476129511));
#46405=CARTESIAN_POINT('Ctrl Pts',(32.774975179409,4.23079139261945,15.2345378471302));
#46406=CARTESIAN_POINT('Ctrl Pts',(32.6360636889205,1.43596722108643,13.7913589668703));
#46407=CARTESIAN_POINT('Ctrl Pts',(32.4971521984318,-1.70870807523846,13.8608191057836));
#46408=CARTESIAN_POINT('Ctrl Pts',(32.3582407079432,-4.43708317105403,15.4259953791621));
#46409=CARTESIAN_POINT('Ctrl Pts',(32.2376096309457,-5.86764475673546,17.7529331209653));
#46410=CARTESIAN_POINT('Ctrl Pts',(32.1632823841111,-6.11248550422285,19.3848963265668));
#46411=CARTESIAN_POINT('Ctrl Pts',(32.1352589674394,-6.11281908049607,20.0000934609265));
#46412=CARTESIAN_POINT('Origin',(53.8647410325606,0.,20.));
#46413=CARTESIAN_POINT('',(35.6352589674395,-6.11279596489353,19.9999180648868));
#46414=CARTESIAN_POINT('',(35.4897410325605,-6.11272955150596,20.0000146122445));
#46415=CARTESIAN_POINT('',(53.8647410325606,-6.11325,19.9999999999994));
#46416=CARTESIAN_POINT('Ctrl Pts',(35.4897410325605,-6.11272955150596,20.0000146122445));
#46417=CARTESIAN_POINT('Ctrl Pts',(35.4673040465744,-6.11277055632431,20.4925936701237));
#46418=CARTESIAN_POINT('Ctrl Pts',(35.3985632304255,-5.93250613741697,22.0016922885538));
#46419=CARTESIAN_POINT('Ctrl Pts',(35.2835185841137,-4.70411576761554,24.2988975856361));
#46420=CARTESIAN_POINT('Ctrl Pts',(35.144607093625,-2.07480213772069,26.025315070287));
#46421=CARTESIAN_POINT('Ctrl Pts',(35.0056956031364,1.06000482861184,26.2837580610839));
#46422=CARTESIAN_POINT('Ctrl Pts',(34.8667841126477,3.93655807151044,25.0112609347891));
#46423=CARTESIAN_POINT('Ctrl Pts',(34.7278726221591,5.85403004228618,22.5178478649292));
#46424=CARTESIAN_POINT('Ctrl Pts',(34.5889611316705,6.34525845764879,19.4110002440119));
#46425=CARTESIAN_POINT('Ctrl Pts',(34.4500496411818,5.29056313888617,16.4476532713745));
#46426=CARTESIAN_POINT('Ctrl Pts',(34.3111381506932,2.94690422977004,14.3497804407721));
#46427=CARTESIAN_POINT('Ctrl Pts',(34.1722266602045,-0.114722154020674,
13.6284959048672));
#46428=CARTESIAN_POINT('Ctrl Pts',(34.033315169716,-3.14839826566498,14.459529445284));
#46429=CARTESIAN_POINT('Ctrl Pts',(33.8944036792273,-5.41501600831516,16.6404126389379));
#46430=CARTESIAN_POINT('Ctrl Pts',(33.7965456335088,-6.08237743127135,18.7533759642386));
#46431=CARTESIAN_POINT('Ctrl Pts',(33.7449914179532,-6.11370347767532,19.8846719267787));
#46432=CARTESIAN_POINT('Ctrl Pts',(33.7397410325605,-6.11360782021148,19.9998906860949));
#46433=CARTESIAN_POINT('Ctrl Pts',(35.6352589674395,-6.11279596489353,19.9999180648868));
#46434=CARTESIAN_POINT('Ctrl Pts',(35.6079076413536,-6.11251190746788,20.6003673166567));
#46435=CARTESIAN_POINT('Ctrl Pts',(35.5342524851048,-5.87588159442696,22.2175530727367));
#46436=CARTESIAN_POINT('Ctrl Pts',(35.4142934986932,-4.47007877524375,24.5417640935448));
#46437=CARTESIAN_POINT('Ctrl Pts',(35.2753820082045,-1.7531057040892,26.1266504493554));
#46438=CARTESIAN_POINT('Ctrl Pts',(35.1364705177159,1.39098436071829,26.2188735190977));
#46439=CARTESIAN_POINT('Ctrl Pts',(34.9975590272273,4.19618267645299,24.7959645832859));
#46440=CARTESIAN_POINT('Ctrl Pts',(34.8586475367386,5.97904621488101,22.2045933181914));
#46441=CARTESIAN_POINT('Ctrl Pts',(34.7197360462499,6.3052079479044,19.0761071101149));
#46442=CARTESIAN_POINT('Ctrl Pts',(34.5808245557615,5.09520363185058,16.1727130642877));
#46443=CARTESIAN_POINT('Ctrl Pts',(34.4419130652726,2.64383203702432,14.2017780744179));
#46444=CARTESIAN_POINT('Ctrl Pts',(34.3030015747841,-0.451668196904035,
13.6434898585621));
#46445=CARTESIAN_POINT('Ctrl Pts',(34.1640900842954,-3.43712648530661,14.6338666749417));
#46446=CARTESIAN_POINT('Ctrl Pts',(34.0251785938068,-5.58518225554684,16.9316185845593));
#46447=CARTESIAN_POINT('Ctrl Pts',(33.9322348881881,-6.1119620728916,18.9691958825699));
#46448=CARTESIAN_POINT('Ctrl Pts',(33.8855950127323,-6.11377489434444,19.9926182984567));
#46449=CARTESIAN_POINT('Ctrl Pts',(33.8852589674394,-6.11377433895741,19.9999921684411));
#46450=CARTESIAN_POINT('Origin',(53.8647410325606,0.,20.));
#46451=CARTESIAN_POINT('',(37.3852589674394,-6.11338555021776,20.0001503668437));
#46452=CARTESIAN_POINT('',(37.2397410325605,-6.11368048738509,20.0000837791882));
#46453=CARTESIAN_POINT('',(53.8647410325606,-6.11325,19.9999999999994));
#46454=CARTESIAN_POINT('Ctrl Pts',(37.2397410325605,-6.11368048738509,20.0000837791882));
#46455=CARTESIAN_POINT('Ctrl Pts',(37.2359205053585,-6.11373698512472,20.0839216702238));
#46456=CARTESIAN_POINT('Ctrl Pts',(37.1857961479937,-6.09158033549965,21.183823854746));
#46457=CARTESIAN_POINT('Ctrl Pts',(37.0893679604659,-5.46611361180679,23.2757941922132));
#46458=CARTESIAN_POINT('Ctrl Pts',(36.9504564699773,-3.23335168806423,25.4913261119888));
#46459=CARTESIAN_POINT('Ctrl Pts',(36.8115449794887,-0.212833812579934,
26.3689816591933));
#46460=CARTESIAN_POINT('Ctrl Pts',(36.672633489,2.85953771780081,25.6949336824402));
#46461=CARTESIAN_POINT('Ctrl Pts',(36.5337219985114,5.23522726807311,23.6334035089075));
#46462=CARTESIAN_POINT('Ctrl Pts',(36.3948105080228,6.33543495400973,20.6866509669615));
#46463=CARTESIAN_POINT('Ctrl Pts',(36.2558990175341,5.8921122500055,17.572606574893));
#46464=CARTESIAN_POINT('Ctrl Pts',(36.1169875270455,4.01326785177723,15.0499589136242));
#46465=CARTESIAN_POINT('Ctrl Pts',(35.9780760365568,1.15665303412888,13.7333119300896));
#46466=CARTESIAN_POINT('Ctrl Pts',(35.8391645460682,-1.98176234208496,13.9434462252522));
#46467=CARTESIAN_POINT('Ctrl Pts',(35.7002530555796,-4.63735208393372,15.6291658397334));
#46468=CARTESIAN_POINT('Ctrl Pts',(35.583778551077,-5.91668043407849,17.9354935114547));
#46469=CARTESIAN_POINT('Ctrl Pts',(35.5136078767373,-6.11268593354361,19.4760446090339));
#46470=CARTESIAN_POINT('Ctrl Pts',(35.4897410325605,-6.11272955150596,20.0000146122445));
#46471=CARTESIAN_POINT('Ctrl Pts',(37.3852589674394,-6.11338555021775,20.0001503668437));
#46472=CARTESIAN_POINT('Ctrl Pts',(37.3765241001376,-6.11358143049483,20.1918555857849));
#46473=CARTESIAN_POINT('Ctrl Pts',(37.321485402673,-6.05788617552704,21.3996833608107));
#46474=CARTESIAN_POINT('Ctrl Pts',(37.2201428750454,-5.2851402019413,23.5604098618166));
#46475=CARTESIAN_POINT('Ctrl Pts',(37.0812313845568,-2.93828509988496,25.6547065361601));
#46476=CARTESIAN_POINT('Ctrl Pts',(36.9423198940682,0.124437559632812,26.371321733522));
#46477=CARTESIAN_POINT('Ctrl Pts',(36.8034084035795,3.15684293922622,25.5356632841381));
#46478=CARTESIAN_POINT('Ctrl Pts',(36.6644969130909,5.42013253618787,23.3513263983764));
#46479=CARTESIAN_POINT('Ctrl Pts',(36.5255854226022,6.36289097027834,20.3504908538714));
#46480=CARTESIAN_POINT('Ctrl Pts',(36.3866739321137,5.75542978222766,17.2642636530279));
#46481=CARTESIAN_POINT('Ctrl Pts',(36.247762441625,3.74574746168526,14.844556149896));
#46482=CARTESIAN_POINT('Ctrl Pts',(36.1088509511364,0.823471912402398,13.6808925196843));
#46483=CARTESIAN_POINT('Ctrl Pts',(35.9699394606477,-2.29942978666854,14.0567813438779));
#46484=CARTESIAN_POINT('Ctrl Pts',(35.8310279701591,-4.86211110923449,15.8806431448883));
#46485=CARTESIAN_POINT('Ctrl Pts',(35.7194678057564,-5.96886940144111,18.1513987084486));
#46486=CARTESIAN_POINT('Ctrl Pts',(35.6542114715165,-6.11299279628302,19.5838498692729));
#46487=CARTESIAN_POINT('Ctrl Pts',(35.6352589674395,-6.11279596489353,19.9999180648868));
#46488=CARTESIAN_POINT('Origin',(53.8647410325606,0.,20.));
#46489=CARTESIAN_POINT('',(39.1352589674394,-6.11330594686957,19.9998435437343));
#46490=CARTESIAN_POINT('',(38.9897410325605,-6.11298477368481,19.9998596496536));
#46491=CARTESIAN_POINT('',(53.8647410325606,-6.11325,19.9999999999994));
#46492=CARTESIAN_POINT('Ctrl Pts',(38.9897410325605,-6.11298477368481,19.9998596496536));
#46493=CARTESIAN_POINT('Ctrl Pts',(38.9582331339797,-6.1124002527767,20.6914977876344));
#46494=CARTESIAN_POINT('Ctrl Pts',(38.8804214052361,-5.82301090979044,22.4000401985929));
#46495=CARTESIAN_POINT('Ctrl Pts',(38.7563058463296,-4.26232733267651,24.7372767827135));
#46496=CARTESIAN_POINT('Ctrl Pts',(38.6173943558409,-1.47714331403435,26.1989735631571));
#46497=CARTESIAN_POINT('Ctrl Pts',(38.4784828653523,1.66792374532418,26.1503866534309));
#46498=CARTESIAN_POINT('Ctrl Pts',(38.3395713748636,4.40662707311566,24.6033534999391));
#46499=CARTESIAN_POINT('Ctrl Pts',(38.200659884375,6.0717241128045,21.9347847179741));
#46500=CARTESIAN_POINT('Ctrl Pts',(38.0617483938864,6.25753981577645,18.7948356705868));
#46501=CARTESIAN_POINT('Ctrl Pts',(37.9228369033978,4.91880307017454,15.9485062058842));
#46502=CARTESIAN_POINT('Ctrl Pts',(37.7839254129091,2.3816763046193,14.0892603181216));
#46503=CARTESIAN_POINT('Ctrl Pts',(37.6450139224205,-0.735708924935337,
13.6700744092298));
#46504=CARTESIAN_POINT('Ctrl Pts',(37.5061024319318,-3.67385009436911,14.7930766194401));
#46505=CARTESIAN_POINT('Ctrl Pts',(37.3710114686452,-5.660723652261,17.1188882731015));
#46506=CARTESIAN_POINT('Ctrl Pts',(37.2822243355214,-6.11305224670977,19.067827486753));
#46507=CARTESIAN_POINT('Ctrl Pts',(37.2397410325605,-6.11368048738509,20.0000837791882));
#46508=CARTESIAN_POINT('Ctrl Pts',(39.1352589674394,-6.11330594686957,19.9998435437343));
#46509=CARTESIAN_POINT('Ctrl Pts',(39.0988367287589,-6.11248050595374,20.7992369393628));
#46510=CARTESIAN_POINT('Ctrl Pts',(39.0161106599154,-5.75447725529317,22.6156218959943));
#46511=CARTESIAN_POINT('Ctrl Pts',(38.8870807609091,-4.00571514043749,24.9561549160581));
#46512=CARTESIAN_POINT('Ctrl Pts',(38.7481692704204,-1.14709597416125,26.2684444772495));
#46513=CARTESIAN_POINT('Ctrl Pts',(38.6092577799318,1.990995321361,26.0535248383579));
#46514=CARTESIAN_POINT('Ctrl Pts',(38.4703462894431,4.64401151042891,24.3637578334849));
#46515=CARTESIAN_POINT('Ctrl Pts',(38.3314347989546,6.16558637784845,21.6108289653426));
#46516=CARTESIAN_POINT('Ctrl Pts',(38.1925233084659,6.18501182457331,18.4654466225688));
#46517=CARTESIAN_POINT('Ctrl Pts',(38.0536118179773,4.69755514202461,15.6939343913573));
#46518=CARTESIAN_POINT('Ctrl Pts',(37.9147003274886,2.06561206307644,13.9715282083127));
#46519=CARTESIAN_POINT('Ctrl Pts',(37.775788837,-1.06958533326773,13.7178656052934));
#46520=CARTESIAN_POINT('Ctrl Pts',(37.6368773465114,-3.94419486492413,14.9947475382551));
#46521=CARTESIAN_POINT('Ctrl Pts',(37.5067007233245,-5.73752956130376,17.3341100346003));
#46522=CARTESIAN_POINT('Ctrl Pts',(37.4228279303005,-6.11254306245003,19.1756196668516));
#46523=CARTESIAN_POINT('Ctrl Pts',(37.3852589674394,-6.11338555021775,20.0001503668437));
#46524=CARTESIAN_POINT('Origin',(53.8647410325606,0.,20.));
#46525=CARTESIAN_POINT('',(40.8852589674394,-6.11283726768911,20.0001011899177));
#46526=CARTESIAN_POINT('',(40.7397410325605,-6.11310132804271,20.0001544046255));
#46527=CARTESIAN_POINT('',(53.8647410325606,-6.11325,19.9999999999994));
#46528=CARTESIAN_POINT('Ctrl Pts',(40.7397410325605,-6.1131013280427,20.0001544046255));
#46529=CARTESIAN_POINT('Ctrl Pts',(40.7268495927638,-6.11337233064336,20.2831222931156));
#46530=CARTESIAN_POINT('Ctrl Pts',(40.6676543228043,-6.02480017970596,21.5822937801942));
#46531=CARTESIAN_POINT('Ctrl Pts',(40.5621552226819,-5.12049372012104,23.793384988255));
#46532=CARTESIAN_POINT('Ctrl Pts',(40.4232437321932,-2.68225751383601,25.7805467073961));
#46533=CARTESIAN_POINT('Ctrl Pts',(40.2843322417046,0.409469102548303,26.3593679450851));
#46534=CARTESIAN_POINT('Ctrl Pts',(40.145420751216,3.4014349277457,25.388827891038));
#46535=CARTESIAN_POINT('Ctrl Pts',(40.0065092607273,5.56469392878752,23.1053835650098));
#46536=CARTESIAN_POINT('Ctrl Pts',(39.8675977702387,6.37220162748716,20.0653607341416));
#46537=CARTESIAN_POINT('Ctrl Pts',(39.72868627975,5.62722130693377,17.0094137749083));
#46538=CARTESIAN_POINT('Ctrl Pts',(39.5897747892614,3.51125585888291,14.6820767304917));
#46539=CARTESIAN_POINT('Ctrl Pts',(39.4508632987728,0.539827421410421,13.6503691475795));
#46540=CARTESIAN_POINT('Ctrl Pts',(39.3119518082841,-2.56312158825944,14.1656505649116));
#46541=CARTESIAN_POINT('Ctrl Pts',(39.1730403177955,-5.04160580690685,16.1023806631893));
#46542=CARTESIAN_POINT('Ctrl Pts',(39.0656367258876,-6.00821633318123,18.3340291986372));
#46543=CARTESIAN_POINT('Ctrl Pts',(39.0045369641426,-6.11325926140866,19.6750702784136));
#46544=CARTESIAN_POINT('Ctrl Pts',(38.9897410325605,-6.11298477368481,19.9998596496536));
#46545=CARTESIAN_POINT('Ctrl Pts',(40.8852589674394,-6.11283726768911,20.0001011899177));
#46546=CARTESIAN_POINT('Ctrl Pts',(40.8674531875429,-6.11306762891914,20.3909875540726));
#46547=CARTESIAN_POINT('Ctrl Pts',(40.8033435774836,-5.98015945737357,21.7982170396047));
#46548=CARTESIAN_POINT('Ctrl Pts',(40.6929301372614,-4.91261944606622,24.0589894698594));
#46549=CARTESIAN_POINT('Ctrl Pts',(40.5540186467727,-2.37266058160269,25.91436447159));
#46550=CARTESIAN_POINT('Ctrl Pts',(40.4151071562841,0.745360205886424,26.3287963706994));
#46551=CARTESIAN_POINT('Ctrl Pts',(40.2761956657955,3.68178554845507,25.2013152676496));
#46552=CARTESIAN_POINT('Ctrl Pts',(40.1372841753068,5.72120098964531,22.806614432796));
#46553=CARTESIAN_POINT('Ctrl Pts',(39.9983726848182,6.36673461236813,19.728125554767));
#46554=CARTESIAN_POINT('Ctrl Pts',(39.8594611943296,5.46111216921441,16.7158746653705));
#46555=CARTESIAN_POINT('Ctrl Pts',(39.7205497038409,3.22497451167542,14.5037499386089));
#46556=CARTESIAN_POINT('Ctrl Pts',(39.5816382133523,0.203121871393965,13.6307012282624));
#46557=CARTESIAN_POINT('Ctrl Pts',(39.4427267228636,-2.86821826005961,14.3094333014226));
#46558=CARTESIAN_POINT('Ctrl Pts',(39.303815232375,-5.24076153202002,16.3745836235273));
#46559=CARTESIAN_POINT('Ctrl Pts',(39.2013259805669,-6.04918142844035,18.5499403958289));
#46560=CARTESIAN_POINT('Ctrl Pts',(39.1451405589217,-6.11352989438677,19.7829628890735));
#46561=CARTESIAN_POINT('Ctrl Pts',(39.1352589674394,-6.11330594686957,19.9998435437343));
#46562=CARTESIAN_POINT('Origin',(53.8647410325606,0.,20.));
#46563=CARTESIAN_POINT('',(42.6352589674395,-6.11377032462672,19.9999811532723));
#46564=CARTESIAN_POINT('',(42.4897410325605,-6.11358064030395,19.9998832272783));
#46565=CARTESIAN_POINT('',(53.8647410325606,-6.11325,19.9999999999994));
#46566=CARTESIAN_POINT('Ctrl Pts',(42.4897410325605,-6.11358064030395,19.9998832272783));
#46567=CARTESIAN_POINT('Ctrl Pts',(42.4491622213851,-6.1128044966145,20.8903893714117));
#46568=CARTESIAN_POINT('Ctrl Pts',(42.3622795800467,-5.69129834837748,22.7977483927856));
#46569=CARTESIAN_POINT('Ctrl Pts',(42.2290931085455,-3.77988245302682,25.1304692035152));
#46570=CARTESIAN_POINT('Ctrl Pts',(42.0901816180568,-0.865394677250782,
26.3135028042683));
#46571=CARTESIAN_POINT('Ctrl Pts',(41.9512701275682,2.25993307925686,25.9583494429412));
#46572=CARTESIAN_POINT('Ctrl Pts',(41.8123586370795,4.83466321896507,24.151536723444));
#46573=CARTESIAN_POINT('Ctrl Pts',(41.673447146591,6.23150270747516,21.3332665201104));
#46574=CARTESIAN_POINT('Ctrl Pts',(41.5345356561023,6.11013328470932,18.1901666236902));
#46575=CARTESIAN_POINT('Ctrl Pts',(41.3956241656137,4.5001247266669,15.4880045377507));
#46576=CARTESIAN_POINT('Ctrl Pts',(41.256712675125,1.79373062847491,13.8851201124316));
#46577=CARTESIAN_POINT('Ctrl Pts',(41.1178011846364,-1.34967809562946,13.7720312585004));
#46578=CARTESIAN_POINT('Ctrl Pts',(40.9788896941477,-4.16425870100727,15.1762903198884));
#46579=CARTESIAN_POINT('Ctrl Pts',(40.8528696434558,-5.79723424303751,17.5163871102771));
#46580=CARTESIAN_POINT('Ctrl Pts',(40.7731534229267,-6.11239893600378,19.2667504016246));
#46581=CARTESIAN_POINT('Ctrl Pts',(40.7397410325605,-6.1131013280427,20.0001544046255));
#46582=CARTESIAN_POINT('Ctrl Pts',(42.6352589674394,-6.11377032462672,19.9999811532723));
#46583=CARTESIAN_POINT('Ctrl Pts',(42.5897658161642,-6.11359441963512,20.9982430904406));
#46584=CARTESIAN_POINT('Ctrl Pts',(42.497968834726,-5.61028523359083,23.0127267136883));
#46585=CARTESIAN_POINT('Ctrl Pts',(42.3598680231251,-3.5031427704913,25.3232711811303));
#46586=CARTESIAN_POINT('Ctrl Pts',(42.2209565326363,-0.530144605918972,
26.350446601233));
#46587=CARTESIAN_POINT('Ctrl Pts',(42.0820450421478,2.57201506314977,25.8304342765551));
#46588=CARTESIAN_POINT('Ctrl Pts',(41.943133551659,5.04754318408075,23.8899271385383));
#46589=CARTESIAN_POINT('Ctrl Pts',(41.8042220611705,6.2933157545682,21.001699631427));
#46590=CARTESIAN_POINT('Ctrl Pts',(41.6653105706818,6.00581962429792,17.869423557181));
#46591=CARTESIAN_POINT('Ctrl Pts',(41.5263990801932,4.25509876298692,15.256229363099));
#46592=CARTESIAN_POINT('Ctrl Pts',(41.3874875897045,1.46768913436197,13.7987812534008));
#46593=CARTESIAN_POINT('Ctrl Pts',(41.248576099216,-1.67730017084697,13.8521638379692));
#46594=CARTESIAN_POINT('Ctrl Pts',(41.1096646087272,-4.41364132394809,15.4033712786614));
#46595=CARTESIAN_POINT('Ctrl Pts',(40.9885588981351,-5.86175571304379,17.7320917419551));
#46596=CARTESIAN_POINT('Ctrl Pts',(40.9137570177058,-6.11246857584011,19.3744897694183));
#46597=CARTESIAN_POINT('Ctrl Pts',(40.8852589674394,-6.11283726768911,20.0001011899177));
#46598=CARTESIAN_POINT('Origin',(53.8647410325606,0.,20.));
#46599=CARTESIAN_POINT('',(44.3852589674394,-6.11278156388414,19.9999265724237));
#46600=CARTESIAN_POINT('',(44.2397410325605,-6.11273311396858,20.0000242543606));
#46601=CARTESIAN_POINT('',(53.8647410325606,-6.11325,19.9999999999994));
#46602=CARTESIAN_POINT('Ctrl Pts',(44.2397410325605,-6.11273311396858,20.0000242543606));
#46603=CARTESIAN_POINT('Ctrl Pts',(44.2177786801691,-6.11279978336087,20.4821824561146));
#46604=CARTESIAN_POINT('Ctrl Pts',(44.1495124976149,-5.9376425539596,21.9808403899033));
#46605=CARTESIAN_POINT('Ctrl Pts',(44.0349424848978,-4.72603171623352,24.2747923720425));
#46606=CARTESIAN_POINT('Ctrl Pts',(43.8960309944091,-2.10557847814608,26.0146292387217));
#46607=CARTESIAN_POINT('Ctrl Pts',(43.7571195039205,1.02786627402308,26.2890950485458));
#46608=CARTESIAN_POINT('Ctrl Pts',(43.6182080134318,3.91088736273947,25.0313204671222));
#46609=CARTESIAN_POINT('Ctrl Pts',(43.4792965229432,5.84108144907249,22.5477427484381));
#46610=CARTESIAN_POINT('Ctrl Pts',(43.3403850324546,6.34818670374496,19.4434470543486));
#46611=CARTESIAN_POINT('Ctrl Pts',(43.2014735419659,5.30865480258217,16.4747468468295));
#46612=CARTESIAN_POINT('Ctrl Pts',(43.0625620514773,2.9757515580194,14.3649198522237));
#46613=CARTESIAN_POINT('Ctrl Pts',(42.9236505609886,-0.0821473649868688,
13.6279926697042));
#46614=CARTESIAN_POINT('Ctrl Pts',(42.7847390705,-3.12003235757933,14.4435061689429));
#46615=CARTESIAN_POINT('Ctrl Pts',(42.6458275800114,-5.39776989439614,16.6127731439911));
#46616=CARTESIAN_POINT('Ctrl Pts',(42.5474949006982,-6.07921398551127,18.7325287458751));
#46617=CARTESIAN_POINT('Ctrl Pts',(42.4954660515479,-6.11369014172182,19.8742471025154));
#46618=CARTESIAN_POINT('Ctrl Pts',(42.4897410325605,-6.11358064030395,19.9998832272783));
#46619=CARTESIAN_POINT('Ctrl Pts',(44.3852589674395,-6.11278156388414,19.9999265724237));
#46620=CARTESIAN_POINT('Ctrl Pts',(44.3583822749483,-6.11253215560594,20.5899600742025));
#46621=CARTESIAN_POINT('Ctrl Pts',(44.2852017522942,-5.88162653249256,22.1967089582262));
#46622=CARTESIAN_POINT('Ctrl Pts',(44.1657173994773,-4.49323939823524,24.5188521826282));
#46623=CARTESIAN_POINT('Ctrl Pts',(44.0268059089887,-1.78440430929869,26.1176079148025));
#46624=CARTESIAN_POINT('Ctrl Pts',(43.8878944185,1.35917319264309,26.2259034340967));
#46625=CARTESIAN_POINT('Ctrl Pts',(43.7489829280113,4.1716092428508,24.8173542181636));
#46626=CARTESIAN_POINT('Ctrl Pts',(43.6100714375227,5.967697451428,22.2351314204129));
#46627=CARTESIAN_POINT('Ctrl Pts',(43.4711599470341,6.309848804664,19.1083535450766));
#46628=CARTESIAN_POINT('Ctrl Pts',(43.3322484565454,5.11470343610716,16.1988114886301));
#46629=CARTESIAN_POINT('Ctrl Pts',(43.1933369660568,2.67343996414062,14.2153700121414));
#46630=CARTESIAN_POINT('Ctrl Pts',(43.0544254755682,-0.419165658805117,
13.6412638450101));
#46631=CARTESIAN_POINT('Ctrl Pts',(42.9155139850796,-3.40964807513886,14.6163650437647));
#46632=CARTESIAN_POINT('Ctrl Pts',(42.7766024945909,-5.56942266143649,16.9031053365388));
#46633=CARTESIAN_POINT('Ctrl Pts',(42.6831841553776,-6.10935563599417,18.9483542931198));
#46634=CARTESIAN_POINT('Ctrl Pts',(42.6360696463271,-6.11377345921861,19.9821923245347));
#46635=CARTESIAN_POINT('Ctrl Pts',(42.6352589674394,-6.11377032462672,19.9999811532723));
#46636=CARTESIAN_POINT('Origin',(53.8647410325606,0.,20.));
#46637=CARTESIAN_POINT('',(46.1352589674395,-6.11341807123084,20.0001467345291));
#46638=CARTESIAN_POINT('',(45.9897410325605,-6.11370098092917,20.0000743962474));
#46639=CARTESIAN_POINT('',(53.8647410325606,-6.11325,19.9999999999994));
#46640=CARTESIAN_POINT('Ctrl Pts',(45.9897410325605,-6.11370098092917,20.0000743962474));
#46641=CARTESIAN_POINT('Ctrl Pts',(45.9863951389532,-6.11374584420487,20.0734961832118));
#46642=CARTESIAN_POINT('Ctrl Pts',(45.9367454151831,-6.09452688272932,21.1629787472043));
#46643=CARTESIAN_POINT('Ctrl Pts',(45.84079186125,-5.48278915103411,23.2478067572163));
#46644=CARTESIAN_POINT('Ctrl Pts',(45.7018803707614,-3.26138295580096,25.4747243604157));
#46645=CARTESIAN_POINT('Ctrl Pts',(45.5629688802727,-0.245391425534477,
26.3678103501275));
#46646=CARTESIAN_POINT('Ctrl Pts',(45.4240573897841,2.83038591667594,25.7094781871552));
#46647=CARTESIAN_POINT('Ctrl Pts',(45.2851458992955,5.21658366263703,23.6601202845843));
#46648=CARTESIAN_POINT('Ctrl Pts',(45.1462344088069,6.33184176934682,20.719030885896));
#46649=CARTESIAN_POINT('Ctrl Pts',(45.0073229183182,5.90444490978662,17.6027607724275));
#46650=CARTESIAN_POINT('Ctrl Pts',(44.8684114278296,4.03852169487032,15.0705407875732));
#46651=CARTESIAN_POINT('Ctrl Pts',(44.7294999373409,1.18867535364643,13.7393070263308));
#46652=CARTESIAN_POINT('Ctrl Pts',(44.5905884468523,-1.95077328725316,13.9333939316404));
#46653=CARTESIAN_POINT('Ctrl Pts',(44.4516769563636,-4.61494629599519,15.6055152415786));
#46654=CARTESIAN_POINT('Ctrl Pts',(44.3347278182664,-5.91130989900841,17.9146439238443));
#46655=CARTESIAN_POINT('Ctrl Pts',(44.264082510332,-6.11265922245179,19.4656350896121));
#46656=CARTESIAN_POINT('Ctrl Pts',(44.2397410325605,-6.11273311396858,20.0000242543606));
#46657=CARTESIAN_POINT('Ctrl Pts',(46.1352589674395,-6.11341807123084,20.0001467345292));
#46658=CARTESIAN_POINT('Ctrl Pts',(46.1269987337324,-6.11360120807088,20.1814323295707));
#46659=CARTESIAN_POINT('Ctrl Pts',(46.0724346698624,-6.06139532481641,21.3788331453416));
#46660=CARTESIAN_POINT('Ctrl Pts',(45.9715667758295,-5.30327315797554,23.5333439048828));
#46661=CARTESIAN_POINT('Ctrl Pts',(45.832655285341,-2.96715547971806,25.6396111299885));
#46662=CARTESIAN_POINT('Ctrl Pts',(45.6937437948522,0.0918635759318163,
26.371874639516));
#46663=CARTESIAN_POINT('Ctrl Pts',(45.5548323043637,3.12850149718234,25.5517297953366));
#46664=CARTESIAN_POINT('Ctrl Pts',(45.4159208138749,5.40292858824861,23.3789921587039));
#46665=CARTESIAN_POINT('Ctrl Pts',(45.2770093233864,6.36101599132474,20.3830155302438));
#46666=CARTESIAN_POINT('Ctrl Pts',(45.1380978328977,5.76934058177901,17.2937231128846));
#46667=CARTESIAN_POINT('Ctrl Pts',(44.9991863424091,3.77205488934985,14.8637730531032));
#46668=CARTESIAN_POINT('Ctrl Pts',(44.8602748519205,0.855766571765285,13.6851849660543));
#46669=CARTESIAN_POINT('Ctrl Pts',(44.7213633614318,-2.26901598809372,14.0451035454785));
#46670=CARTESIAN_POINT('Ctrl Pts',(44.5824518709432,-4.84098802139722,15.8558402160407));
#46671=CARTESIAN_POINT('Ctrl Pts',(44.4704170729457,-5.96409876329752,18.130544729991));
#46672=CARTESIAN_POINT('Ctrl Pts',(44.4046861051111,-6.1129618423525,19.5734357728683));
#46673=CARTESIAN_POINT('Ctrl Pts',(44.3852589674395,-6.11278156388414,19.9999265724237));
#46674=CARTESIAN_POINT('Origin',(53.8647410325606,0.,20.));
#46675=CARTESIAN_POINT('',(47.8852589674394,-6.1132728958666,19.9998421342197));
#46676=CARTESIAN_POINT('',(47.7397410325605,-6.1129581875993,19.99986454581));
#46677=CARTESIAN_POINT('',(53.8647410325606,-6.11325,19.9999999999994));
#46678=CARTESIAN_POINT('Ctrl Pts',(47.7397410325605,-6.1129581875993,19.99986454581));
#46679=CARTESIAN_POINT('Ctrl Pts',(47.7087077675744,-6.11240605145268,20.6810923733887));
#46680=CARTESIAN_POINT('Ctrl Pts',(47.6313706724255,-5.82928215365088,22.3792079115881));
#46681=CARTESIAN_POINT('Ctrl Pts',(47.5077297471136,-4.28649019781716,24.71542441243));
#46682=CARTESIAN_POINT('Ctrl Pts',(47.3688182566251,-1.50881526580176,26.1913408969229));
#46683=CARTESIAN_POINT('Ctrl Pts',(47.2299067661364,1.63645908624929,26.1588332714235));
#46684=CARTESIAN_POINT('Ctrl Pts',(47.0909952756477,4.38303558259688,24.6258215150332));
#46685=CARTESIAN_POINT('Ctrl Pts',(46.9520837851591,6.06175349129441,21.9658001469101));
#46686=CARTESIAN_POINT('Ctrl Pts',(46.8131722946704,6.26361925046179,18.8268420855787));
#46687=CARTESIAN_POINT('Ctrl Pts',(46.6742608041818,4.93945140114888,15.9737057406808));
#46688=CARTESIAN_POINT('Ctrl Pts',(46.5353493136932,2.41186288654182,14.1015134972249));
#46689=CARTESIAN_POINT('Ctrl Pts',(46.3964378232046,-0.703338584205735,
13.6663959357331));
#46690=CARTESIAN_POINT('Ctrl Pts',(46.257526332716,-3.64718252590797,14.7743626963189));
#46691=CARTESIAN_POINT('Ctrl Pts',(46.1219607358346,-5.65294289701776,17.0981221826294));
#46692=CARTESIAN_POINT('Ctrl Pts',(46.0326989691161,-6.11312498121801,19.0574118861948));
#46693=CARTESIAN_POINT('Ctrl Pts',(45.9897410325605,-6.11370098092917,20.0000743962474));
#46694=CARTESIAN_POINT('Ctrl Pts',(47.8852589674394,-6.1132728958666,19.9998421342197));
#46695=CARTESIAN_POINT('Ctrl Pts',(47.8493113623536,-6.11246000348838,20.7888305772424));
#46696=CARTESIAN_POINT('Ctrl Pts',(47.7670599271048,-5.76138532239845,22.5948112591935));
#46697=CARTESIAN_POINT('Ctrl Pts',(47.6385046616932,-4.03100033593876,24.9356115677216));
#46698=CARTESIAN_POINT('Ctrl Pts',(47.4995931712046,-1.17912739907028,26.2624982202955));
#46699=CARTESIAN_POINT('Ctrl Pts',(47.3606816807159,1.96002163140553,26.0636243719931));
#46700=CARTESIAN_POINT('Ctrl Pts',(47.2217701902273,4.62164181175045,24.387442570214));
#46701=CARTESIAN_POINT('Ctrl Pts',(47.0828586997386,6.15727070156947,21.6423284830756));
#46702=CARTESIAN_POINT('Ctrl Pts',(46.94394720925,6.19277615550858,18.4970865545706));
#46703=CARTESIAN_POINT('Ctrl Pts',(46.8050357187613,4.71950782178093,15.7180061583685));
#46704=CARTESIAN_POINT('Ctrl Pts',(46.6661242282728,2.09640466180927,13.9821670984087));
#46705=CARTESIAN_POINT('Ctrl Pts',(46.527212737784,-1.03745495420322,13.7124796177954));
#46706=CARTESIAN_POINT('Ctrl Pts',(46.3883012472955,-3.91855477371191,14.9746488855395));
#46707=CARTESIAN_POINT('Ctrl Pts',(46.2576499905139,-5.73040780021207,17.3133086251774));
#46708=CARTESIAN_POINT('Ctrl Pts',(46.1733025638953,-6.11257461034511,19.1652120019819));
#46709=CARTESIAN_POINT('Ctrl Pts',(46.1352589674395,-6.11341807123084,20.0001467345292));
#46710=CARTESIAN_POINT('Origin',(53.8647410325606,0.,20.));
#46711=CARTESIAN_POINT('',(49.6352589674395,-6.11286344962028,20.0001278181581));
#46712=CARTESIAN_POINT('',(49.4897410325605,-6.11313234159337,20.00015660207));
#46713=CARTESIAN_POINT('',(53.8647410325606,-6.11325,19.9999999999994));
#46714=CARTESIAN_POINT('',(50.,-1.57888188187521,14.0941590297752));
#46715=CARTESIAN_POINT('Ctrl Pts',(50.,-1.57888188187519,14.0941590297752));
#46716=CARTESIAN_POINT('Ctrl Pts',(49.9536961698371,-2.56072134667313,14.356646379112));
#46717=CARTESIAN_POINT('Ctrl Pts',(49.8610885095113,-4.38996617743935,15.3805039208954));
#46718=CARTESIAN_POINT('Ctrl Pts',(49.7395081653245,-5.85584351099758,17.7113562466293));
#46719=CARTESIAN_POINT('Ctrl Pts',(49.6642316513006,-6.11246881893309,19.3641290267299));
#46720=CARTESIAN_POINT('Ctrl Pts',(49.6352589674395,-6.11286344962028,20.0001278181581));
#46721=CARTESIAN_POINT('',(50.,1.57906037163134,14.0937031294847));
#46722=CARTESIAN_POINT('Origin',(50.,0.,20.));
#46723=CARTESIAN_POINT('Ctrl Pts',(50.,1.57906037163134,14.0937031294847));
#46724=CARTESIAN_POINT('Ctrl Pts',(49.9564083618068,0.654826993355806,13.8471232379456));
#46725=CARTESIAN_POINT('Ctrl Pts',(49.8665128934508,-1.37290819747911,13.7923707941805));
#46726=CARTESIAN_POINT('Ctrl Pts',(49.7303135949318,-4.13954687382562,15.1550528216166));
#46727=CARTESIAN_POINT('Ctrl Pts',(49.6038189106453,-5.79065559120778,17.495568430254));
#46728=CARTESIAN_POINT('Ctrl Pts',(49.5236280565214,-6.1124042328096,19.2563462638635));
#46729=CARTESIAN_POINT('Ctrl Pts',(49.4897410325605,-6.11313234159337,20.00015660207));
#46730=CARTESIAN_POINT('Origin',(53.8647410325606,0.,20.));
#46731=CARTESIAN_POINT('Ctrl Pts',(49.4897410325605,-6.11313234159337,20.00015660207));
#46732=CARTESIAN_POINT('Ctrl Pts',(49.4773242263585,-6.11339913355694,20.2727018934829));
#46733=CARTESIAN_POINT('Ctrl Pts',(49.4186035899936,-6.02879365594887,21.5614386427174));
#46734=CARTESIAN_POINT('Ctrl Pts',(49.313579123466,-5.13981947893865,23.7671592113954));
#46735=CARTESIAN_POINT('Ctrl Pts',(49.1746676329772,-2.71177477849166,25.7667577971016));
#46736=CARTESIAN_POINT('Ctrl Pts',(49.0357561424887,0.376952608096762,26.3613785707909));
#46737=CARTESIAN_POINT('Ctrl Pts',(48.896844652,3.37384090977041,25.4061465625371));
#46738=CARTESIAN_POINT('Ctrl Pts',(48.7579331615114,5.54874546123675,23.1337916855913));
#46739=CARTESIAN_POINT('Ctrl Pts',(48.6190216710227,6.37178419535544,20.0979366854017));
#46740=CARTESIAN_POINT('Ctrl Pts',(48.4801101805342,5.64243666772738,17.0382211455748));
#46741=CARTESIAN_POINT('Ctrl Pts',(48.3411986900455,3.53839699735355,14.7000969433883));
#46742=CARTESIAN_POINT('Ctrl Pts',(48.2022871995569,0.572281835046422,13.653211912598));
#46743=CARTESIAN_POINT('Ctrl Pts',(48.0633757090682,-2.53326092100598,14.1526232585264));
#46744=CARTESIAN_POINT('Ctrl Pts',(47.9244642185796,-5.02161397036119,16.0766572005871));
#46745=CARTESIAN_POINT('Ctrl Pts',(47.816585993077,-6.00394277771977,18.3131749736855));
#46746=CARTESIAN_POINT('Ctrl Pts',(47.7550115977373,-6.11322987770401,19.664652187524));
#46747=CARTESIAN_POINT('Ctrl Pts',(47.7397410325605,-6.1129581875993,19.99986454581));
#46748=CARTESIAN_POINT('Ctrl Pts',(49.6352589674395,-6.11286344962028,20.0001278181581));
#46749=CARTESIAN_POINT('Ctrl Pts',(49.6179278211377,-6.11309951343155,20.3805754202803));
#46750=CARTESIAN_POINT('Ctrl Pts',(49.554292844673,-5.9847147188434,21.7773037579676));
#46751=CARTESIAN_POINT('Ctrl Pts',(49.4443540380453,-4.93332128443375,24.0338649607667));
#46752=CARTESIAN_POINT('Ctrl Pts',(49.3054425475569,-2.40285814042326,25.9021352451997));
#46753=CARTESIAN_POINT('Ctrl Pts',(49.1665310570681,0.712991615200806,26.332535419579));
#46754=CARTESIAN_POINT('Ctrl Pts',(49.0276195665795,3.65514852614605,25.2200641339167));
#46755=CARTESIAN_POINT('Ctrl Pts',(48.8887080760909,5.70677685429529,22.8358293701168));
#46756=CARTESIAN_POINT('Ctrl Pts',(48.7497965856023,6.36804183630338,19.7606765440198));
#46757=CARTESIAN_POINT('Ctrl Pts',(48.6108850951136,5.47783010606213,16.7438373869472));
#46758=CARTESIAN_POINT('Ctrl Pts',(48.471973604625,3.25303119352331,14.5203085482529));
#46759=CARTESIAN_POINT('Ctrl Pts',(48.3330621141364,0.235681165538501,13.6318230833962));
#46760=CARTESIAN_POINT('Ctrl Pts',(48.1941506236477,-2.83908863701214,14.2948442639057));
#46761=CARTESIAN_POINT('Ctrl Pts',(48.0552391331592,-5.22215870445453,16.3478385001443));
#46762=CARTESIAN_POINT('Ctrl Pts',(47.9522752477563,-6.04548447131879,18.5290888028145));
#46763=CARTESIAN_POINT('Ctrl Pts',(47.8956151925164,-6.11350708383023,19.7725407081699));
#46764=CARTESIAN_POINT('Ctrl Pts',(47.8852589674394,-6.1132728958666,19.9998421342197));
#46765=CARTESIAN_POINT('Ctrl Pts',(50.,3.87994761181434,23.3663343702128));
#46766=CARTESIAN_POINT('Ctrl Pts',(49.9536961698371,4.43959694085051,22.7212974134384));
#46767=CARTESIAN_POINT('Ctrl Pts',(49.8610885095113,5.23040625982842,21.1473591665083));
#46768=CARTESIAN_POINT('Ctrl Pts',(49.7221770190228,5.14179909425296,18.5053810374451));
#46769=CARTESIAN_POINT('Ctrl Pts',(49.583265528534,3.80064971386127,16.2281825446883));
#46770=CARTESIAN_POINT('Ctrl Pts',(49.4443540380455,1.5334472851601,14.869615687937));
#46771=CARTESIAN_POINT('Ctrl Pts',(49.3054425475568,-1.10731381638287,14.7611453275656));
#46772=CARTESIAN_POINT('Ctrl Pts',(49.1665310570682,-3.47831634631721,15.9289604680716));
#46773=CARTESIAN_POINT('Ctrl Pts',(49.0276195665795,-5.00187030240194,18.0886618719085));
#46774=CARTESIAN_POINT('Ctrl Pts',(48.8887080760909,-5.30680167200989,20.7140104959872));
#46775=CARTESIAN_POINT('Ctrl Pts',(48.7497965856023,-4.31881040501176,23.1654120278307));
#46776=CARTESIAN_POINT('Ctrl Pts',(48.6108850951136,-2.27860942925891,24.8456047297691));
#46777=CARTESIAN_POINT('Ctrl Pts',(48.471973604625,0.316740082548733,25.345243753079));
#46778=CARTESIAN_POINT('Ctrl Pts',(48.3330621141364,2.83492042583946,24.5425957314215));
#46779=CARTESIAN_POINT('Ctrl Pts',(48.1941506236477,4.66241659477494,22.6332154649264));
#46780=CARTESIAN_POINT('Ctrl Pts',(48.0552391331591,5.35398723518456,20.0822927687788));
#46781=CARTESIAN_POINT('Ctrl Pts',(47.9163276426705,4.74114203622437,17.5113208963368));
#46782=CARTESIAN_POINT('Ctrl Pts',(47.7774161521818,2.97319114646969,15.5466769678894));
#46783=CARTESIAN_POINT('Ctrl Pts',(47.6385046616932,0.480868395072131,14.6670161194189));
#46784=CARTESIAN_POINT('Ctrl Pts',(47.4995931712046,-2.12861048312721,15.0866539930864));
#46785=CARTESIAN_POINT('Ctrl Pts',(47.3606816807159,-4.21948645356445,16.7033523698713));
#46786=CARTESIAN_POINT('Ctrl Pts',(47.2217701902273,-5.28235004472098,19.1232277661683));
#46787=CARTESIAN_POINT('Ctrl Pts',(47.0828586997386,-5.05825103762128,21.7567151113327));
#46788=CARTESIAN_POINT('Ctrl Pts',(46.94394720925,-3.60178767818055,23.9622060852329));
#46789=CARTESIAN_POINT('Ctrl Pts',(46.8050357187614,-1.2678046565423,25.2023670473592));
#46790=CARTESIAN_POINT('Ctrl Pts',(46.6661242282727,1.37505929109574,25.1750520274788));
#46791=CARTESIAN_POINT('Ctrl Pts',(46.5272127377841,3.68291138574482,23.8869159068166));
#46792=CARTESIAN_POINT('Ctrl Pts',(46.3883012472954,5.09347928620727,21.6517930568259));
#46793=CARTESIAN_POINT('Ctrl Pts',(46.2493897568068,5.26310001796256,19.0142364671977));
#46794=CARTESIAN_POINT('Ctrl Pts',(46.1104782663182,4.15044812249646,16.6168458616026));
#46795=CARTESIAN_POINT('Ctrl Pts',(45.9715667758295,2.0266039639216,15.0437082496005));
#46796=CARTESIAN_POINT('Ctrl Pts',(45.8326552853409,-0.590990794163301,
14.6780941925943));
#46797=CARTESIAN_POINT('Ctrl Pts',(45.6937437948523,-3.06459981842027,15.609079880639));
#46798=CARTESIAN_POINT('Ctrl Pts',(45.5548323043636,-4.79156666466196,17.6098451013006));
#46799=CARTESIAN_POINT('Ctrl Pts',(45.415920813875,-5.35114266623027,20.1929344638081));
#46800=CARTESIAN_POINT('Ctrl Pts',(45.2770093233863,-4.60699581590389,22.7290183388755));
#46801=CARTESIAN_POINT('Ctrl Pts',(45.1380978328978,-2.74042594335429,24.6002192546297));
#46802=CARTESIAN_POINT('Ctrl Pts',(44.999186342409,-0.206193825725144,25.3506481521314));
#46803=CARTESIAN_POINT('Ctrl Pts',(44.8602748519205,2.37827421706705,24.797474678423));
#46804=CARTESIAN_POINT('Ctrl Pts',(44.7213633614318,4.3833126616858,23.0754709641907));
#46805=CARTESIAN_POINT('Ctrl Pts',(44.5824518709432,5.32042501266795,20.6041764860142));
#46806=CARTESIAN_POINT('Ctrl Pts',(44.4435403804546,4.9612983912561,17.9856837848553));
#46807=CARTESIAN_POINT('Ctrl Pts',(44.3046288899659,3.39342842450826,15.8579479639417));
#46808=CARTESIAN_POINT('Ctrl Pts',(44.1657173994772,0.998802293844237,14.7393588300012));
#46809=CARTESIAN_POINT('Ctrl Pts',(44.0268059089887,-1.63916651262383,14.902443263134));
#46810=CARTESIAN_POINT('Ctrl Pts',(43.8878944185,-3.87777784091168,16.3074682725521));
#46811=CARTESIAN_POINT('Ctrl Pts',(43.7489829280114,-5.17162878789402,18.6121213230614));
#46812=CARTESIAN_POINT('Ctrl Pts',(43.6100714375227,-5.20549265308095,21.254909470996));
#46813=CARTESIAN_POINT('Ctrl Pts',(43.4711599470341,-3.9711190313438,23.5919584046275));
#46814=CARTESIAN_POINT('Ctrl Pts',(43.3322484565454,-1.7692438960646,25.053882426206));
#46815=CARTESIAN_POINT('Ctrl Pts',(43.1933369660568,0.863680052850456,25.2845064393927));
#46816=CARTESIAN_POINT('Ctrl Pts',(43.0544254755682,3.28618176265521,24.2276424830475));
#46817=CARTESIAN_POINT('Ctrl Pts',(42.9155139850795,4.90805629305576,22.1407790558278));
#46818=CARTESIAN_POINT('Ctrl Pts',(42.7766024945909,5.3341590889399,19.5323480401464));
#46819=CARTESIAN_POINT('Ctrl Pts',(42.6376910041023,4.46067681792238,17.0378531657386));
#46820=CARTESIAN_POINT('Ctrl Pts',(42.4987795136136,2.500419877423,15.2650393899988));
#46821=CARTESIAN_POINT('Ctrl Pts',(42.359868023125,-0.0690255554895172,
14.6458252723352));
#46822=CARTESIAN_POINT('Ctrl Pts',(42.2209565326364,-2.6216539831997,15.3310727212722));
#46823=CARTESIAN_POINT('Ctrl Pts',(42.0820450421477,-4.53555711038145,17.1538318320691));
#46824=CARTESIAN_POINT('Ctrl Pts',(41.9431335516591,-5.34444214709172,19.6700156396664));
#46825=CARTESIAN_POINT('Ctrl Pts',(41.8042220611705,-4.85123680939198,22.2665950147469));
#46826=CARTESIAN_POINT('Ctrl Pts',(41.6653105706818,-3.17610292243659,24.3109536958502));
#46827=CARTESIAN_POINT('Ctrl Pts',(41.5263990801932,-0.727160856887576,
25.30501542221));
#46828=CARTESIAN_POINT('Ctrl Pts',(41.3874875897045,1.89894266468289,25.0065924837081));
#46829=CARTESIAN_POINT('Ctrl Pts',(41.2485760992159,4.06239828078662,23.4883909972847));
#46830=CARTESIAN_POINT('Ctrl Pts',(41.1096646087273,5.236113611029,21.120297190067));
#46831=CARTESIAN_POINT('Ctrl Pts',(40.9707531182386,5.13413113323201,18.4792603613856));
#46832=CARTESIAN_POINT('Ctrl Pts',(40.83184162775,3.78129729517135,16.2087281412163));
#46833=CARTESIAN_POINT('Ctrl Pts',(40.6929301372613,1.50720906323453,14.8618804625253));
#46834=CARTESIAN_POINT('Ctrl Pts',(40.5540186467727,-1.13408726254032,14.766855856885));
#46835=CARTESIAN_POINT('Ctrl Pts',(40.4151071562841,-3.49908082973853,15.9468055945179));
#46836=CARTESIAN_POINT('Ctrl Pts',(40.2761956657955,-5.01157766438919,18.1142532366539));
#46837=CARTESIAN_POINT('Ctrl Pts',(40.1372841753068,-5.30308138922381,20.7411338077184));
#46838=CARTESIAN_POINT('Ctrl Pts',(39.9983726848182,-4.30257164631444,23.1874486301752));
#46839=CARTESIAN_POINT('Ctrl Pts',(39.8594611943296,-2.25380710492735,24.8571910684525));
#46840=CARTESIAN_POINT('Ctrl Pts',(39.7205497038409,0.344062554699214,25.343554294674));
#46841=CARTESIAN_POINT('Ctrl Pts',(39.5816382133522,2.8581067133027,24.5280434579462));
#46842=CARTESIAN_POINT('Ctrl Pts',(39.4427267228637,4.67581753383213,22.6093451155382));
#46843=CARTESIAN_POINT('Ctrl Pts',(39.303815232375,5.35433798879396,20.0549203371532));
#46844=CARTESIAN_POINT('Ctrl Pts',(39.1649037418864,4.72835710111512,17.4871150710768));
#46845=CARTESIAN_POINT('Ctrl Pts',(39.0259922513977,2.95038539780261,15.531535213733));
#46846=CARTESIAN_POINT('Ctrl Pts',(38.8870807609091,0.453598087257998,14.6646274434759));
#46847=CARTESIAN_POINT('Ctrl Pts',(38.7481692704204,-2.15370135664199,15.0976003826622));
#46848=CARTESIAN_POINT('Ctrl Pts',(38.6092577799318,-4.2362848940627,16.7249668951274));
#46849=CARTESIAN_POINT('Ctrl Pts',(38.4703462894432,-5.28676337130995,19.150244389574));
#46850=CARTESIAN_POINT('Ctrl Pts',(38.3314347989546,-5.04920401259486,21.7825516488649));
#46851=CARTESIAN_POINT('Ctrl Pts',(38.1925233084659,-3.58148446834762,23.9805678671089));
#46852=CARTESIAN_POINT('Ctrl Pts',(38.0536118179773,-1.24119182404874,25.2087805096385));
#46853=CARTESIAN_POINT('Ctrl Pts',(37.9147003274886,1.4014979427954,25.1679546300268));
#46854=CARTESIAN_POINT('Ctrl Pts',(37.775788837,3.70273448948216,23.8680368201549));
#46855=CARTESIAN_POINT('Ctrl Pts',(37.6368773465113,5.10185725047209,21.625731877488));
#46856=CARTESIAN_POINT('Ctrl Pts',(37.4979658560227,5.25799168178786,18.9873425969634));
#46857=CARTESIAN_POINT('Ctrl Pts',(37.3590543655341,4.13309805270831,16.5956715745431));
#46858=CARTESIAN_POINT('Ctrl Pts',(37.2201428750455,2.00123923571802,15.0334123320837));
#46859=CARTESIAN_POINT('Ctrl Pts',(37.0812313845568,-0.618190458456889,
14.6811850851202));
#46860=CARTESIAN_POINT('Ctrl Pts',(36.9423198940682,-3.0870076427842,15.624804535216));
#46861=CARTESIAN_POINT('Ctrl Pts',(36.8034084035795,-4.80372333049662,17.6343724499157));
#46862=CARTESIAN_POINT('Ctrl Pts',(36.6644969130909,-5.35008639059716,20.2202887986762));
#46863=CARTESIAN_POINT('Ctrl Pts',(36.5255854226023,-4.59298394396574,22.7525352008917));
#46864=CARTESIAN_POINT('Ctrl Pts',(36.3866739321136,-2.71687225022107,24.6141691253848));
#46865=CARTESIAN_POINT('Ctrl Pts',(36.247762441625,-0.178836803135813,25.3516323621414));
#46866=CARTESIAN_POINT('Ctrl Pts',(36.1088509511364,2.40276945518559,24.7852534401954));
#46867=CARTESIAN_POINT('Ctrl Pts',(35.9699394606477,4.39897823077324,23.0530217927257));
#46868=CARTESIAN_POINT('Ctrl Pts',(35.8310279701591,5.32344423997211,20.5769687734903));
#46869=CARTESIAN_POINT('Ctrl Pts',(35.6921164796704,4.95093568890783,17.9603462681195));
#46870=CARTESIAN_POINT('Ctrl Pts',(35.5532049891818,3.37220850408812,15.8406537356658));
#46871=CARTESIAN_POINT('Ctrl Pts',(35.4142934986931,0.971895059593761,14.7343213604691));
#46872=CARTESIAN_POINT('Ctrl Pts',(35.2753820082046,-1.66520553072505,14.9108898536072));
#46873=CARTESIAN_POINT('Ctrl Pts',(35.1364705177159,-3.8966046402726,16.3273410423671));
#46874=CARTESIAN_POINT('Ctrl Pts',(34.9975590272272,-5.17865651107395,18.6385785803116));
#46875=CARTESIAN_POINT('Ctrl Pts',(34.8586475367386,-5.19900910440918,21.2815053156134));
#46876=CARTESIAN_POINT('Ctrl Pts',(34.71973604625,-3.95270382681866,23.6122131718835));
#46877=CARTESIAN_POINT('Ctrl Pts',(34.5808245557613,-1.74338361443369,25.0628613564465));
#46878=CARTESIAN_POINT('Ctrl Pts',(34.4419130652727,0.890684955362837,25.2800219556329));
#46879=CARTESIAN_POINT('Ctrl Pts',(34.3030015747841,3.30775196071341,24.2107871601485));
#46880=CARTESIAN_POINT('Ctrl Pts',(34.1640900842955,4.91893654270863,22.1156594315912));
#46881=CARTESIAN_POINT('Ctrl Pts',(34.0251785938068,5.33169858623931,19.5050841211186));
#46882=CARTESIAN_POINT('Ctrl Pts',(33.8862671033182,4.44547502616015,17.0150873826088));
#46883=CARTESIAN_POINT('Ctrl Pts',(33.7473556128296,2.47618047720463,15.2523182724633));
#46884=CARTESIAN_POINT('Ctrl Pts',(33.6084441223409,-0.0963970105370617,
14.6462481232285));
#46885=CARTESIAN_POINT('Ctrl Pts',(33.4695326318523,-2.64548886290509,15.3445365195375));
#46886=CARTESIAN_POINT('Ctrl Pts',(33.3306211413636,-4.55004841626188,17.1770563322397));
#46887=CARTESIAN_POINT('Ctrl Pts',(33.191709650875,-5.34605929739887,19.6973425527592));
#46888=CARTESIAN_POINT('Ctrl Pts',(33.0527981603863,-4.83958581055438,22.2913665625464));
#46889=CARTESIAN_POINT('Ctrl Pts',(32.9138866698977,-3.15402235947797,24.3271346752312));
#46890=CARTESIAN_POINT('Ctrl Pts',(32.7749751794091,-0.700030316245315,
25.3086635887022));
#46891=CARTESIAN_POINT('Ctrl Pts',(32.6360636889204,1.9245132478929,24.9968190181714));
#46892=CARTESIAN_POINT('Ctrl Pts',(32.4971521984318,4.08017903086373,23.4675770528966));
#46893=CARTESIAN_POINT('Ctrl Pts',(32.3582407079432,5.24177252420404,21.0935137613101));
#46894=CARTESIAN_POINT('Ctrl Pts',(32.2193292174545,5.12628950314575,18.4530328149528));
#46895=CARTESIAN_POINT('Ctrl Pts',(32.0804177269659,3.76186561327901,16.1894464117002));
#46896=CARTESIAN_POINT('Ctrl Pts',(31.9415062364773,1.48092155721679,14.8542422440378));
#46897=CARTESIAN_POINT('Ctrl Pts',(31.8025947459886,-1.16082604986853,14.7727220828024));
#46898=CARTESIAN_POINT('Ctrl Pts',(31.6636832555,-3.51975640787564,15.9647470499492));
#46899=CARTESIAN_POINT('Ctrl Pts',(31.5247717650114,-5.0211527496418,18.1398987644648));
#46900=CARTESIAN_POINT('Ctrl Pts',(31.3858602745227,-5.29922316069158,20.7682352731195));
#46901=CARTESIAN_POINT('Ctrl Pts',(31.2469487840341,-4.28622010149303,23.209403181782));
#46902=CARTESIAN_POINT('Ctrl Pts',(31.1080372935454,-2.22894604390901,24.8686498205372));
#46903=CARTESIAN_POINT('Ctrl Pts',(30.9691258030568,0.371376120282793,25.3417255001506));
#46904=CARTESIAN_POINT('Ctrl Pts',(30.8302143125681,2.88121825714956,24.5133726742142));
#46905=CARTESIAN_POINT('Ctrl Pts',(30.6913028220796,4.68909628701403,22.5854066513387));
#46906=CARTESIAN_POINT('Ctrl Pts',(30.5523913315909,5.35454878920669,20.0275464277232));
#46907=CARTESIAN_POINT('Ctrl Pts',(30.4134798411023,4.7154485905101,17.4629749445598));
#46908=CARTESIAN_POINT('Ctrl Pts',(30.2745683506136,2.92750253442696,15.5165102372595));
#46909=CARTESIAN_POINT('Ctrl Pts',(30.135656860125,0.426315925592653,14.6623782193507));
#46910=CARTESIAN_POINT('Ctrl Pts',(29.9967453696363,-2.17873594137227,15.1086748994319));
#46911=CARTESIAN_POINT('Ctrl Pts',(29.8578338791477,-4.25297261386722,16.746667018676));
#46912=CARTESIAN_POINT('Ctrl Pts',(29.7189223886591,-5.29103852227984,19.1772832216213));
#46913=CARTESIAN_POINT('Ctrl Pts',(29.5800108981704,-5.04002502055383,21.8083415976708));
#46914=CARTESIAN_POINT('Ctrl Pts',(29.4410994076818,-3.56108765223307,23.9988256119501));
#46915=CARTESIAN_POINT('Ctrl Pts',(29.3021879171931,-1.21454655151411,25.2150578343754));
#46916=CARTESIAN_POINT('Ctrl Pts',(29.1632764267045,1.4278999646765,25.1607221619219));
#46917=CARTESIAN_POINT('Ctrl Pts',(29.0243649362159,3.72246081788218,23.8490566378019));
#46918=CARTESIAN_POINT('Ctrl Pts',(28.8854534457272,5.11010187166212,21.5996282077128));
#46919=CARTESIAN_POINT('Ctrl Pts',(28.7465419552387,5.25274592178536,18.960475193734));
#46920=CARTESIAN_POINT('Ctrl Pts',(28.6076304647499,4.11563995951487,16.5745862636289));
#46921=CARTESIAN_POINT('Ctrl Pts',(28.4687189742614,1.97582220276126,15.0232462222096));
#46922=CARTESIAN_POINT('Ctrl Pts',(28.3298074837727,-0.645373965612155,
14.6844149911618));
#46923=CARTESIAN_POINT('Ctrl Pts',(28.1908959932841,-3.10933478455334,15.6406435406999));
#46924=CARTESIAN_POINT('Ctrl Pts',(28.0519845027954,-4.81575444534233,17.6589616270038));
#46925=CARTESIAN_POINT('Ctrl Pts',(27.9130730123068,-5.34889028413044,20.2476373760362));
#46926=CARTESIAN_POINT('Ctrl Pts',(27.7741615218182,-4.57885202896163,22.7759801221459));
#46927=CARTESIAN_POINT('Ctrl Pts',(27.6352500313295,-2.69324754841923,24.6279983993741));
#46928=CARTESIAN_POINT('Ctrl Pts',(27.4963385408409,-0.151475106435163,
25.352476700912));
#46929=CARTESIAN_POINT('Ctrl Pts',(27.3574270503523,2.42720189408347,24.7729071337113));
#46930=CARTESIAN_POINT('Ctrl Pts',(27.2185155598636,4.41452882736344,23.0304928269264));
#46931=CARTESIAN_POINT('Ctrl Pts',(27.079604069375,5.32632433276681,20.5497459812053));
#46932=CARTESIAN_POINT('Ctrl Pts',(26.9406925788863,4.94044358800147,17.9350620601456));
#46933=CARTESIAN_POINT('Ctrl Pts',(26.8017810883977,3.35090044701153,15.8234682168224));
#46934=CARTESIAN_POINT('Ctrl Pts',(26.6628695979091,0.944962423716766,14.7294215156742));
#46935=CARTESIAN_POINT('Ctrl Pts',(26.5239581074204,-1.69120102671082,14.9194694539913));
#46936=CARTESIAN_POINT('Ctrl Pts',(26.3850466169318,-3.91532959726404,16.3473098014664));
#46937=CARTESIAN_POINT('Ctrl Pts',(26.2461351264432,-5.1855488839429,18.6650714199203));
#46938=CARTESIAN_POINT('Ctrl Pts',(26.1072236359545,-5.19238967348734,21.3080676665743));
#46939=CARTESIAN_POINT('Ctrl Pts',(25.9683121454659,-3.93418531370541,23.6323735296772));
#46940=CARTESIAN_POINT('Ctrl Pts',(25.8294006549773,-1.7174777674106,25.0717079628193));
#46941=CARTESIAN_POINT('Ctrl Pts',(25.6904891644886,0.917666578770842,25.2753994722563));
#46942=CARTESIAN_POINT('Ctrl Pts',(25.551577674,3.32923570676315,24.1938217833485));
#46943=CARTESIAN_POINT('Ctrl Pts',(25.4126661835114,4.92968823013898,22.0904845120939));
#46944=CARTESIAN_POINT('Ctrl Pts',(25.2737546930227,5.32909873329212,19.4778331373023));
#46945=CARTESIAN_POINT('Ctrl Pts',(25.1348432025341,4.43015704665191,16.9923996136994));
#46946=CARTESIAN_POINT('Ctrl Pts',(24.9959317120454,2.45187635908171,15.2397212412033));
#46947=CARTESIAN_POINT('Ctrl Pts',(24.8570202215568,-0.123765946134771,
14.6468109007572));
#46948=CARTESIAN_POINT('Ctrl Pts',(24.7181087310681,-2.6692545996311,15.3581219938452));
#46949=CARTESIAN_POINT('Ctrl Pts',(24.5791972405796,-4.56442080124713,17.2003546133809));
#46950=CARTESIAN_POINT('Ctrl Pts',(24.4402857500909,-5.34753672212527,19.7246773761623));
#46951=CARTESIAN_POINT('Ctrl Pts',(24.3013742596023,-4.82780832341947,22.3160782227716));
#46952=CARTESIAN_POINT('Ctrl Pts',(24.1624627691136,-3.13185936241575,24.3432025598312));
#46953=CARTESIAN_POINT('Ctrl Pts',(24.023551278625,-0.672881479482988,25.3121730069948));
#46954=CARTESIAN_POINT('Ctrl Pts',(23.8846397881364,1.95003353167377,24.9869149548617));
#46955=CARTESIAN_POINT('Ctrl Pts',(23.7457282976477,4.09785314063762,23.4466724792822));
#46956=CARTESIAN_POINT('Ctrl Pts',(23.6068168071591,5.24729443745648,21.0667017522782));
#46957=CARTESIAN_POINT('Ctrl Pts',(23.4679053166704,5.11831389142216,18.4268457003364));
#46958=CARTESIAN_POINT('Ctrl Pts',(23.3289938261818,3.74233561058096,16.1702642755077));
#46959=CARTESIAN_POINT('Ctrl Pts',(23.1900823356931,1.45459534556316,14.8467385160133));
#46960=CARTESIAN_POINT('Ctrl Pts',(23.0511708452045,-1.1875344976354,14.7787249298087));
#46961=CARTESIAN_POINT('Ctrl Pts',(22.9122593547159,-3.54033999301738,15.9827939714875));
#46962=CARTESIAN_POINT('Ctrl Pts',(22.7733478642272,-5.03059660113046,18.1655929082208));
#46963=CARTESIAN_POINT('Ctrl Pts',(22.6344363737386,-5.29522643069642,20.7953166597835));
#46964=CARTESIAN_POINT('Ctrl Pts',(22.49552488325,-4.26975653124141,23.2312738518418));
#46965=CARTESIAN_POINT('Ctrl Pts',(22.3566133927614,-2.20402672675047,24.8799813247024));
#46966=CARTESIAN_POINT('Ctrl Pts',(22.2177019022727,0.398679979512333,25.3397570933153));
#46967=CARTESIAN_POINT('Ctrl Pts',(22.0787904117841,2.90425449695062,24.4985839281508));
#46968=CARTESIAN_POINT('Ctrl Pts',(21.9398789212954,4.70225248512023,22.5614006144795));
#46969=CARTESIAN_POINT('Ctrl Pts',(21.8009674308068,5.35461964215578,20.0001717983347));
#46970=CARTESIAN_POINT('Ctrl Pts',(21.6620559403182,4.70241683608078,17.4389011261923));
#46971=CARTESIAN_POINT('Ctrl Pts',(21.5231444498295,2.9045431573112,15.5016024420921));
#46972=CARTESIAN_POINT('Ctrl Pts',(21.3842329593409,0.399022621656567,14.6602685002819));
#46973=CARTESIAN_POINT('Ctrl Pts',(21.2453214688522,-2.20371358226263,15.1198772567664));
#46974=CARTESIAN_POINT('Ctrl Pts',(21.1064099783636,-4.26954917720392,16.7684521719287));
#46975=CARTESIAN_POINT('Ctrl Pts',(20.967498487875,-5.29517538570201,19.2043435563444));
#46976=CARTESIAN_POINT('Ctrl Pts',(20.8285869973863,-5.03071430149971,21.8340842833308));
#46977=CARTESIAN_POINT('Ctrl Pts',(20.6896755068977,-3.54059776288221,24.0169788427559));
#46978=CARTESIAN_POINT('Ctrl Pts',(20.550764016409,-1.18786953536933,25.2211988574097));
#46979=CARTESIAN_POINT('Ctrl Pts',(20.4118525259204,1.4542646667037,25.1533548122415));
#46980=CARTESIAN_POINT('Ctrl Pts',(20.2729410354318,3.74208985536738,23.8299758558027));
#46981=CARTESIAN_POINT('Ctrl Pts',(20.1340295449431,5.11821293429771,21.5734827297631));
#46982=CARTESIAN_POINT('Ctrl Pts',(19.9951180544545,5.24736287505752,18.9336349597145));
#46983=CARTESIAN_POINT('Ctrl Pts',(19.8562065639659,4.0980742992049,16.5535904799529));
#46984=CARTESIAN_POINT('Ctrl Pts',(19.7172950734773,1.9503535293551,15.0132101856798));
#46985=CARTESIAN_POINT('Ctrl Pts',(19.5783835829886,-0.672540605155714,
14.6877838263027));
#46986=CARTESIAN_POINT('Ctrl Pts',(19.4394720925,-3.13158066018142,15.6565964831191));
#46987=CARTESIAN_POINT('Ctrl Pts',(19.3005606020113,-4.8276596947516,17.6836119898977));
#46988=CARTESIAN_POINT('Ctrl Pts',(19.1616491115227,-5.3475543780918,20.2749794811006));
#46989=CARTESIAN_POINT('Ctrl Pts',(19.0227376210341,-4.56460044024587,22.7993524898773));
#46990=CARTESIAN_POINT('Ctrl Pts',(18.8838261305454,-2.66955245540832,24.6417067151532));
#46991=CARTESIAN_POINT('Ctrl Pts',(18.7449146400568,-0.124109450753522,
25.3531811463754));
#46992=CARTESIAN_POINT('Ctrl Pts',(18.6060031495681,2.45157089518999,24.760436081656));
#46993=CARTESIAN_POINT('Ctrl Pts',(18.4670916590795,4.4299640450231,23.0078846556139));
#46994=CARTESIAN_POINT('Ctrl Pts',(18.3281801685909,5.32906521577738,20.5225088206591));
#46995=CARTESIAN_POINT('Ctrl Pts',(18.1892686781023,4.92982236276058,17.9098318217663));
#46996=CARTESIAN_POINT('Ctrl Pts',(18.0503571876136,3.32950481018978,15.8063918565752));
#46997=CARTESIAN_POINT('Ctrl Pts',(17.911445697125,0.918005090129485,14.7246594236797));
#46998=CARTESIAN_POINT('Ctrl Pts',(17.7725342066363,-1.71715232115819,14.9281818400483));
#46999=CARTESIAN_POINT('Ctrl Pts',(17.6336227161477,-3.93395222248708,16.3673740279429));
#47000=CARTESIAN_POINT('Ctrl Pts',(17.4947112256591,-5.19230572636053,18.6915991494658));
#47001=CARTESIAN_POINT('Ctrl Pts',(17.3557997351705,-5.18563453332208,21.3345958296401));
#47002=CARTESIAN_POINT('Ctrl Pts',(17.2168882446818,-3.91556397600737,23.652438951094));
#47003=CARTESIAN_POINT('Ctrl Pts',(17.0779767541931,-1.69152703207546,25.0804220141079));
#47004=CARTESIAN_POINT('Ctrl Pts',(16.9390652637045,0.94462421787777,25.2706391100771));
#47005=CARTESIAN_POINT('Ctrl Pts',(16.8001537732159,3.35063243930134,24.1767467960574));
#47006=CARTESIAN_POINT('Ctrl Pts',(16.6612422827273,4.9403110743387,22.0652549553122));
#47007=CARTESIAN_POINT('Ctrl Pts',(16.5223307922386,5.3263595980486,19.4505958009346));
#47008=CARTESIAN_POINT('Ctrl Pts',(16.38341930175,4.41472327975128,16.9697904519824));
#47009=CARTESIAN_POINT('Ctrl Pts',(16.2445078112613,2.42750815827123,15.227248625457));
#47010=CARTESIAN_POINT('Ctrl Pts',(16.1055963207727,-0.151131646963111,
14.6475135902124));
#47011=CARTESIAN_POINT('Ctrl Pts',(15.9666848302841,-2.69295057223214,15.3718287891231));
#47012=CARTESIAN_POINT('Ctrl Pts',(15.8277733397954,-4.57867388969788,17.2237260665644));
#47013=CARTESIAN_POINT('Ctrl Pts',(15.6888618493068,-5.34887438265668,19.7520193954475));
#47014=CARTESIAN_POINT('Ctrl Pts',(15.5499503588182,-4.81590465580583,22.3407293495539));
#47015=CARTESIAN_POINT('Ctrl Pts',(15.4110388683295,-3.10961451050615,24.3591569296969));
#47016=CARTESIAN_POINT('Ctrl Pts',(15.2721273778409,-0.645715056167731,
25.3155435853648));
#47017=CARTESIAN_POINT('Ctrl Pts',(15.1332158873523,1.97550284902251,24.9768805526333));
#47018=CARTESIAN_POINT('Ctrl Pts',(14.9943043968636,4.11542014817447,23.4256778228074));
#47019=CARTESIAN_POINT('Ctrl Pts',(14.855392906375,5.25267920646456,21.0398618637348));
#47020=CARTESIAN_POINT('Ctrl Pts',(14.7164814158863,5.11020450651333,18.4006997019677));
#47021=CARTESIAN_POINT('Ctrl Pts',(14.5775699253977,3.72270779751692,16.1511822339864));
#47022=CARTESIAN_POINT('Ctrl Pts',(14.4386584349091,1.42823111634034,14.8393694745707));
#47023=CARTESIAN_POINT('Ctrl Pts',(14.2997469444204,-1.21421190778405,14.7848642410124));
#47024=CARTESIAN_POINT('Ctrl Pts',(14.1608354539318,-3.56083104718738,16.0009458874552));
#47025=CARTESIAN_POINT('Ctrl Pts',(14.0219239634432,-5.03990897202894,18.1913349963752));
#47026=CARTESIAN_POINT('Ctrl Pts',(13.8830124729545,-5.29109130369761,20.8223772599062));
#47027=CARTESIAN_POINT('Ctrl Pts',(13.7441009824659,-4.2531813658544,23.2530600687389));
#47028=CARTESIAN_POINT('Ctrl Pts',(13.6051894919772,-2.17904980474738,24.8911852847859));
#47029=CARTESIAN_POINT('Ctrl Pts',(13.4662780014886,0.425973418769273,25.3376491256149));
#47030=CARTESIAN_POINT('Ctrl Pts',(13.327366511,2.92721483062653,24.4836776062776));
#47031=CARTESIAN_POINT('Ctrl Pts',(13.1884550205113,4.71528578429796,22.5373276323866));
#47032=CARTESIAN_POINT('Ctrl Pts',(13.0495435300227,5.3545505457894,19.9727971644561));
#47033=CARTESIAN_POINT('Ctrl Pts',(12.9106320395341,4.68926217842746,17.414894245172));
#47034=CARTESIAN_POINT('Ctrl Pts',(12.7717205490454,2.8815078665258,15.4868122178637));
#47035=CARTESIAN_POINT('Ctrl Pts',(12.6328090585568,0.371718888792551,14.6582983414094));
#47036=CARTESIAN_POINT('Ctrl Pts',(12.4938975680682,-2.22863362649285,15.1312071618788));
#47037=CARTESIAN_POINT('Ctrl Pts',(12.3549860775795,-4.28601415082467,16.7903217855047));
#47038=CARTESIAN_POINT('Ctrl Pts',(12.2160745870909,-5.29917385345463,19.2314246864894));
#47039=CARTESIAN_POINT('Ctrl Pts',(12.0771630966022,-5.02127209877919,21.8597790330297));
#47040=CARTESIAN_POINT('Ctrl Pts',(11.9382516061136,-3.52001533582255,24.03502708507));
#47041=CARTESIAN_POINT('Ctrl Pts',(11.799340115625,-1.16116147284977,25.2272034182385));
#47042=CARTESIAN_POINT('Ctrl Pts',(11.6604286251363,1.48059135980434,25.1458527735399));
#47043=CARTESIAN_POINT('Ctrl Pts',(11.5215171346477,3.76162108890966,23.8107949728561));
#47044=CARTESIAN_POINT('Ctrl Pts',(11.3826056441591,5.12619022638666,21.5472961269818));
#47045=CARTESIAN_POINT('Ctrl Pts',(11.2436941536704,5.24184268229665,18.9068225964061));
#47046=CARTESIAN_POINT('Ctrl Pts',(11.1047826631818,4.0804015308777,16.5326847722646));
#47047=CARTESIAN_POINT('Ctrl Pts',(10.9658711726932,1.92483388115344,15.0033044847981));
#47048=CARTESIAN_POINT('Ctrl Pts',(10.8269596822045,-0.69968966705539,14.6912915024941));
#47049=CARTESIAN_POINT('Ctrl Pts',(10.6880481917159,-3.15374468824635,15.6726629455249));
#47050=CARTESIAN_POINT('Ctrl Pts',(10.5491367012272,-4.83943876756671,17.708322894331));
#47051=CARTESIAN_POINT('Ctrl Pts',(10.4102252107386,-5.34607870739673,20.3023143992512));
#47052=CARTESIAN_POINT('Ctrl Pts',(10.27131372025,-4.55022955030055,22.8226516932216));
#47053=CARTESIAN_POINT('Ctrl Pts',(10.1324022297614,-2.64578759048757,24.6552937144392));
#47054=CARTESIAN_POINT('Ctrl Pts',(9.99349073927269,-0.096740551324623,
25.3537456801201));
#47055=CARTESIAN_POINT('Ctrl Pts',(9.85457924878407,2.47587582159254,24.7478406099751));
#47056=CARTESIAN_POINT('Ctrl Pts',(9.71566775829542,4.44528348033462,22.9851978696795));
#47057=CARTESIAN_POINT('Ctrl Pts',(9.5767562678068,5.33166681736764,20.4952580037272));
#47058=CARTESIAN_POINT('Ctrl Pts',(9.43784477731815,4.91907229078337,17.8846562124036));
#47059=CARTESIAN_POINT('Ctrl Pts',(9.29893328682952,3.30802215282312,15.7894251012354));
#47060=CARTESIAN_POINT('Ctrl Pts',(9.16002179634088,0.891023763393785,14.7200352089486));
#47061=CARTESIAN_POINT('Ctrl Pts',(9.02111030585224,-1.74305873579932,14.9370267840696));
#47062=CARTESIAN_POINT('Ctrl Pts',(8.8821988153636,-3.95247202921743,16.3875331973942));
#47063=CARTESIAN_POINT('Ctrl Pts',(8.74328732487497,-5.19892686172881,18.7181610756146));
#47064=CARTESIAN_POINT('Ctrl Pts',(8.60437583438634,-5.17874386046697,21.3610891114658));
#47065=CARTESIAN_POINT('Ctrl Pts',(8.46546434389769,-3.89684030041517,23.6724089117002));
#47066=CARTESIAN_POINT('Ctrl Pts',(8.32655285340906,-1.66553208668131,25.0890032825603));
#47067=CARTESIAN_POINT('Ctrl Pts',(8.18764136292043,0.971557168113871,25.2657409935129));
#47068=CARTESIAN_POINT('Ctrl Pts',(8.0487298724318,3.37194159909904,24.1595626445505));
#47069=CARTESIAN_POINT('Ctrl Pts',(7.90981838194316,4.95080479766731,22.0399714206502));
#47070=CARTESIAN_POINT('Ctrl Pts',(7.77090689145451,5.32348125209927,19.423372823895));
#47071=CARTESIAN_POINT('Ctrl Pts',(7.63199540096589,4.39917412883777,16.9472604883745));
#47072=CARTESIAN_POINT('Ctrl Pts',(7.49308391047725,2.40307651166472,15.2149007512111));
#47073=CARTESIAN_POINT('Ctrl Pts',(7.35417241998861,-0.17849339778717,14.6483561732285));
#47074=CARTESIAN_POINT('Ctrl Pts',(7.21526092949998,-2.71657616138589,15.3856565471278));
#47075=CARTESIAN_POINT('Ctrl Pts',(7.07634943901133,-4.59280730909292,17.2471700809498));
#47076=CARTESIAN_POINT('Ctrl Pts',(6.93743794852271,-5.3500722440318,19.7793678959993));
#47077=CARTESIAN_POINT('Ctrl Pts',(6.79852645803405,-4.80387511882975,22.3653192986072));
#47078=CARTESIAN_POINT('Ctrl Pts',(6.65961496754543,-3.08728838514452,24.3749973678423));
#47079=CARTESIAN_POINT('Ctrl Pts',(6.52070347705679,-0.61853175632593,25.3187752357184));
#47080=CARTESIAN_POINT('Ctrl Pts',(6.38179198656815,2.0009205342686,24.9667160737471));
#47081=CARTESIAN_POINT('Ctrl Pts',(6.24288049607952,4.13287959433989,23.4045936321923));
#47082=CARTESIAN_POINT('Ctrl Pts',(6.10396900559087,5.25792669049103,21.0129947971718));
#47083=CARTESIAN_POINT('Ctrl Pts',(5.96505751510225,5.10196156036751,18.3745955032032));
#47084=CARTESIAN_POINT('Ctrl Pts',(5.82614602461359,3.70298268708293,16.1322007858681));
#47085=CARTESIAN_POINT('Ctrl Pts',(5.68723453412498,1.40182955860857,14.8321353123087));
#47086=CARTESIAN_POINT('Ctrl Pts',(5.54832304363632,-1.24085758306887,14.7911398559554));
#47087=CARTESIAN_POINT('Ctrl Pts',(5.40941155314771,-3.58122903482779,16.0192023234305));
#47088=CARTESIAN_POINT('Ctrl Pts',(5.27050006265906,-5.04908961894742,18.2171243561278));
#47089=CARTESIAN_POINT('Ctrl Pts',(5.13158857217043,-5.28681788777155,20.8494163662269));
#47090=CARTESIAN_POINT('Ctrl Pts',(4.9926770816818,-4.23649503854359,23.2747612630649));
#47091=CARTESIAN_POINT('Ctrl Pts',(4.85376559119315,-2.15401593070123,24.9022614079586));
#47092=CARTESIAN_POINT('Ctrl Pts',(4.71485410070452,0.453255724707226,25.3354016521434));
#47093=CARTESIAN_POINT('Ctrl Pts',(4.57594261021588,2.95009865808178,24.4686540981888));
#47094=CARTESIAN_POINT('Ctrl Pts',(4.43703111972724,4.72819584390646,22.5131883342361));
#47095=CARTESIAN_POINT('Ctrl Pts',(4.29811962923862,5.35434150191347,19.9454232415558));
#47096=CARTESIAN_POINT('Ctrl Pts',(4.15920813874997,4.67598496136272,17.3909549289472));
#47097=CARTESIAN_POINT('Ctrl Pts',(4.02029664826134,2.85839726412539,15.4721399511341));
#47098=CARTESIAN_POINT('Ctrl Pts',(3.88138515777269,0.344405440615539,14.6564677942253));
#47099=CARTESIAN_POINT('Ctrl Pts',(3.74247366728406,-2.25349542274803,15.1426643186491));
#47100=CARTESIAN_POINT('Ctrl Pts',(3.60356217679542,-4.30236710439854,16.8122752878152));
#47101=CARTESIAN_POINT('Ctrl Pts',(3.46465068630679,-5.30303382103181,19.25852590426));
#47102=CARTESIAN_POINT('Ctrl Pts',(3.32573919581815,-5.01169865917778,21.885425175202));
#47103=CARTESIAN_POINT('Ctrl Pts',(3.18682770532951,-3.49934090899555,24.0529698671851));
#47104=CARTESIAN_POINT('Ctrl Pts',(3.04791621484087,-1.13442306201116,25.2330713599164));
#47105=CARTESIAN_POINT('Ctrl Pts',(2.90900472435224,1.5068793559172,25.1382162419096));
#47106=CARTESIAN_POINT('Ctrl Pts',(2.77009323386361,3.78105400800197,23.7915144902417));
#47107=CARTESIAN_POINT('Ctrl Pts',(2.63118174337497,5.13403353950245,21.5210690838564));
#47108=CARTESIAN_POINT('Ctrl Pts',(2.49227025288633,5.23618548764273,18.8800388044447));
#47109=CARTESIAN_POINT('Ctrl Pts',(2.3533587623977,4.06262211670135,16.5118696872292));
#47110=CARTESIAN_POINT('Ctrl Pts',(2.21444727190906,1.8992639246118,14.99352937793));
#47111=CARTESIAN_POINT('Ctrl Pts',(2.07553578142043,-0.726820440693177,
14.694937929106));
#47112=CARTESIAN_POINT('Ctrl Pts',(1.93662429093179,-3.17582629152359,15.6888425059388));
#47113=CARTESIAN_POINT('Ctrl Pts',(1.79771280044315,-4.8510913518727,17.7330936985172));
#47114=CARTESIAN_POINT('Ctrl Pts',(1.65880130995451,-5.34446331860061,20.3296414080563));
#47115=CARTESIAN_POINT('Ctrl Pts',(1.51988981946587,-4.53573971899385,22.8458771389863));
#47116=CARTESIAN_POINT('Ctrl Pts',(1.38097832897724,-2.62195360576743,24.6687590110773));
#47117=CARTESIAN_POINT('Ctrl Pts',(1.24206683848861,-0.0693690624308824,
25.3541703485356));
#47118=CARTESIAN_POINT('Ctrl Pts',(1.10315534799997,2.50011591782952,24.7351209274301));
#47119=CARTESIAN_POINT('Ctrl Pts',(0.964243857511331,4.46048696971124,22.9624332992928));
#47120=CARTESIAN_POINT('Ctrl Pts',(0.82533236702269,5.33412860310603,20.467993775381));
#47121=CARTESIAN_POINT('Ctrl Pts',(0.686420876534053,4.90819457177639,17.8595368104176));
#47122=CARTESIAN_POINT('Ctrl Pts',(0.54750938604542,3.28645122673724,15.7725665813991));
#47123=CARTESIAN_POINT('Ctrl Pts',(0.408597895556785,0.864022713178557,
14.7155525631285));
#47124=CARTESIAN_POINT('Ctrl Pts',(0.269686405068149,-1.76892661457066,
14.9459970213854));
#47125=CARTESIAN_POINT('Ctrl Pts',(0.130774914579505,-3.97087470340791,
16.4078006379552));
#47126=CARTESIAN_POINT('Ctrl Pts',(-0.00813657590912362,-5.20543936546245,
18.7447292011997));
#47127=CARTESIAN_POINT('Ctrl Pts',(-0.147048066397761,-5.17166407855605,
21.3876007430961));
#47128=CARTESIAN_POINT('Ctrl Pts',(-0.285959556886395,-3.87812163490998,
23.6921750166713));
#47129=CARTESIAN_POINT('Ctrl Pts',(-0.424871047375028,-1.63927203245633,
25.0976827974512));
#47130=CARTESIAN_POINT('Ctrl Pts',(-0.517478707700787,0.118837970738912,
25.205896478639));
#47131=CARTESIAN_POINT('Ctrl Pts',(-0.563782537863666,0.957839028560417,
25.0466568099948));
#47132=CARTESIAN_POINT('Ctrl Pts',(50.1879275126212,4.1258079218636,23.5796485937013));
#47133=CARTESIAN_POINT('Ctrl Pts',(50.1416236824583,4.72092050229439,22.8937376349937));
#47134=CARTESIAN_POINT('Ctrl Pts',(50.0490160221326,5.56184096807278,21.220063777147));
#47135=CARTESIAN_POINT('Ctrl Pts',(49.9101045316439,5.46761903977869,18.4106716448697));
#47136=CARTESIAN_POINT('Ctrl Pts',(49.7711930411553,4.04148516076094,15.9891741090619));
#47137=CARTESIAN_POINT('Ctrl Pts',(49.6322815506667,1.63061710874887,14.5445190619427));
#47138=CARTESIAN_POINT('Ctrl Pts',(49.4933700601781,-1.17748087672893,14.4291752694788));
#47139=CARTESIAN_POINT('Ctrl Pts',(49.3544585696893,-3.69872652215335,15.6709912525866));
#47140=CARTESIAN_POINT('Ctrl Pts',(49.2155470792008,-5.31882339208546,17.9675462714425));
#47141=CARTESIAN_POINT('Ctrl Pts',(49.076635588712,-5.64307732183502,20.7592551383084));
#47142=CARTESIAN_POINT('Ctrl Pts',(48.9377240982236,-4.59248009632072,23.3659944223523));
#47143=CARTESIAN_POINT('Ctrl Pts',(48.7988126077348,-2.42299787900316,25.1526557522133));
#47144=CARTESIAN_POINT('Ctrl Pts',(48.6599011172463,0.336810924398074,25.6839553589829));
#47145=CARTESIAN_POINT('Ctrl Pts',(48.5209896267575,3.01456058714978,24.8304460084601));
#47146=CARTESIAN_POINT('Ctrl Pts',(48.382078136269,4.95785955026221,22.8000742051481));
#47147=CARTESIAN_POINT('Ctrl Pts',(48.2431666457803,5.69325288857485,20.0875074076531));
#47148=CARTESIAN_POINT('Ctrl Pts',(48.1042551552917,5.04157358005871,17.3536209794161));
#47149=CARTESIAN_POINT('Ctrl Pts',(47.965343664803,3.16159309676431,15.264483626389));
#47150=CARTESIAN_POINT('Ctrl Pts',(47.8264321743145,0.51133954173023,14.329081383812));
#47151=CARTESIAN_POINT('Ctrl Pts',(47.6875206838257,-2.26349396242014,14.7753104148998));
#47152=CARTESIAN_POINT('Ctrl Pts',(47.5486091933372,-4.48686229249669,16.4944539801099));
#47153=CARTESIAN_POINT('Ctrl Pts',(47.4096977028484,-5.61707627036106,19.0676694146596));
#47154=CARTESIAN_POINT('Ctrl Pts',(47.2707862123599,-5.3787768005542,21.8680327282576));
#47155=CARTESIAN_POINT('Ctrl Pts',(47.1318747218712,-3.83002185139275,24.2132788609653));
#47156=CARTESIAN_POINT('Ctrl Pts',(46.9929632313826,-1.34814152629545,25.5320249972138));
#47157=CARTESIAN_POINT('Ctrl Pts',(46.854051740894,1.46219255614692,25.5029791087937));
#47158=CARTESIAN_POINT('Ctrl Pts',(46.7151402504053,3.91628611802883,24.1332177762222));
#47159=CARTESIAN_POINT('Ctrl Pts',(46.5762287599167,5.41623735456965,21.7564620868539));
#47160=CARTESIAN_POINT('Ctrl Pts',(46.437317269428,5.59660642879563,18.9517716733247));
#47161=CARTESIAN_POINT('Ctrl Pts',(46.2984057789394,4.4134492153806,16.4024658212954));
#47162=CARTESIAN_POINT('Ctrl Pts',(46.1594942884507,2.15502360479501,14.729643332142));
#47163=CARTESIAN_POINT('Ctrl Pts',(46.0205827979622,-0.62844005751078,14.3408614403073));
#47164=CARTESIAN_POINT('Ctrl Pts',(45.8816713074735,-3.2587940542495,15.330840819199));
#47165=CARTESIAN_POINT('Ctrl Pts',(45.7427598169849,-5.09519346163427,17.4583883592892));
#47166=CARTESIAN_POINT('Ctrl Pts',(45.6038483264962,-5.69022806806176,20.2051601255532));
#47167=CARTESIAN_POINT('Ctrl Pts',(45.4649368360076,-4.89892692761397,22.9019478116558));
#47168=CARTESIAN_POINT('Ctrl Pts',(45.326025345519,-2.91407828083651,24.8917209565584));
#47169=CARTESIAN_POINT('Ctrl Pts',(45.1871138550302,-0.219259692328256,
25.6897022181302));
#47170=CARTESIAN_POINT('Ctrl Pts',(45.0482023645418,2.52897811693668,25.1014758480003));
#47171=CARTESIAN_POINT('Ctrl Pts',(44.9092908740529,4.66106966200288,23.2703540709886));
#47172=CARTESIAN_POINT('Ctrl Pts',(44.7703793835645,5.6575639315609,20.6424612859748));
#47173=CARTESIAN_POINT('Ctrl Pts',(44.6314678930757,5.27568056409961,17.8580427807128));
#47174=CARTESIAN_POINT('Ctrl Pts',(44.4925564025872,3.60845951462895,15.5954789051522));
#47175=CARTESIAN_POINT('Ctrl Pts',(44.3536449120985,1.0620933137783,14.4060082287777));
#47176=CARTESIAN_POINT('Ctrl Pts',(44.2147334216099,-1.74303543750027,14.5794268193028));
#47177=CARTESIAN_POINT('Ctrl Pts',(44.0758219311212,-4.12350065927285,16.0734839288943));
#47178=CARTESIAN_POINT('Ctrl Pts',(43.9369104406326,-5.49933894907755,18.5241757330787));
#47179=CARTESIAN_POINT('Ctrl Pts',(43.797998950144,-5.53534866292723,21.3344292126242));
#47180=CARTESIAN_POINT('Ctrl Pts',(43.6590874596553,-4.22275659297371,23.8195697270992));
#47181=CARTESIAN_POINT('Ctrl Pts',(43.5201759691667,-1.88135542342509,25.3741313637112));
#47182=CARTESIAN_POINT('Ctrl Pts',(43.381264478678,0.918408793241331,25.6193693091104));
#47183=CARTESIAN_POINT('Ctrl Pts',(43.2423529881894,3.49441696268329,24.4955351444057));
#47184=CARTESIAN_POINT('Ctrl Pts',(43.1034414977008,5.21906467839467,22.2764336200312));
#47185=CARTESIAN_POINT('Ctrl Pts',(42.9645300072122,5.67216829387492,19.5027143782138));
#47186=CARTESIAN_POINT('Ctrl Pts',(42.8256185167235,4.74333614614231,16.8501510594355));
#47187=CARTESIAN_POINT('Ctrl Pts',(42.6867070262348,2.65886377095513,14.9649995440738));
#47188=CARTESIAN_POINT('Ctrl Pts',(42.5477955357463,-0.0733994919886356,
14.3065477381249));
#47189=CARTESIAN_POINT('Ctrl Pts',(42.4088840452575,-2.78778010799291,15.0352172038291));
#47190=CARTESIAN_POINT('Ctrl Pts',(42.269972554769,-4.82296137171968,16.9734789360431));
#47191=CARTESIAN_POINT('Ctrl Pts',(42.1310610642803,-5.68310295769733,19.649105548794));
#47192=CARTESIAN_POINT('Ctrl Pts',(41.9921495737917,-5.15864471934614,22.4102221481095));
#47193=CARTESIAN_POINT('Ctrl Pts',(41.8532380833031,-3.37736276596667,24.5841255317385));
#47194=CARTESIAN_POINT('Ctrl Pts',(41.7143265928144,-0.773238797008643,
25.6411778828961));
#47195=CARTESIAN_POINT('Ctrl Pts',(41.5754151023258,2.01927280287421,25.3238448034525));
#47196=CARTESIAN_POINT('Ctrl Pts',(41.4365036118371,4.3198199268461,23.7094395726711));
#47197=CARTESIAN_POINT('Ctrl Pts',(41.2975921213485,5.56790997651105,21.1912869667481));
#47198=CARTESIAN_POINT('Ctrl Pts',(41.1586806308598,5.45946518372445,18.3828957821538));
#47199=CARTESIAN_POINT('Ctrl Pts',(41.0197691403712,4.0209064390032,15.9684869400611));
#47200=CARTESIAN_POINT('Ctrl Pts',(40.8808576498826,1.60271625164799,14.5362936791607));
#47201=CARTESIAN_POINT('Ctrl Pts',(40.7419461593939,-1.20595087357003,14.4352476574235));
#47202=CARTESIAN_POINT('Ctrl Pts',(40.6030346689053,-3.72080678682811,15.6899671696414));
#47203=CARTESIAN_POINT('Ctrl Pts',(40.4641231784166,-5.32914587965345,17.9947592820193));
#47204=CARTESIAN_POINT('Ctrl Pts',(40.325211687928,-5.63912129620631,20.7880971706253));
#47205=CARTESIAN_POINT('Ctrl Pts',(40.1863001974394,-4.57521233758331,23.3894274162019));
#47206=CARTESIAN_POINT('Ctrl Pts',(40.0473887069508,-2.3966239078969,25.1649762814336));
#47207=CARTESIAN_POINT('Ctrl Pts',(39.9084772164621,0.365864737315575,25.6821588448111));
#47208=CARTESIAN_POINT('Ctrl Pts',(39.7695657259735,3.03921611811703,24.8149716023101));
#47209=CARTESIAN_POINT('Ctrl Pts',(39.6306542354848,4.97210966548392,22.7746912653621));
#47210=CARTESIAN_POINT('Ctrl Pts',(39.4917427449962,5.69362586835836,20.0584004694827));
#47211=CARTESIAN_POINT('Ctrl Pts',(39.3528312545076,5.02797850305467,17.3278813056873));
#47212=CARTESIAN_POINT('Ctrl Pts',(39.2139197640189,3.13734221816271,15.2483823859859));
#47213=CARTESIAN_POINT('Ctrl Pts',(39.0750082735303,0.482341198642141,14.3265413448437));
#47214=CARTESIAN_POINT('Ctrl Pts',(38.9360967830416,-2.29017476718114,14.786950443412));
#47215=CARTESIAN_POINT('Ctrl Pts',(38.7971852925531,-4.50472519834409,16.5174381511481));
#47216=CARTESIAN_POINT('Ctrl Pts',(38.6582738020644,-5.62176925584033,19.096397998141));
#47217=CARTESIAN_POINT('Ctrl Pts',(38.5193623115758,-5.36915649346304,21.8955064474643));
#47218=CARTESIAN_POINT('Ctrl Pts',(38.3804508210871,-3.80843208979058,24.2328041723104));
#47219=CARTESIAN_POINT('Ctrl Pts',(38.2415393305985,-1.31984232071061,25.5388448608114));
#47220=CARTESIAN_POINT('Ctrl Pts',(38.1026278401098,1.49030654363833,25.4954319711615));
#47221=CARTESIAN_POINT('Ctrl Pts',(37.9637163496212,3.93736535069332,24.113142380083));
#47222=CARTESIAN_POINT('Ctrl Pts',(37.8248048591326,5.42514620458289,21.7287494909833));
#47223=CARTESIAN_POINT('Ctrl Pts',(37.6858933686439,5.59117439311739,18.9231736215046));
#47224=CARTESIAN_POINT('Ctrl Pts',(37.5469818781553,4.39499972519705,16.3799497849901));
#47225=CARTESIAN_POINT('Ctrl Pts',(37.4080703876667,2.12805159201845,14.7186949940963));
#47226=CARTESIAN_POINT('Ctrl Pts',(37.269158897178,-0.657363280616373,14.3441481931567));
#47227=CARTESIAN_POINT('Ctrl Pts',(37.1302474066894,-3.2826217933125,15.347561896624));
#47228=CARTESIAN_POINT('Ctrl Pts',(36.9913359162008,-5.10812045787807,17.4844699303163));
#47229=CARTESIAN_POINT('Ctrl Pts',(36.8524244257121,-5.68910485950053,20.2342478202305));
#47230=CARTESIAN_POINT('Ctrl Pts',(36.7135129352235,-4.88402716657942,22.9269548646656));
#47231=CARTESIAN_POINT('Ctrl Pts',(36.5746014447348,-2.88903206283546,24.9065547875861));
#47232=CARTESIAN_POINT('Ctrl Pts',(36.4356899542462,-0.190169139617183,
25.690748794492));
#47233=CARTESIAN_POINT('Ctrl Pts',(36.2967784637576,2.55502554272399,25.0884801876104));
#47234=CARTESIAN_POINT('Ctrl Pts',(36.1578669732689,4.6777279098732,23.2464823647863));
#47235=CARTESIAN_POINT('Ctrl Pts',(36.0189554827803,5.66077447798464,20.6135295046474));
#47236=CARTESIAN_POINT('Ctrl Pts',(35.8800439922917,5.26466120927372,17.8310997037107));
#47237=CARTESIAN_POINT('Ctrl Pts',(35.741132501803,3.58589495331782,15.5770887949852));
#47238=CARTESIAN_POINT('Ctrl Pts',(35.6022210113144,1.03348105110547,14.4006515503426));
#47239=CARTESIAN_POINT('Ctrl Pts',(35.4633095208258,-1.77072446784502,14.5884086441555));
#47240=CARTESIAN_POINT('Ctrl Pts',(35.3243980303371,-4.14352045482631,16.0946159748226));
#47241=CARTESIAN_POINT('Ctrl Pts',(35.1854865398485,-5.50681199739401,18.552309505097));
#47242=CARTESIAN_POINT('Ctrl Pts',(35.0465750493599,-5.52845427177867,21.3627103538637));
#47243=CARTESIAN_POINT('Ctrl Pts',(34.9076635588712,-4.20317447375095,23.8411079764677));
#47244=CARTESIAN_POINT('Ctrl Pts',(34.7687520683826,-1.85385645552935,25.38367926106));
#47245=CARTESIAN_POINT('Ctrl Pts',(34.6298405778939,0.947124913112505,25.6146006574499));
#47246=CARTESIAN_POINT('Ctrl Pts',(34.4909290874053,3.51735399764575,24.4776117516954));
#47247=CARTESIAN_POINT('Ctrl Pts',(34.3520175969167,5.23063437590115,22.2497222427039));
#47248=CARTESIAN_POINT('Ctrl Pts',(34.213106106428,5.66955187670913,19.4737228287497));
#47249=CARTESIAN_POINT('Ctrl Pts',(34.0741946159394,4.72717106373549,16.825942678864));
#47250=CARTESIAN_POINT('Ctrl Pts',(33.9352831254507,2.63308839472643,14.9514723285663));
#47251=CARTESIAN_POINT('Ctrl Pts',(33.7963716349621,-0.102505391698266,
14.3069973837747));
#47252=CARTESIAN_POINT('Ctrl Pts',(33.6574601444735,-2.81312533049172,15.049534161453));
#47253=CARTESIAN_POINT('Ctrl Pts',(33.5185486539848,-4.83837094694631,16.9981751011391));
#47254=CARTESIAN_POINT('Ctrl Pts',(33.3796371634962,-5.68482258183033,19.6781640840627));
#47255=CARTESIAN_POINT('Ctrl Pts',(33.2407256730075,-5.14625543265696,22.4365633924698));
#47256=CARTESIAN_POINT('Ctrl Pts',(33.101814182519,-3.35388302585458,24.6013318498626));
#47257=CARTESIAN_POINT('Ctrl Pts',(32.9629026920303,-0.744389077706911,
25.6450572224439));
#47258=CARTESIAN_POINT('Ctrl Pts',(32.8239912015417,2.04646371505388,25.3134520235571));
#47259=CARTESIAN_POINT('Ctrl Pts',(32.685079711053,4.33872738819982,23.6873067128407));
#47260=CARTESIAN_POINT('Ctrl Pts',(32.5461682205644,5.57392747755557,21.1628063547411));
#47261=CARTESIAN_POINT('Ctrl Pts',(32.4072567300757,5.451126653732,18.3550062770187));
#47262=CARTESIAN_POINT('Ctrl Pts',(32.2683452395871,4.00024343137845,15.9479833868321));
#47263=CARTESIAN_POINT('Ctrl Pts',(32.1294337490985,1.57476298747406,14.5281714503324));
#47264=CARTESIAN_POINT('Ctrl Pts',(31.9905222586099,-1.23438401535882,14.4414856079792));
#47265=CARTESIAN_POINT('Ctrl Pts',(31.8516107681212,-3.74279251256509,15.7090455197518));
#47266=CARTESIAN_POINT('Ctrl Pts',(31.7126992776326,-5.33932770851822,18.022029887808));
#47267=CARTESIAN_POINT('Ctrl Pts',(31.5737877871439,-5.6350185836351,20.8169159722777));
#47268=CARTESIAN_POINT('Ctrl Pts',(31.4348762966553,-4.55782464581307,23.4127731600114));
#47269=CARTESIAN_POINT('Ctrl Pts',(31.2959648061666,-2.37018747814123,25.1771611392864));
#47270=CARTESIAN_POINT('Ctrl Pts',(31.157053315678,0.394909079284509,25.6802141652207));
#47271=CARTESIAN_POINT('Ctrl Pts',(31.0181418251894,3.06379216919554,24.7993711762741));
#47272=CARTESIAN_POINT('Ctrl Pts',(30.8792303347008,4.98622985228839,22.7492358945393));
#47273=CARTESIAN_POINT('Ctrl Pts',(30.7403188442121,5.6938500265429,20.0292919598639));
#47274=CARTESIAN_POINT('Ctrl Pts',(30.6014073537235,5.01425201995693,17.3022114938281));
#47275=CARTESIAN_POINT('Ctrl Pts',(30.4624958632348,3.11300933833137,15.2324053231072));
#47276=CARTESIAN_POINT('Ctrl Pts',(30.3235843727462,0.453330250560852,14.3241495943249));
#47277=CARTESIAN_POINT('Ctrl Pts',(30.1846728822575,-2.31679571631103,14.7987267181431));
#47278=CARTESIAN_POINT('Ctrl Pts',(30.045761391769,-4.52247036746897,16.5405133445784));
#47279=CARTESIAN_POINT('Ctrl Pts',(29.9068499012803,-5.62631530993781,19.125150197557));
#47280=CARTESIAN_POINT('Ctrl Pts',(29.7679384107917,-5.35939585701468,21.9229306257609));
#47281=CARTESIAN_POINT('Ctrl Pts',(29.629026920303,-3.78674279036552,24.2522188541149));
#47282=CARTESIAN_POINT('Ctrl Pts',(29.4901154298144,-1.29150861945937,25.5455199602506));
#47283=CARTESIAN_POINT('Ctrl Pts',(29.3512039393258,1.51838158019258,25.4877412038659));
#47284=CARTESIAN_POINT('Ctrl Pts',(29.2122924488371,3.95834167566592,24.0929594821304));
#47285=CARTESIAN_POINT('Ctrl Pts',(29.0733809583485,5.43391326198207,21.7009917121875));
#47286=CARTESIAN_POINT('Ctrl Pts',(28.9344694678598,5.58559622548734,18.8946037138217));
#47287=CARTESIAN_POINT('Ctrl Pts',(28.7955579773712,4.37643536649829,16.3575283629741));
#47288=CARTESIAN_POINT('Ctrl Pts',(28.6566464868826,2.10102396009786,14.7078846892032));
#47289=CARTESIAN_POINT('Ctrl Pts',(28.5177349963939,-0.686269322755631,
14.3475827683796));
#47290=CARTESIAN_POINT('Ctrl Pts',(28.3788235059053,-3.3063637371736,15.3644045710202));
#47291=CARTESIAN_POINT('Ctrl Pts',(28.2399120154166,-5.12091394735409,17.5106172476958));
#47292=CARTESIAN_POINT('Ctrl Pts',(28.101000524928,-5.68783295945715,20.2633293925641));
#47293=CARTESIAN_POINT('Ctrl Pts',(27.9620890344394,-4.86899975572019,22.9518854182492));
#47294=CARTESIAN_POINT('Ctrl Pts',(27.8231775439507,-2.86391033656552,24.9212603800031));
#47295=CARTESIAN_POINT('Ctrl Pts',(27.6842660534621,-0.161073616610791,
25.6916466364056));
#47296=CARTESIAN_POINT('Ctrl Pts',(27.5453545629735,2.58100618989778,25.0753515337742));
#47297=CARTESIAN_POINT('Ctrl Pts',(27.4064430724848,4.69426389979383,23.2225258079289));
#47298=CARTESIAN_POINT('Ctrl Pts',(27.2675315819962,5.66383707337432,20.5845816880009));
#47299=CARTESIAN_POINT('Ctrl Pts',(27.1286200915076,5.25350425630234,17.8042133134823));
#47300=CARTESIAN_POINT('Ctrl Pts',(26.9897086010189,3.56323667040224,15.5588142828321));
#47301=CARTESIAN_POINT('Ctrl Pts',(26.8507971105303,1.00484177718341,14.3954412174996));
#47302=CARTESIAN_POINT('Ctrl Pts',(26.7118856200417,-1.79836721821213,14.5975319073469));
#47303=CARTESIAN_POINT('Ctrl Pts',(26.572974129553,-4.16343195457351,16.1158500925799));
#47304=CARTESIAN_POINT('Ctrl Pts',(26.4340626390644,-5.51414111866785,18.580481114218));
#47305=CARTESIAN_POINT('Ctrl Pts',(26.2951511485758,-5.52141538794106,21.3909558790569));
#47306=CARTESIAN_POINT('Ctrl Pts',(26.1562396580872,-4.18348249959358,23.8625458339377));
#47307=CARTESIAN_POINT('Ctrl Pts',(26.0173281675984,-1.82630903490311,25.3930864495858));
#47308=CARTESIAN_POINT('Ctrl Pts',(25.8784166771098,0.975816278754277,25.6096852615627));
#47309=CARTESIAN_POINT('Ctrl Pts',(25.7395051866212,3.54019910240269,24.4595713313078));
#47310=CARTESIAN_POINT('Ctrl Pts',(25.6005936961325,5.24206736459369,22.2229520662257));
#47311=CARTESIAN_POINT('Ctrl Pts',(25.4616822056439,5.66678727910155,19.4447450341616));
#47312=CARTESIAN_POINT('Ctrl Pts',(25.3227707151553,4.71088243112365,16.8018172560334));
#47313=CARTESIAN_POINT('Ctrl Pts',(25.1838592246667,2.60724419961922,14.9380770622986));
#47314=CARTESIAN_POINT('Ctrl Pts',(25.044947734178,-0.131608612308295,14.3075958227792));
#47315=CARTESIAN_POINT('Ctrl Pts',(24.9060362436894,-2.83839702863386,15.0639805053548));
#47316=CARTESIAN_POINT('Ctrl Pts',(24.7671247532008,-4.85365406562751,17.0229497224782));
#47317=CARTESIAN_POINT('Ctrl Pts',(24.6282132627121,-5.68639362640362,19.7072310308935));
#47318=CARTESIAN_POINT('Ctrl Pts',(24.4893017722235,-5.13373164249729,22.4628409543649));
#47319=CARTESIAN_POINT('Ctrl Pts',(24.3503902817348,-3.33031562804408,24.6184179067382));
#47320=CARTESIAN_POINT('Ctrl Pts',(24.2114787912462,-0.715519902916424,
25.6487890217467));
#47321=CARTESIAN_POINT('Ctrl Pts',(24.0725673007576,2.07360114048475,25.3029203703106));
#47322=CARTESIAN_POINT('Ctrl Pts',(23.9336558102689,4.3575214517833,23.6650774808896));
#47323=CARTESIAN_POINT('Ctrl Pts',(23.7947443197803,5.57979929741503,21.1342953514151));
#47324=CARTESIAN_POINT('Ctrl Pts',(23.6558328292917,5.44264565209923,18.3271597657396));
#47325=CARTESIAN_POINT('Ctrl Pts',(23.516921338803,3.97947587266186,15.9275857378482));
#47326=CARTESIAN_POINT('Ctrl Pts',(23.3780098483144,1.54676856500752,14.520192234213));
#47327=CARTESIAN_POINT('Ctrl Pts',(23.2390983578257,-1.26278489506185,14.4478688368808));
#47328=CARTESIAN_POINT('Ctrl Pts',(23.1001868673371,-3.76468041599438,15.7282360190311));
#47329=CARTESIAN_POINT('Ctrl Pts',(22.9612753768485,-5.34936998774029,18.0493521901843));
#47330=CARTESIAN_POINT('Ctrl Pts',(22.8223638863598,-5.63076859319054,20.8457134228651));
#47331=CARTESIAN_POINT('Ctrl Pts',(22.6834523958712,-4.54031782990674,23.4360297069592));
#47332=CARTESIAN_POINT('Ctrl Pts',(22.5445409053826,-2.34368910073348,25.1892106859115));
#47333=CARTESIAN_POINT('Ctrl Pts',(22.4056294148939,0.423943099837686,25.6781210265171));
#47334=CARTESIAN_POINT('Ctrl Pts',(22.2667179244053,3.08828814444319,24.7836453129979));
#47335=CARTESIAN_POINT('Ctrl Pts',(22.1278064339167,5.0002197180801,22.7237086691859));
#47336=CARTESIAN_POINT('Ctrl Pts',(21.988894943428,5.69392536922479,20.0001826846651));
#47337=CARTESIAN_POINT('Ctrl Pts',(21.8499834529394,5.00039448345398,17.2766121918614));
#47338=CARTESIAN_POINT('Ctrl Pts',(21.7110719624507,3.08859509632026,15.2165528669524));
#47339=CARTESIAN_POINT('Ctrl Pts',(21.5721604719621,0.424307454157508,14.3219061888675));
#47340=CARTESIAN_POINT('Ctrl Pts',(21.4332489814735,-2.34335611324554,14.8106389343013));
#47341=CARTESIAN_POINT('Ctrl Pts',(21.2943374909848,-4.54009733648359,16.5636789557828));
#47342=CARTESIAN_POINT('Ctrl Pts',(21.1554260004962,-5.63071431363232,19.1539252622071));
#47343=CARTESIAN_POINT('Ctrl Pts',(21.0165145100076,-5.3494951464188,21.9503045459919));
#47344=CARTESIAN_POINT('Ctrl Pts',(20.8776030195189,-3.76495451994031,24.2715223991519));
#47345=CARTESIAN_POINT('Ctrl Pts',(20.7386915290303,-1.26314116310334,25.5520501209687));
#47346=CARTESIAN_POINT('Ctrl Pts',(20.5997800385416,1.54641693204892,25.4799070079654));
#47347=CARTESIAN_POINT('Ctrl Pts',(20.460868548053,3.97921454469859,24.0726696098425));
#47348=CARTESIAN_POINT('Ctrl Pts',(20.3219570575644,5.44253829763327,21.6731894759621));
#47349=CARTESIAN_POINT('Ctrl Pts',(20.1830455670758,5.57987207169572,18.8660626969777));
#47350=CARTESIAN_POINT('Ctrl Pts',(20.0441340765871,4.35775662448668,16.335202141261));
#47351=CARTESIAN_POINT('Ctrl Pts',(19.9052225860985,2.07394141543192,14.6972127000009));
#47352=CARTESIAN_POINT('Ctrl Pts',(19.7663110956099,-0.715157428434673,
14.35116507621));
#47353=CARTESIAN_POINT('Ctrl Pts',(19.6273996051212,-3.33001926530899,15.3813684021838));
#47354=CARTESIAN_POINT('Ctrl Pts',(19.4884881146326,-5.13357359568929,17.5368296280369));
#47355=CARTESIAN_POINT('Ctrl Pts',(19.3495766241439,-5.68641240117427,20.2924040824727));
#47356=CARTESIAN_POINT('Ctrl Pts',(19.2106651336553,-4.85384508779539,22.9767388208171));
#47357=CARTESIAN_POINT('Ctrl Pts',(19.0717536431667,-2.83871375861276,24.9358373494614));
#47358=CARTESIAN_POINT('Ctrl Pts',(18.932842152678,-0.131973883754986,25.6923957204047));
#47359=CARTESIAN_POINT('Ctrl Pts',(18.7939306621894,2.60691937942308,25.0620902296248));
#47360=CARTESIAN_POINT('Ctrl Pts',(18.6550191717008,4.71067719957706,23.1984850265493));
#47361=CARTESIAN_POINT('Ctrl Pts',(18.5161076812121,5.66675163768531,20.5556185926209));
#47362=CARTESIAN_POINT('Ctrl Pts',(18.3771961907235,5.24220999678571,17.7773843127353));
#47363=CARTESIAN_POINT('Ctrl Pts',(18.2382847002348,3.54048525808325,15.5406558463188));
#47364=CARTESIAN_POINT('Ctrl Pts',(18.0993732097462,0.97617624053337,14.3903773664271));
#47365=CARTESIAN_POINT('Ctrl Pts',(17.9604617192575,-1.82596296612573,14.6067963704295));
#47366=CARTESIAN_POINT('Ctrl Pts',(17.821550228769,-4.18323463810387,16.1371857271876));
#47367=CARTESIAN_POINT('Ctrl Pts',(17.6826387382803,-5.52132612134381,18.6086898241436));
#47368=CARTESIAN_POINT('Ctrl Pts',(17.5437272477917,-5.51423219538396,21.4191650499735));
#47369=CARTESIAN_POINT('Ctrl Pts',(17.404815757303,-4.16368118517472,23.8838827392053));
#47370=CARTESIAN_POINT('Ctrl Pts',(17.2659042668144,-1.79871388153097,25.4023526834207));
#47371=CARTESIAN_POINT('Ctrl Pts',(17.1269927763257,1.00448214028381,25.6046232499185));
#47372=CARTESIAN_POINT('Ctrl Pts',(16.9880812858371,3.5629516798703,24.4414143547506));
#47373=CARTESIAN_POINT('Ctrl Pts',(16.8491697953485,5.25336334565759,22.1961237902669));
#47374=CARTESIAN_POINT('Ctrl Pts',(16.7102583048598,5.66387457330821,19.4157817518188));
#47375=CARTESIAN_POINT('Ctrl Pts',(16.5713468143712,4.69447067402958,16.7777754214904));
#47376=CARTESIAN_POINT('Ctrl Pts',(16.4324353238826,2.58133186110226,14.9248140953721));
#47377=CARTESIAN_POINT('Ctrl Pts',(16.2935238333939,-0.160708393171607,
14.3083430394972));
#47378=CARTESIAN_POINT('Ctrl Pts',(16.1546123429053,-2.86359454191366,15.0785558579623));
#47379=CARTESIAN_POINT('Ctrl Pts',(16.0157008524166,-4.86881032832087,17.0478021525462));
#47380=CARTESIAN_POINT('Ctrl Pts',(15.876789361928,-5.68781605035605,19.7363056295874));
#47381=CARTESIAN_POINT('Ctrl Pts',(15.7378778714394,-5.12107367619125,22.4890541469997));
#47382=CARTESIAN_POINT('Ctrl Pts',(15.5989663809508,-3.30666118849705,24.6353832558012));
#47383=CARTESIAN_POINT('Ctrl Pts',(15.4600548904621,-0.686632027167408,
25.6523731832694));
#47384=CARTESIAN_POINT('Ctrl Pts',(15.3211433999735,2.10068436989794,25.2922501189704));
#47385=CARTESIAN_POINT('Ctrl Pts',(15.1822319094848,4.3762016263914,23.642752457805));
#47386=CARTESIAN_POINT('Ctrl Pts',(15.0433204189962,5.58552528262248,21.105754701939));
#47387=CARTESIAN_POINT('Ctrl Pts',(14.9044089285076,5.43402240048716,18.2993569761178));
#47388=CARTESIAN_POINT('Ctrl Pts',(14.7654974380189,3.95860430563815,15.9072945262262));
#47389=CARTESIAN_POINT('Ctrl Pts',(14.6265859475303,1.51873371591571,14.5123562393486));
#47390=CARTESIAN_POINT('Ctrl Pts',(14.4876744570417,-1.29115277038856,14.454397177295));
#47391=CARTESIAN_POINT('Ctrl Pts',(14.348762966553,-3.78646992504974,15.7475381659127));
#47392=CARTESIAN_POINT('Ctrl Pts',(14.2098514760644,-5.3592724548528,18.0767254750475));
#47393=CARTESIAN_POINT('Ctrl Pts',(14.0709399855757,-5.62637143595118,20.8744887697324));
#47394=CARTESIAN_POINT('Ctrl Pts',(13.9320284950871,-4.52269234742555,23.459196449208));
#47395=CARTESIAN_POINT('Ctrl Pts',(13.7931170045985,-2.31712946823991,25.2011246063798));
#47396=CARTESIAN_POINT('Ctrl Pts',(13.6542055141098,0.452966040136749,25.6758794834068));
#47397=CARTESIAN_POINT('Ctrl Pts',(13.5152940236212,3.11270340362871,24.7677944234954));
#47398=CARTESIAN_POINT('Ctrl Pts',(13.3763825331326,5.01407889721741,22.6981102564859));
#47399=CARTESIAN_POINT('Ctrl Pts',(13.2374710426439,5.69385189443484,19.9710734046917));
#47400=CARTESIAN_POINT('Ctrl Pts',(13.0985595521553,4.9864062557289,17.251084068855));
#47401=CARTESIAN_POINT('Ctrl Pts',(12.9596480616667,3.06410013022447,15.2008254318442));
#47402=CARTESIAN_POINT('Ctrl Pts',(12.820736571178,0.395273567977247,14.3198111871053));
#47403=CARTESIAN_POINT('Ctrl Pts',(12.6818250806894,-2.36985526379726,14.8226867805465));
#47404=CARTESIAN_POINT('Ctrl Pts',(12.5429135902007,-4.55760564468624,16.5869343793007));
#47405=CARTESIAN_POINT('Ctrl Pts',(12.4040020997121,-5.63496615195067,19.1827224400208));
#47406=CARTESIAN_POINT('Ctrl Pts',(12.2650906092235,-5.33945462044222,21.9776274927077));
#47407=CARTESIAN_POINT('Ctrl Pts',(12.1261791187348,-3.74306784797717,24.2907143029005));
#47408=CARTESIAN_POINT('Ctrl Pts',(11.9872676282462,-1.23474069305955,25.5584351722925));
#47409=CARTESIAN_POINT('Ctrl Pts',(11.8483561377576,1.57441186647029,25.4719295882159));
#47410=CARTESIAN_POINT('Ctrl Pts',(11.7094446472689,3.9999834122542,24.0522732935189));
#47411=CARTESIAN_POINT('Ctrl Pts',(11.5705331567803,5.45102108611097,21.6453435089515));
#47412=CARTESIAN_POINT('Ctrl Pts',(11.4316216662917,5.57400208135005,18.8375513169259));
#47413=CARTESIAN_POINT('Ctrl Pts',(11.292710175803,4.33896398735324,16.3129717033732));
#47414=CARTESIAN_POINT('Ctrl Pts',(11.1537986853144,2.04680466585494,14.6866793054146));
#47415=CARTESIAN_POINT('Ctrl Pts',(11.0148871948257,-0.744026842628766,
14.3548950230201));
#47416=CARTESIAN_POINT('Ctrl Pts',(10.8759757043371,-3.35358775945367,15.3984529467452));
#47417=CARTESIAN_POINT('Ctrl Pts',(10.7370642138485,-5.14609907200881,17.563106386248));
#47418=CARTESIAN_POINT('Ctrl Pts',(10.5981527233598,-5.68484322177988,20.3214711300549));
#47419=CARTESIAN_POINT('Ctrl Pts',(10.4592412328712,-4.83856355889019,23.0015144227965));
#47420=CARTESIAN_POINT('Ctrl Pts',(10.3203297423826,-2.81344298751949,24.9502853149745));
#47421=CARTESIAN_POINT('Ctrl Pts',(10.1814182518939,-0.10287070160567,25.6929960269112));
#47422=CARTESIAN_POINT('Ctrl Pts',(10.0425067614053,2.6327644340281,25.0486966217621));
#47423=CARTESIAN_POINT('Ctrl Pts',(9.90359527091664,4.72696738024193,23.1743606489817));
#47424=CARTESIAN_POINT('Ctrl Pts',(9.76468378042803,5.66951809474209,20.526640975492));
#47425=CARTESIAN_POINT('Ctrl Pts',(9.62577228993937,5.23077872591258,17.7506134026771));
#47426=CARTESIAN_POINT('Ctrl Pts',(9.48686079945075,3.51764131099587,15.5226139600376));
#47427=CARTESIAN_POINT('Ctrl Pts',(9.3479493089621,0.947485190363111,14.3854601294747));
#47428=CARTESIAN_POINT('Ctrl Pts',(9.20903781847346,-1.85351099033822,14.6162017912657));
#47429=CARTESIAN_POINT('Ctrl Pts',(9.07012632798483,-4.20292798785086,16.1586223210136));
#47430=CARTESIAN_POINT('Ctrl Pts',(8.93121483749619,-5.52836681763337,18.6369348976056));
#47431=CARTESIAN_POINT('Ctrl Pts',(8.79230334700757,-5.50690488184858,21.4473371293336));
#47432=CARTESIAN_POINT('Ctrl Pts',(8.6533918565189,-4.14377104802507,23.9051181346055));
#47433=CARTESIAN_POINT('Ctrl Pts',(8.51448036603029,-1.77107171664475,25.4114777203806));
#47434=CARTESIAN_POINT('Ctrl Pts',(8.37556887554165,1.03312174848493,25.5994147548189));
#47435=CARTESIAN_POINT('Ctrl Pts',(8.23665738505302,3.58561113538302,24.4231412965778));
#47436=CARTESIAN_POINT('Ctrl Pts',(8.09774589456438,5.2645220238591,22.1692381160162));
#47437=CARTESIAN_POINT('Ctrl Pts',(7.95883440407574,5.66081383545613,19.3868337387104));
#47438=CARTESIAN_POINT('Ctrl Pts',(7.8199229135871,4.6779362213937,16.7538178035964));
#47439=CARTESIAN_POINT('Ctrl Pts',(7.68101142309847,2.55535205642491,14.9116837744299));
#47440=CARTESIAN_POINT('Ctrl Pts',(7.54209993260983,-0.189803973731052,
14.3092390143996));
#47441=CARTESIAN_POINT('Ctrl Pts',(7.40318844212119,-2.88871721176426,15.0932598383313));
#47442=CARTESIAN_POINT('Ctrl Pts',(7.26427695163256,-4.88383933889966,17.0727317417955));
#47443=CARTESIAN_POINT('Ctrl Pts',(7.12536546114392,-5.68908981651096,19.7653871202457));
#47444=CARTESIAN_POINT('Ctrl Pts',(6.98645397065528,-5.10828186456958,22.5152022852615));
#47445=CARTESIAN_POINT('Ctrl Pts',(6.84754248016665,-3.28292032545007,24.6522274536422));
#47446=CARTESIAN_POINT('Ctrl Pts',(6.70863098967801,-0.657726205478431,
25.6558096133358));
#47447=CARTESIAN_POINT('Ctrl Pts',(6.56971949918938,2.12771269544141,25.2814415484158));
#47448=CARTESIAN_POINT('Ctrl Pts',(6.43080800870074,4.39476742379579,23.6203322270779));
#47449=CARTESIAN_POINT('Ctrl Pts',(6.29189651821209,5.5911052835226,21.0771851522562));
#47450=CARTESIAN_POINT('Ctrl Pts',(6.15298502772346,5.42525712427457,18.2715986348122));
#47451=CARTESIAN_POINT('Ctrl Pts',(6.01407353723483,3.93762927581034,15.8871102823007));
#47452=CARTESIAN_POINT('Ctrl Pts',(5.87516204674619,1.4906591729225,14.5046636705423));
#47453=CARTESIAN_POINT('Ctrl Pts',(5.73625055625756,-1.31948689991102,14.4610704585959));
#47454=CARTESIAN_POINT('Ctrl Pts',(5.59733906576892,-3.80816047023665,15.7669514559124));
#47455=CARTESIAN_POINT('Ctrl Pts',(5.45842757528029,-5.36903485104308,18.1041490269644));
#47456=CARTESIAN_POINT('Ctrl Pts',(5.31951608479166,-5.6218272268419,20.9032412608016));
#47457=CARTESIAN_POINT('Ctrl Pts',(5.18060459430301,-4.50494865903241,23.4822727812676));
#47458=CARTESIAN_POINT('Ctrl Pts',(5.04169310381438,-2.29050927482802,25.2129025893069));
#47459=CARTESIAN_POINT('Ctrl Pts',(4.90278161332574,0.481977141632756,25.6734895944752));
#47460=CARTESIAN_POINT('Ctrl Pts',(4.7638701228371,3.1370373086304,24.7518189220483));
#47461=CARTESIAN_POINT('Ctrl Pts',(4.62495863234846,5.0278070274742,22.6724413254842));
#47462=CARTESIAN_POINT('Ctrl Pts',(4.48604714185984,5.69362960409341,19.9419648807492));
#47463=CARTESIAN_POINT('Ctrl Pts',(4.34713565137119,4.97228770238059,17.2256277920167));
#47464=CARTESIAN_POINT('Ctrl Pts',(4.20822416088256,3.03952508024898,15.1852234288378));
#47465=CARTESIAN_POINT('Ctrl Pts',(4.06931267039391,0.366229350854573,14.3178646437937));
#47466=CARTESIAN_POINT('Ctrl Pts',(3.93040117990528,-2.39629247537946,14.8348699419947));
#47467=CARTESIAN_POINT('Ctrl Pts',(3.79148968941664,-4.57499483447723,16.6102790073235));
#47468=CARTESIAN_POINT('Ctrl Pts',(3.65257819892802,-5.63907071376474,19.2115409783509));
#47469=CARTESIAN_POINT('Ctrl Pts',(3.51366670843937,-5.3292745415085,22.004898751788));
#47470=CARTESIAN_POINT('Ctrl Pts',(3.37475521795074,-3.72108334650527,24.3097940637625));
#47471=CARTESIAN_POINT('Ctrl Pts',(3.23584372746209,-1.20630795161736,25.5646749473313));
#47472=CARTESIAN_POINT('Ctrl Pts',(3.09693223697347,1.60236565179515,25.4638091531359));
#47473=CARTESIAN_POINT('Ctrl Pts',(2.95802074648483,4.02064773547646,24.0317710662039));
#47474=CARTESIAN_POINT('Ctrl Pts',(2.8191092559962,5.45936140578133,21.6174545390167));
#47475=CARTESIAN_POINT('Ctrl Pts',(2.68019776550755,5.56798640772404,18.8090703186992));
#47476=CARTESIAN_POINT('Ctrl Pts',(2.54128627501892,4.32005794655219,16.2908376306162));
#47477=CARTESIAN_POINT('Ctrl Pts',(2.40237478453028,2.01961442005369,14.6762847801816));
#47478=CARTESIAN_POINT('Ctrl Pts',(2.26346329404165,-0.772876809690231,
14.3587725124367));
#47479=CARTESIAN_POINT('Ctrl Pts',(2.12455180355301,-3.37706860580615,15.4156577559866));
#47480=CARTESIAN_POINT('Ctrl Pts',(1.98564031306437,-5.15849004463263,17.5894468398745));
#47481=CARTESIAN_POINT('Ctrl Pts',(1.84672882257574,-5.68312547077942,20.3505297671009));
#47482=CARTESIAN_POINT('Ctrl Pts',(1.7078173320871,-4.82315555167649,23.0262115934059));
#47483=CARTESIAN_POINT('Ctrl Pts',(1.56890584159846,-2.78809871671838,24.9646038659185));
#47484=CARTESIAN_POINT('Ctrl Pts',(1.42999435110983,-0.0737647659051136,
25.693447605254));
#47485=CARTESIAN_POINT('Ctrl Pts',(1.29108286062119,2.65854055037997,25.035170932176));
#47486=CARTESIAN_POINT('Ctrl Pts',(1.15217137013255,4.74313426783574,23.1501535580012));
#47487=CARTESIAN_POINT('Ctrl Pts',(1.01325987964391,5.6721358762478,20.497649097109));
#47488=CARTESIAN_POINT('Ctrl Pts',(0.874348389155275,5.21921171941123,17.7239022616837));
#47489=CARTESIAN_POINT('Ctrl Pts',(0.735436898666642,3.49470350187287,15.5046871678098));
#47490=CARTESIAN_POINT('Ctrl Pts',(0.596525408178007,0.918773166897274,
14.3806934322185));
#47491=CARTESIAN_POINT('Ctrl Pts',(0.457613917689371,-1.88101803678174,
14.625740444846));
#47492=CARTESIAN_POINT('Ctrl Pts',(0.318702427200727,-4.2224967827303,16.1801740467554));
#47493=CARTESIAN_POINT('Ctrl Pts',(0.179790936712099,-5.53529199863674,
18.6651865633432));
#47494=CARTESIAN_POINT('Ctrl Pts',(0.0408794462234612,-5.49937647599996,
21.4755287212687));
#47495=CARTESIAN_POINT('Ctrl Pts',(-0.098032044265173,-4.12386623843618,
23.9261367566677));
#47496=CARTESIAN_POINT('Ctrl Pts',(-0.236943534753806,-1.74314764379901,
25.4207072293527));
#47497=CARTESIAN_POINT('Ctrl Pts',(-0.329551195079564,0.12636836631501,
25.5357780776651));
#47498=CARTESIAN_POINT('Ctrl Pts',(-0.375855025242444,1.01853433275011,
25.3664478824926));
#47499=CARTESIAN_POINT('Ctrl Pts',(50.3758550252424,4.37166823191287,23.7929628171897));
#47500=CARTESIAN_POINT('Ctrl Pts',(50.3295511950796,5.00224406373827,23.066177856549));
#47501=CARTESIAN_POINT('Ctrl Pts',(50.2369435347538,5.89327567631712,21.2927683877858));
#47502=CARTESIAN_POINT('Ctrl Pts',(50.0980320442652,5.79343898530443,18.3159622522944));
#47503=CARTESIAN_POINT('Ctrl Pts',(49.9591205537765,4.2823206076606,15.7501656734355));
#47504=CARTESIAN_POINT('Ctrl Pts',(49.8202090632879,1.72778693233764,14.2194224359483));
#47505=CARTESIAN_POINT('Ctrl Pts',(49.6812975727993,-1.247647937075,14.097205211392));
#47506=CARTESIAN_POINT('Ctrl Pts',(49.5423860823106,-3.91913669798948,15.4130220371016));
#47507=CARTESIAN_POINT('Ctrl Pts',(49.403474591822,-5.63577648176899,17.8464306709765));
#47508=CARTESIAN_POINT('Ctrl Pts',(49.2645631013334,-5.97935297166014,20.8044997806298));
#47509=CARTESIAN_POINT('Ctrl Pts',(49.1256516108447,-4.86614978762969,23.5665768168738));
#47510=CARTESIAN_POINT('Ctrl Pts',(48.9867401203561,-2.56738632874741,25.4597067746574));
#47511=CARTESIAN_POINT('Ctrl Pts',(48.8478286298675,0.356881766247415,26.0226669648869));
#47512=CARTESIAN_POINT('Ctrl Pts',(48.7089171393788,3.19420074846009,25.1182962854986));
#47513=CARTESIAN_POINT('Ctrl Pts',(48.5700056488902,5.25330250574948,22.9669329453697));
#47514=CARTESIAN_POINT('Ctrl Pts',(48.4310941584015,6.03251854196515,20.0927220465274));
#47515=CARTESIAN_POINT('Ctrl Pts',(48.2921826679129,5.34200512389304,17.1959210624955));
#47516=CARTESIAN_POINT('Ctrl Pts',(48.1532711774242,3.34999504705893,14.9822902848886));
#47517=CARTESIAN_POINT('Ctrl Pts',(48.0143596869356,0.541810688388326,13.991146648205));
#47518=CARTESIAN_POINT('Ctrl Pts',(47.8754481964469,-2.39837744171306,14.4639668367131));
#47519=CARTESIAN_POINT('Ctrl Pts',(47.7365367059584,-4.75423813142894,16.2855555903485));
#47520=CARTESIAN_POINT('Ctrl Pts',(47.5976252154697,-5.95180249600114,19.012111063151));
#47521=CARTESIAN_POINT('Ctrl Pts',(47.4587137249811,-5.69930256348713,21.9793503451825));
#47522=CARTESIAN_POINT('Ctrl Pts',(47.3198022344924,-4.05825602460495,24.4643516366976));
#47523=CARTESIAN_POINT('Ctrl Pts',(47.1808907440038,-1.42847839604861,25.8616829470684));
#47524=CARTESIAN_POINT('Ctrl Pts',(47.0419792535151,1.54932582119811,25.8309061901086));
#47525=CARTESIAN_POINT('Ctrl Pts',(46.9030677630265,4.14966085031285,24.3795196456277));
#47526=CARTESIAN_POINT('Ctrl Pts',(46.7641562725379,5.73899542293203,21.861131116882));
#47527=CARTESIAN_POINT('Ctrl Pts',(46.6252447820492,5.93011283962871,18.8893068794517));
#47528=CARTESIAN_POINT('Ctrl Pts',(46.4863332915607,4.67645030826474,16.1880857809881));
#47529=CARTESIAN_POINT('Ctrl Pts',(46.347421801072,2.28344324566841,14.4155784146835));
#47530=CARTESIAN_POINT('Ctrl Pts',(46.2085103105834,-0.665889320858256,
14.0036286880202));
#47531=CARTESIAN_POINT('Ctrl Pts',(46.0695988200947,-3.45298829007873,15.052601757759));
#47532=CARTESIAN_POINT('Ctrl Pts',(45.9306873296061,-5.39882025860657,17.3069316172779));
#47533=CARTESIAN_POINT('Ctrl Pts',(45.7917758391174,-6.02931346989326,20.2173857872984));
#47534=CARTESIAN_POINT('Ctrl Pts',(45.6528643486288,-5.19085803932404,23.074877284436));
#47535=CARTESIAN_POINT('Ctrl Pts',(45.5139528581402,-3.08773061831874,25.183222658487));
#47536=CARTESIAN_POINT('Ctrl Pts',(45.3750413676515,-0.232325558931368,
26.0287562841288));
#47537=CARTESIAN_POINT('Ctrl Pts',(45.2361298771629,2.67968201680631,25.4054770175777));
#47538=CARTESIAN_POINT('Ctrl Pts',(45.0972183866742,4.93882666231995,23.4652371777865));
#47539=CARTESIAN_POINT('Ctrl Pts',(44.9583068961857,5.99470285045386,20.6807460859354));
#47540=CARTESIAN_POINT('Ctrl Pts',(44.819395405697,5.59006273694311,17.7304017765701));
#47541=CARTESIAN_POINT('Ctrl Pts',(44.6804839152084,3.82349060474963,15.3330098463627));
#47542=CARTESIAN_POINT('Ctrl Pts',(44.5415724247197,1.12538433371236,14.0726576275543));
#47543=CARTESIAN_POINT('Ctrl Pts',(44.4026609342311,-1.84690436237671,14.2564103754716));
#47544=CARTESIAN_POINT('Ctrl Pts',(44.2637494437424,-4.36922347763402,15.8394995852365));
#47545=CARTESIAN_POINT('Ctrl Pts',(44.1248379532538,-5.82704911026108,18.436230143096));
#47546=CARTESIAN_POINT('Ctrl Pts',(43.9859264627652,-5.86520467277351,21.4139489542525));
#47547=CARTESIAN_POINT('Ctrl Pts',(43.8470149722765,-4.47439415460361,24.0471810495708));
#47548=CARTESIAN_POINT('Ctrl Pts',(43.7081034817879,-1.99346695078559,25.6943803012164));
#47549=CARTESIAN_POINT('Ctrl Pts',(43.5691919912993,0.973137533632203,25.9542321788281));
#47550=CARTESIAN_POINT('Ctrl Pts',(43.4302805008106,3.70265216271139,24.7634278057639));
#47551=CARTESIAN_POINT('Ctrl Pts',(43.291369010322,5.53007306373358,22.4120881842347));
#47552=CARTESIAN_POINT('Ctrl Pts',(43.1524575198334,6.01017749880994,19.4730807162811));
#47553=CARTESIAN_POINT('Ctrl Pts',(43.0135460293447,5.02599547436225,16.6624489531326));
#47554=CARTESIAN_POINT('Ctrl Pts',(42.8746345388561,2.81730766448726,14.6649596981487));
#47555=CARTESIAN_POINT('Ctrl Pts',(42.7357230483674,-0.0777734284877525,
13.9672702039146));
#47556=CARTESIAN_POINT('Ctrl Pts',(42.5968115578788,-2.95390623278611,14.739361686386));
#47557=CARTESIAN_POINT('Ctrl Pts',(42.4579000673901,-5.11036563305792,16.7931260400171));
#47558=CARTESIAN_POINT('Ctrl Pts',(42.3189885769016,-6.02176376830294,19.6281954579217));
#47559=CARTESIAN_POINT('Ctrl Pts',(42.1800770864129,-5.46605262930032,22.553849281472));
#47560=CARTESIAN_POINT('Ctrl Pts',(42.0411655959243,-3.57862260949675,24.8572973676269));
#47561=CARTESIAN_POINT('Ctrl Pts',(41.9022541054356,-0.819316737129712,
25.9773403435821));
#47562=CARTESIAN_POINT('Ctrl Pts',(41.763342614947,2.13960294106554,25.6410971231969));
#47563=CARTESIAN_POINT('Ctrl Pts',(41.6244311244583,4.57724157290559,23.9304881480575));
#47564=CARTESIAN_POINT('Ctrl Pts',(41.4855196339698,5.8997063419931,21.2622767434293));
#47565=CARTESIAN_POINT('Ctrl Pts',(41.346608143481,5.78479923421689,18.286531202922));
#47566=CARTESIAN_POINT('Ctrl Pts',(41.2076966529925,4.26051558283505,15.7282457389059));
#47567=CARTESIAN_POINT('Ctrl Pts',(41.0687851625038,1.69822344006145,14.2107068957962));
#47568=CARTESIAN_POINT('Ctrl Pts',(40.9298736720152,-1.27781448459974,14.103639457962));
#47569=CARTESIAN_POINT('Ctrl Pts',(40.7909621815266,-3.94253274391769,15.4331287447649));
#47570=CARTESIAN_POINT('Ctrl Pts',(40.6520506910379,-5.6467140949177,17.8752653273847));
#47571=CARTESIAN_POINT('Ctrl Pts',(40.5131392005493,-5.97516120318881,20.8350605335323));
#47572=CARTESIAN_POINT('Ctrl Pts',(40.3742277100606,-4.84785302885217,23.5914062022284));
#47573=CARTESIAN_POINT('Ctrl Pts',(40.235316219572,-2.53944071086646,25.4727614944149));
#47574=CARTESIAN_POINT('Ctrl Pts',(40.0964047290833,0.387666919931939,26.020763394948));
#47575=CARTESIAN_POINT('Ctrl Pts',(39.9574932385947,3.22032552293136,25.1018997466741));
#47576=CARTESIAN_POINT('Ctrl Pts',(39.8185817481061,5.26840179713572,22.9400374151859));
#47577=CARTESIAN_POINT('Ctrl Pts',(39.6796702576175,6.03291374792276,20.0618806018121));
#47578=CARTESIAN_POINT('Ctrl Pts',(39.5407587671288,5.32759990499422,17.1686475402978));
#47579=CARTESIAN_POINT('Ctrl Pts',(39.4018472766402,3.32429903852281,14.9652295582388));
#47580=CARTESIAN_POINT('Ctrl Pts',(39.2629357861515,0.511084310026281,13.9884552462116));
#47581=CARTESIAN_POINT('Ctrl Pts',(39.1240242956629,-2.42664817772029,14.4763005041618));
#47582=CARTESIAN_POINT('Ctrl Pts',(38.9851128051743,-4.77316550262547,16.3099094071687));
#47583=CARTESIAN_POINT('Ctrl Pts',(38.8462013146856,-5.95677514037071,19.0425516067079));
#47584=CARTESIAN_POINT('Ctrl Pts',(38.707289824197,-5.68910897433122,22.0084612460638));
#47585=CARTESIAN_POINT('Ctrl Pts',(38.5683783337084,-4.03537971123355,24.4850404775119));
#47586=CARTESIAN_POINT('Ctrl Pts',(38.4294668432197,-1.39849281737248,25.8689092119843));
#47587=CARTESIAN_POINT('Ctrl Pts',(38.2905553527311,1.57911514448126,25.8229093122962));
#47588=CARTESIAN_POINT('Ctrl Pts',(38.1516438622424,4.17199621190449,24.3582479400111));
#47589=CARTESIAN_POINT('Ctrl Pts',(38.0127323717538,5.7484351586937,21.8317671044787));
#47590=CARTESIAN_POINT('Ctrl Pts',(37.8738208812651,5.92435710444692,18.8590046460457));
#47591=CARTESIAN_POINT('Ctrl Pts',(37.7349093907765,4.6569013976858,16.1642279954371));
#47592=CARTESIAN_POINT('Ctrl Pts',(37.5959979002879,2.25486394831888,14.4039776561089));
#47593=CARTESIAN_POINT('Ctrl Pts',(37.4570864097993,-0.696536102775852,
14.0071113011932));
#47594=CARTESIAN_POINT('Ctrl Pts',(37.3181749193106,-3.47823594384081,15.070319258032));
#47595=CARTESIAN_POINT('Ctrl Pts',(37.179263428822,-5.41251758525951,17.3345674107169));
#47596=CARTESIAN_POINT('Ctrl Pts',(37.0403519383333,-6.0281233284039,20.2482068417848));
#47597=CARTESIAN_POINT('Ctrl Pts',(36.9014404478447,-5.17507038919311,23.1013745284394));
#47598=CARTESIAN_POINT('Ctrl Pts',(36.7625289573561,-3.06119187544985,25.1989404497874));
#47599=CARTESIAN_POINT('Ctrl Pts',(36.6236174668674,-0.20150147609856,26.0298652268426));
#47600=CARTESIAN_POINT('Ctrl Pts',(36.4847059763788,2.7072816302624,25.3917069350253));
#47601=CARTESIAN_POINT('Ctrl Pts',(36.3457944858901,4.95647758897316,23.4399429368469));
#47602=CARTESIAN_POINT('Ctrl Pts',(36.2068829954015,5.99810471599718,20.6500902358045));
#47603=CARTESIAN_POINT('Ctrl Pts',(36.0679715049129,5.57838672963962,17.7018531393018));
#47604=CARTESIAN_POINT('Ctrl Pts',(35.9290600144242,3.79958140254752,15.3135238543047));
#47605=CARTESIAN_POINT('Ctrl Pts',(35.7901485239356,1.09506704261718,14.0669817402161));
#47606=CARTESIAN_POINT('Ctrl Pts',(35.651237033447,-1.87624340496498,14.2659274347039));
#47607=CARTESIAN_POINT('Ctrl Pts',(35.5123255429584,-4.39043626938002,15.861890907278));
#47608=CARTESIAN_POINT('Ctrl Pts',(35.3734140524697,-5.83496748371407,18.4660404298824));
#47609=CARTESIAN_POINT('Ctrl Pts',(35.2345025619811,-5.85789943914815,21.443915392114));
#47610=CARTESIAN_POINT('Ctrl Pts',(35.0955910714924,-4.45364512068325,24.0700027810519));
#47611=CARTESIAN_POINT('Ctrl Pts',(34.9566795810038,-1.96432929662502,25.7044971656735));
#47612=CARTESIAN_POINT('Ctrl Pts',(34.8177680905152,1.00356487086217,25.9491793592669));
#47613=CARTESIAN_POINT('Ctrl Pts',(34.6788566000265,3.7269560345781,24.7444363432422));
#47614=CARTESIAN_POINT('Ctrl Pts',(34.5399451095379,5.54233220909366,22.3837850538165));
#47615=CARTESIAN_POINT('Ctrl Pts',(34.4010336190493,6.00740516717897,19.4423615363808));
#47616=CARTESIAN_POINT('Ctrl Pts',(34.2621221285606,5.00886710131083,16.6367979751193));
#47617=CARTESIAN_POINT('Ctrl Pts',(34.123210638072,2.78999631224823,14.6506263846692));
#47618=CARTESIAN_POINT('Ctrl Pts',(33.9842991475834,-0.10861377285947,13.967746644321));
#47619=CARTESIAN_POINT('Ctrl Pts',(33.8453876570947,-2.98076179807835,14.7545318033685));
#47620=CARTESIAN_POINT('Ctrl Pts',(33.706476166606,-5.12669347763074,16.8192938700385));
#47621=CARTESIAN_POINT('Ctrl Pts',(33.5675646761175,-6.0235858662618,19.6589856153662));
#47622=CARTESIAN_POINT('Ctrl Pts',(33.4286531856287,-5.45292505475955,22.5817602223931));
#47623=CARTESIAN_POINT('Ctrl Pts',(33.2897416951402,-3.55374369223119,24.875529024494));
#47624=CARTESIAN_POINT('Ctrl Pts',(33.1508302046515,-0.788747839168509,
25.9814508561855));
#47625=CARTESIAN_POINT('Ctrl Pts',(33.0119187141629,2.16841418221486,25.6300850289428));
#47626=CARTESIAN_POINT('Ctrl Pts',(32.8730072236743,4.59727574553591,23.9070363727848));
#47627=CARTESIAN_POINT('Ctrl Pts',(32.7340957331856,5.90608243090708,21.232098948172));
#47628=CARTESIAN_POINT('Ctrl Pts',(32.595184242697,5.77596380431826,18.2569797390846));
#47629=CARTESIAN_POINT('Ctrl Pts',(32.4562727522083,4.23862124947789,15.7065203619639));
#47630=CARTESIAN_POINT('Ctrl Pts',(32.3173612617197,1.66860441773134,14.2021006566271));
#47631=CARTESIAN_POINT('Ctrl Pts',(32.1784497712311,-1.3079419808491,14.1102491331561));
#47632=CARTESIAN_POINT('Ctrl Pts',(32.0395382807424,-3.96582861725453,15.4533439895544));
#47633=CARTESIAN_POINT('Ctrl Pts',(31.9006267902538,-5.65750266739463,17.9041610111513));
#47634=CARTESIAN_POINT('Ctrl Pts',(31.7617152997651,-5.97081400657861,20.8655966714357));
#47635=CARTESIAN_POINT('Ctrl Pts',(31.6228038092766,-4.82942919013311,23.6161431382409));
#47636=CARTESIAN_POINT('Ctrl Pts',(31.4838923187878,-2.51142891237346,25.4856724580356));
#47637=CARTESIAN_POINT('Ctrl Pts',(31.3449808282993,0.418442038286222,26.0187028302909));
#47638=CARTESIAN_POINT('Ctrl Pts',(31.2060693378106,3.24636608124152,25.0853696783341));
#47639=CARTESIAN_POINT('Ctrl Pts',(31.067157847322,5.28336341756275,22.9130651377399));
#47640=CARTESIAN_POINT('Ctrl Pts',(30.9282463568333,6.03315126387911,20.0310374920047));
#47641=CARTESIAN_POINT('Ctrl Pts',(30.7893348663447,5.31305544940377,17.1414480430965));
#47642=CARTESIAN_POINT('Ctrl Pts',(30.650423375856,3.29851614223578,14.9483004089548));
#47643=CARTESIAN_POINT('Ctrl Pts',(30.5115118853675,0.480344575529053,13.9859209692991));
#47644=CARTESIAN_POINT('Ctrl Pts',(30.3726003948788,-2.45485549124979,14.4887785368544));
#47645=CARTESIAN_POINT('Ctrl Pts',(30.2336889043902,-4.79196812107072,16.3343596704807));
#47646=CARTESIAN_POINT('Ctrl Pts',(30.0947774139015,-5.96159209759578,19.0730171734927));
#47647=CARTESIAN_POINT('Ctrl Pts',(29.9558659234129,-5.67876669347553,22.037519653851));
#47648=CARTESIAN_POINT('Ctrl Pts',(29.8169544329242,-4.01239792849797,24.5056120962796));
#47649=CARTESIAN_POINT('Ctrl Pts',(29.6780429424356,-1.36847068740464,25.8759820861257));
#47650=CARTESIAN_POINT('Ctrl Pts',(29.539131451947,1.60886319570866,25.8147602458098));
#47651=CARTESIAN_POINT('Ctrl Pts',(29.4002199614584,4.19422253344966,24.336862326459));
#47652=CARTESIAN_POINT('Ctrl Pts',(29.2613084709697,5.75772465230203,21.8023552166622));
#47653=CARTESIAN_POINT('Ctrl Pts',(29.1223969804811,5.91844652918931,18.8287322339093));
#47654=CARTESIAN_POINT('Ctrl Pts',(28.9834854899924,4.63723077348171,16.1404704623192));
#47655=CARTESIAN_POINT('Ctrl Pts',(28.8445739995038,2.22622571743447,14.3925231561968));
#47656=CARTESIAN_POINT('Ctrl Pts',(28.7056625090152,-0.72716467989911,14.0107505455973));
#47657=CARTESIAN_POINT('Ctrl Pts',(28.5667510185265,-3.50339268979386,15.0881656013405));
#47658=CARTESIAN_POINT('Ctrl Pts',(28.4278395280379,-5.42607344936586,17.3622728683879));
#47659=CARTESIAN_POINT('Ctrl Pts',(28.2889280375493,-6.02677563478385,20.279021409092));
#47660=CARTESIAN_POINT('Ctrl Pts',(28.1500165470606,-5.15914748247874,23.1277907143524));
#47661=CARTESIAN_POINT('Ctrl Pts',(28.011105056572,-3.03457312471181,25.2145223606322));
#47662=CARTESIAN_POINT('Ctrl Pts',(27.8721935660833,-0.170672126786414,
26.0308165718992));
#47663=CARTESIAN_POINT('Ctrl Pts',(27.7332820755947,2.73481048571209,25.3777959338371));
#47664=CARTESIAN_POINT('Ctrl Pts',(27.5943705851061,4.97399897222422,23.4145587889313));
#47665=CARTESIAN_POINT('Ctrl Pts',(27.4554590946174,6.00134981398182,20.6194173947965));
#47666=CARTESIAN_POINT('Ctrl Pts',(27.3165476041288,5.5665649246032,17.673364566819));
#47667=CARTESIAN_POINT('Ctrl Pts',(27.1776361136402,3.77557289379296,15.2941603488419));
#47668=CARTESIAN_POINT('Ctrl Pts',(27.0387246231515,1.06472113065006,14.0614609193251));
#47669=CARTESIAN_POINT('Ctrl Pts',(26.8998131326629,-1.90553340971345,14.2755943607024));
#47670=CARTESIAN_POINT('Ctrl Pts',(26.7609016421742,-4.41153431188298,15.8843903836934));
#47671=CARTESIAN_POINT('Ctrl Pts',(26.6219901516856,-5.84273335339281,18.4958908085158));
#47672=CARTESIAN_POINT('Ctrl Pts',(26.483078661197,-5.85044110239477,21.4738440915395));
#47673=CARTESIAN_POINT('Ctrl Pts',(26.3441671707084,-4.43277968548176,24.0927181381982));
#47674=CARTESIAN_POINT('Ctrl Pts',(26.2052556802197,-1.93514030239562,25.7144649363523));
#47675=CARTESIAN_POINT('Ctrl Pts',(26.0663441897311,1.03396597873771,25.943971050869));
#47676=CARTESIAN_POINT('Ctrl Pts',(25.9274326992424,3.75116249804223,24.7253208792671));
#47677=CARTESIAN_POINT('Ctrl Pts',(25.7885212087538,5.5544464990484,22.3554196203575));
#47678=CARTESIAN_POINT('Ctrl Pts',(25.6496097182652,6.00447582491098,19.4116569310209));
#47679=CARTESIAN_POINT('Ctrl Pts',(25.5106982277765,4.99160781559538,16.6112348983674));
#47680=CARTESIAN_POINT('Ctrl Pts',(25.3717867372879,2.76261204015674,14.636432883394));
#47681=CARTESIAN_POINT('Ctrl Pts',(25.2328752467992,-0.13945127848183,13.9683807448011));
#47682=CARTESIAN_POINT('Ctrl Pts',(25.0939637563106,-3.00753945763662,14.7698390168643));
#47683=CARTESIAN_POINT('Ctrl Pts',(24.955052265822,-5.1428873300079,16.8455448315755));
#47684=CARTESIAN_POINT('Ctrl Pts',(24.8161407753333,-6.02525053068195,19.6897846856248));
#47685=CARTESIAN_POINT('Ctrl Pts',(24.6772292848447,-5.43965496157513,22.6096036859583));
#47686=CARTESIAN_POINT('Ctrl Pts',(24.538317794356,-3.5287718936724,24.8936332536454));
#47687=CARTESIAN_POINT('Ctrl Pts',(24.3994063038674,-0.758158326349866,
25.9854050364986));
#47688=CARTESIAN_POINT('Ctrl Pts',(24.2604948133788,2.19716874929574,25.6189257857596));
#47689=CARTESIAN_POINT('Ctrl Pts',(24.1215833228901,4.61718976292897,23.8834824824969));
#47690=CARTESIAN_POINT('Ctrl Pts',(23.9826718324015,5.91230415737359,21.201888950552));
#47691=CARTESIAN_POINT('Ctrl Pts',(23.8437603419129,5.76697741277629,18.2274738311427));
#47692=CARTESIAN_POINT('Ctrl Pts',(23.7048488514242,4.21661613474277,15.6849072001887));
#47693=CARTESIAN_POINT('Ctrl Pts',(23.5659373609356,1.63894178445187,14.1936459524127));
#47694=CARTESIAN_POINT('Ctrl Pts',(23.427025870447,-1.3380352924883,14.117012743953));
#47695=CARTESIAN_POINT('Ctrl Pts',(23.2881143799583,-3.9890208389714,15.4736780665746));
#47696=CARTESIAN_POINT('Ctrl Pts',(23.1492028894697,-5.6681433743501,17.9331114721478));
#47697=CARTESIAN_POINT('Ctrl Pts',(23.0102913989811,-5.96631075568467,20.8961101859467));
#47698=CARTESIAN_POINT('Ctrl Pts',(22.8713799084924,-4.81087912857205,23.6407855620767));
#47699=CARTESIAN_POINT('Ctrl Pts',(22.7324684180038,-2.48335147471651,25.4984400471206));
#47700=CARTESIAN_POINT('Ctrl Pts',(22.5935569275151,0.449206220163045,26.0164849597188));
#47701=CARTESIAN_POINT('Ctrl Pts',(22.4546454370265,3.27232179193575,25.068706697845));
#47702=CARTESIAN_POINT('Ctrl Pts',(22.3157339465378,5.29818695103998,22.8860167238922));
#47703=CARTESIAN_POINT('Ctrl Pts',(22.1768224560493,6.03323109629379,20.0001935709956));
#47704=CARTESIAN_POINT('Ctrl Pts',(22.0379109655606,5.29837213082718,17.1143232575304));
#47705=CARTESIAN_POINT('Ctrl Pts',(21.898999475072,3.27264703532933,14.9315032918126));
#47706=CARTESIAN_POINT('Ctrl Pts',(21.7600879845833,0.44959228665845,13.983543877453));
#47707=CARTESIAN_POINT('Ctrl Pts',(21.6211764940947,-2.48299864422846,14.5014006118362));
#47708=CARTESIAN_POINT('Ctrl Pts',(21.4822650036061,-4.81064549576327,16.358905739637));
#47709=CARTESIAN_POINT('Ctrl Pts',(21.3433535131174,-5.96625324156263,19.1035069680698));
#47710=CARTESIAN_POINT('Ctrl Pts',(21.2044420226288,-5.6682759913379,22.066524808653));
#47711=CARTESIAN_POINT('Ctrl Pts',(21.0655305321402,-3.9893112769984,24.5260659555479));
#47712=CARTESIAN_POINT('Ctrl Pts',(20.9266190416515,-1.33841279083736,25.8829013845278));
#47713=CARTESIAN_POINT('Ctrl Pts',(20.7877075511629,1.63856919739414,25.8064592036892));
#47714=CARTESIAN_POINT('Ctrl Pts',(20.6487960606742,4.21633923402979,24.3153633638823));
#47715=CARTESIAN_POINT('Ctrl Pts',(20.5098845701856,5.76686366096883,21.7728962221611));
#47716=CARTESIAN_POINT('Ctrl Pts',(20.370973079697,5.91238126833391,18.798490434241));
#47717=CARTESIAN_POINT('Ctrl Pts',(20.2320615892084,4.61743894976846,16.1168138025692));
#47718=CARTESIAN_POINT('Ctrl Pts',(20.0931500987197,2.19752930150873,14.381215214322));
#47719=CARTESIAN_POINT('Ctrl Pts',(19.9542386082311,-0.757774251713633,
14.0145463261173));
#47720=CARTESIAN_POINT('Ctrl Pts',(19.8153271177424,-3.52845787043656,15.1061403212485));
#47721=CARTESIAN_POINT('Ctrl Pts',(19.6764156272538,-5.43948749662697,17.3900472661761));
#47722=CARTESIAN_POINT('Ctrl Pts',(19.5375041367651,-6.02527042425674,20.3098286838448));
#47723=CARTESIAN_POINT('Ctrl Pts',(19.3985926462765,-5.14308973534492,23.1541251517569));
#47724=CARTESIAN_POINT('Ctrl Pts',(19.2596811557879,-3.0078750618172,25.2299679837695));
#47725=CARTESIAN_POINT('Ctrl Pts',(19.1207696652993,-0.139838316756449,
26.0316102944341));
#47726=CARTESIAN_POINT('Ctrl Pts',(18.9818581748106,2.76226786365617,25.3637443775937));
#47727=CARTESIAN_POINT('Ctrl Pts',(18.842946684322,4.99139035413101,23.3890853974847));
#47728=CARTESIAN_POINT('Ctrl Pts',(18.7040351938333,6.00443805959323,20.5887283645827));
#47729=CARTESIAN_POINT('Ctrl Pts',(18.5651237033447,5.55459763081084,17.6449368037043));
#47730=CARTESIAN_POINT('Ctrl Pts',(18.426212212856,3.75146570597672,15.2749198360624));
#47731=CARTESIAN_POINT('Ctrl Pts',(18.2873007223674,1.03434739093725,14.0560953091745));
#47732=CARTESIAN_POINT('Ctrl Pts',(18.1483892318788,-1.93477361109326,14.2854109008107));
#47733=CARTESIAN_POINT('Ctrl Pts',(18.0094777413902,-4.43251705372066,15.9069974264324));
#47734=CARTESIAN_POINT('Ctrl Pts',(17.8705662509015,-5.85034651632709,18.5257804988213));
#47735=CARTESIAN_POINT('Ctrl Pts',(17.7316547604129,-5.84282985744584,21.5037342703069));
#47736=CARTESIAN_POINT('Ctrl Pts',(17.5927432699242,-4.41179839434207,24.1153265273167));
#47737=CARTESIAN_POINT('Ctrl Pts',(17.4538317794356,-1.90590073098647,25.7242833527334));
#47738=CARTESIAN_POINT('Ctrl Pts',(17.314920288947,1.06434006268985,25.9386073897598));
#47739=CARTESIAN_POINT('Ctrl Pts',(17.1760087984583,3.77527092043926,24.7060819134437));
#47740=CARTESIAN_POINT('Ctrl Pts',(17.0370973079697,5.56641561697647,22.3269926252217));
#47741=CARTESIAN_POINT('Ctrl Pts',(16.8981858174811,6.00138954856782,19.3809677027029));
#47742=CARTESIAN_POINT('Ctrl Pts',(16.7592743269924,4.97421806830788,16.5857603909984));
#47743=CARTESIAN_POINT('Ctrl Pts',(16.6203628365038,2.73515556393329,14.6223795652872));
#47744=CARTESIAN_POINT('Ctrl Pts',(16.4814513460151,-0.170285139380104,
13.9691724887821));
#47745=CARTESIAN_POINT('Ctrl Pts',(16.3425398555265,-3.03423851159519,14.7852829268014));
#47746=CARTESIAN_POINT('Ctrl Pts',(16.2036283650379,-5.15894676694387,16.8718782385279));
#47747=CARTESIAN_POINT('Ctrl Pts',(16.0647168745492,-6.02675771805542,19.7205918637273));
#47748=CARTESIAN_POINT('Ctrl Pts',(15.9258053840606,-5.42624269657667,22.6373789444455));
#47749=CARTESIAN_POINT('Ctrl Pts',(15.786893893572,-3.50370786648795,24.9116095819056));
#47750=CARTESIAN_POINT('Ctrl Pts',(15.6479824030833,-0.727548998167088,
25.989202781174));
#47751=CARTESIAN_POINT('Ctrl Pts',(15.5090709125947,2.22586589077336,25.6076196853075));
#47752=CARTESIAN_POINT('Ctrl Pts',(15.3701594221061,4.63698310460833,23.8598270928026));
#47753=CARTESIAN_POINT('Ctrl Pts',(15.2312479316174,5.91837135878041,21.1716475401432));
#47754=CARTESIAN_POINT('Ctrl Pts',(15.0923364411288,5.75784029446099,18.1980142502679));
#47755=CARTESIAN_POINT('Ctrl Pts',(14.9534249506401,4.19450081375939,15.6634068184659));
#47756=CARTESIAN_POINT('Ctrl Pts',(14.8145134601515,1.60923631549108,14.1853430041265));
#47757=CARTESIAN_POINT('Ctrl Pts',(14.6756019696629,-1.36809363299307,14.1239301135776));
#47758=CARTESIAN_POINT('Ctrl Pts',(14.5366904791742,-4.01210880291211,15.4941304443702));
#47759=CARTESIAN_POINT('Ctrl Pts',(14.3977789886856,-5.67863593767664,17.9621159537198));
#47760=CARTESIAN_POINT('Ctrl Pts',(14.258867498197,-5.96165156820477,20.9266002795585));
#47761=CARTESIAN_POINT('Ctrl Pts',(14.1199560077083,-4.7922033289967,23.6653328296771));
#47762=CARTESIAN_POINT('Ctrl Pts',(13.9810445172197,-2.45520913173245,25.5110639279737));
#47763=CARTESIAN_POINT('Ctrl Pts',(13.8421330267311,0.479958661504232,26.0141098411987));
#47764=CARTESIAN_POINT('Ctrl Pts',(13.7032215362424,3.29819197663088,25.0519112407131));
#47765=CARTESIAN_POINT('Ctrl Pts',(13.5643100457538,5.31287201013686,22.8588928805851));
#47766=CARTESIAN_POINT('Ctrl Pts',(13.4253985552651,6.03315324308028,19.9693496449273));
#47767=CARTESIAN_POINT('Ctrl Pts',(13.2864870647765,5.28355033303033,17.087273892538));
#47768=CARTESIAN_POINT('Ctrl Pts',(13.1475755742879,3.24669239392315,14.9148386458247));
#47769=CARTESIAN_POINT('Ctrl Pts',(13.0086640837993,0.418828247161937,13.9813240328013));
#47770=CARTESIAN_POINT('Ctrl Pts',(12.8697525933106,-2.51107690110167,14.5141663992143));
#47771=CARTESIAN_POINT('Ctrl Pts',(12.730841102822,-4.82919713854782,16.3835469730967));
#47772=CARTESIAN_POINT('Ctrl Pts',(12.5919296123333,-5.9707584504467,19.1340201935521));
#47773=CARTESIAN_POINT('Ctrl Pts',(12.4530181218447,-5.65763714210527,22.0954759523857));
#47774=CARTESIAN_POINT('Ctrl Pts',(12.314106631356,-3.96612036013178,24.5464015207309));
#47775=CARTESIAN_POINT('Ctrl Pts',(12.1751951408674,-1.30831991326933,25.8896669263464));
#47776=CARTESIAN_POINT('Ctrl Pts',(12.0362836503788,1.66823237313624,25.798006402892));
#47777=CARTESIAN_POINT('Ctrl Pts',(11.8973721598901,4.23834573559875,24.2937516141817));
#47778=CARTESIAN_POINT('Ctrl Pts',(11.7584606694015,5.77585194583529,21.7433908909211));
#47779=CARTESIAN_POINT('Ctrl Pts',(11.6195491789129,5.90616148040345,18.7682800374458));
#47780=CARTESIAN_POINT('Ctrl Pts',(11.4806376884242,4.59752644382878,16.0932586344818));
#47781=CARTESIAN_POINT('Ctrl Pts',(11.3417261979356,2.16877545055644,14.3700541260311));
#47782=CARTESIAN_POINT('Ctrl Pts',(11.202814707447,-0.788364018202142,14.0184985435461));
#47783=CARTESIAN_POINT('Ctrl Pts',(11.0639032169583,-3.55343083066098,15.1242429479655));
#47784=CARTESIAN_POINT('Ctrl Pts',(10.9249917264697,-5.45275937645092,17.417889878165));
#47785=CARTESIAN_POINT('Ctrl Pts',(10.786080235981,-6.02360773616301,20.3406278608587));
#47786=CARTESIAN_POINT('Ctrl Pts',(10.6471687454924,-5.12689756747983,23.1803771523713));
#47787=CARTESIAN_POINT('Ctrl Pts',(10.5082572550038,-2.9810983845514,25.2452769155099));
#47788=CARTESIAN_POINT('Ctrl Pts',(10.3693457645151,-0.109000851886715,
26.0322463737023));
#47789=CARTESIAN_POINT('Ctrl Pts',(10.2304342740265,2.78965304646366,25.3495526335491));
#47790=CARTESIAN_POINT('Ctrl Pts',(10.0915227835379,5.00865128014925,23.363523428284));
#47791=CARTESIAN_POINT('Ctrl Pts',(9.95261129304924,6.00736937211653,20.5580239472569));
#47792=CARTESIAN_POINT('Ctrl Pts',(9.8136998025606,5.5424851610418,17.6165705929506));
#47793=CARTESIAN_POINT('Ctrl Pts',(9.67478831207196,3.72726046916863,15.2558028188397));
#47794=CARTESIAN_POINT('Ctrl Pts',(9.53587682158333,1.00394661733243,14.0508850500009));
#47795=CARTESIAN_POINT('Ctrl Pts',(9.39696533109468,-1.96396324487712,14.2953767984618));
#47796=CARTESIAN_POINT('Ctrl Pts',(9.25805384060606,-4.45338394648429,15.929711444633));
#47797=CARTESIAN_POINT('Ctrl Pts',(9.11914235011741,-5.85780677353792,18.5557087195966));
#47798=CARTESIAN_POINT('Ctrl Pts',(8.98023085962879,-5.83506590323019,21.5335851472013));
#47799=CARTESIAN_POINT('Ctrl Pts',(8.84131936914014,-4.39070179563497,24.1378273575107));
#47800=CARTESIAN_POINT('Ctrl Pts',(8.7024078786515,-1.87661134660821,25.7339521582009));
#47801=CARTESIAN_POINT('Ctrl Pts',(8.56349638816287,1.09468632885601,25.9330885161248));
#47802=CARTESIAN_POINT('Ctrl Pts',(8.42458489767425,3.79928067166699,24.6867199486051));
#47803=CARTESIAN_POINT('Ctrl Pts',(8.2856734071856,5.57823925005091,22.2985048113823));
#47804=CARTESIAN_POINT('Ctrl Pts',(8.14676191669697,5.99814641881297,19.3502946535258));
#47805=CARTESIAN_POINT('Ctrl Pts',(8.00785042620833,4.95669831394964,16.5603751188182));
#47806=CARTESIAN_POINT('Ctrl Pts',(7.86893893571969,2.70762760118508,14.6084667976487));
#47807=CARTESIAN_POINT('Ctrl Pts',(7.73002744523105,-0.201114549674929,
13.9701218555708));
#47808=CARTESIAN_POINT('Ctrl Pts',(7.59111595474242,-3.06085826214264,14.800863129535));
#47809=CARTESIAN_POINT('Ctrl Pts',(7.45220446425378,-5.17487136870639,16.8982934026413));
#47810=CARTESIAN_POINT('Ctrl Pts',(7.31329297376514,-6.02810738899013,19.7514063444921));
#47811=CARTESIAN_POINT('Ctrl Pts',(7.1743814832765,-5.41268861030941,22.6650852719158));
#47812=CARTESIAN_POINT('Ctrl Pts',(7.03546999278787,-3.47855226575563,24.9294575394421));
#47813=CARTESIAN_POINT('Ctrl Pts',(6.89655850229923,-0.696920654630925,
25.9928439909533));
#47814=CARTESIAN_POINT('Ctrl Pts',(6.7576470118106,2.25450485661422,25.5961670230846));
#47815=CARTESIAN_POINT('Ctrl Pts',(6.61873552132196,4.65665525325171,23.8360708219635));
#47816=CARTESIAN_POINT('Ctrl Pts',(6.47982403083332,5.92428387655414,21.1413755073405));
#47817=CARTESIAN_POINT('Ctrl Pts',(6.34091254034468,5.74855268818165,18.1686017664212));
#47818=CARTESIAN_POINT('Ctrl Pts',(6.20200104985605,4.17227586453774,15.6420197787333));
#47819=CARTESIAN_POINT('Ctrl Pts',(6.06308955936741,1.57948878723643,14.177192028776));
#47820=CARTESIAN_POINT('Ctrl Pts',(5.92417806887878,-1.39811621675317,14.1310010612364));
#47821=CARTESIAN_POINT('Ctrl Pts',(5.78526657839015,-4.0350919056455,15.5147005883943));
#47822=CARTESIAN_POINT('Ctrl Pts',(5.64635508790151,-5.68898008313875,17.991173697801));
#47823=CARTESIAN_POINT('Ctrl Pts',(5.50744359741287,-5.95683656591226,20.9570661553763));
#47824=CARTESIAN_POINT('Ctrl Pts',(5.36853210692424,-4.77340227952123,23.6897842994703));
#47825=CARTESIAN_POINT('Ctrl Pts',(5.2296206164356,-2.4270026189548,25.5235437706551));
#47826=CARTESIAN_POINT('Ctrl Pts',(5.09070912594696,0.510698558558281,26.011577536807));
#47827=CARTESIAN_POINT('Ctrl Pts',(4.95179763545832,3.32397595917902,25.0349837459078));
#47828=CARTESIAN_POINT('Ctrl Pts',(4.81288614496969,5.32741821104193,22.8316943167324));
#47829=CARTESIAN_POINT('Ctrl Pts',(4.67397465448105,6.03291770627337,19.9385065199425));
#47830=CARTESIAN_POINT('Ctrl Pts',(4.53506316399242,5.26859044339846,17.0603006550862));
#47831=CARTESIAN_POINT('Ctrl Pts',(4.39615167350378,3.22065289637257,14.8983069065414));
#47832=CARTESIAN_POINT('Ctrl Pts',(4.25724018301514,0.388053261093601,13.9792614933621));
#47833=CARTESIAN_POINT('Ctrl Pts',(4.1183286925265,-2.53908952801089,14.5270755653402));
#47834=CARTESIAN_POINT('Ctrl Pts',(3.97941720203786,-4.84762256455593,16.4082827268317));
#47835=CARTESIAN_POINT('Ctrl Pts',(3.84050571154924,-5.97510760649766,19.1645560524418));
#47836=CARTESIAN_POINT('Ctrl Pts',(3.70159422106059,-5.64685042383923,22.1243723283741));
#47837=CARTESIAN_POINT('Ctrl Pts',(3.56268273057196,-3.94282578401499,24.5666182603398));
#47838=CARTESIAN_POINT('Ctrl Pts',(3.42377124008332,-1.27819284122356,25.896278534746));
#47839=CARTESIAN_POINT('Ctrl Pts',(3.28485974959469,1.6978519476731,25.7894020643622));
#47840=CARTESIAN_POINT('Ctrl Pts',(3.14594825910605,4.26024146295097,24.272027642166));
#47841=CARTESIAN_POINT('Ctrl Pts',(3.00703676861741,5.78468927206021,21.7138399941772));
#47842=CARTESIAN_POINT('Ctrl Pts',(2.86812527812878,5.89978732780536,18.7381018329537));
#47843=CARTESIAN_POINT('Ctrl Pts',(2.72921378764015,4.57749377640302,16.0698055740032));
#47844=CARTESIAN_POINT('Ctrl Pts',(2.59030229715151,2.13996491549558,14.3590401824333));
#47845=CARTESIAN_POINT('Ctrl Pts',(2.45139080666287,-0.818933178687291,
14.0226070957675));
#47846=CARTESIAN_POINT('Ctrl Pts',(2.31247931617423,-3.57831092008871,15.1424730060344));
#47847=CARTESIAN_POINT('Ctrl Pts',(2.1735678256856,-5.46588873739256,17.4457999812319));
#47848=CARTESIAN_POINT('Ctrl Pts',(2.03465633519696,-6.02178762295823,20.3714181261455));
#47849=CARTESIAN_POINT('Ctrl Pts',(1.89574484470832,-5.11057138435912,23.2065460478256));
#47850=CARTESIAN_POINT('Ctrl Pts',(1.75683335421969,-2.95424382766933,25.2604487207597));
#47851=CARTESIAN_POINT('Ctrl Pts',(1.61792186373105,-0.0781604693793413,
26.0327248619724));
#47852=CARTESIAN_POINT('Ctrl Pts',(1.47901037324242,2.81696518293041,25.3352209369218));
#47853=CARTESIAN_POINT('Ctrl Pts',(1.34009888275377,5.02578156596024,23.3378738167095));
#47854=CARTESIAN_POINT('Ctrl Pts',(1.20118739226514,6.01014314938957,20.527304418837));
#47855=CARTESIAN_POINT('Ctrl Pts',(1.0622759017765,5.53022886704606,17.5882677129498));
#47856=CARTESIAN_POINT('Ctrl Pts',(0.923364411287864,3.7029557770085,15.2368077542205));
#47857=CARTESIAN_POINT('Ctrl Pts',(0.784452920799229,0.973523620615991,
14.0458343013086));
#47858=CARTESIAN_POINT('Ctrl Pts',(0.645541430310594,-1.99310945899281,
14.3054838683065));
#47859=CARTESIAN_POINT('Ctrl Pts',(0.506629939821949,-4.47411886205269,
15.9525474555556));
#47860=CARTESIAN_POINT('Ctrl Pts',(0.367718449333321,-5.86514463181102,
18.5856439254866));
#47861=CARTESIAN_POINT('Ctrl Pts',(0.228806958844683,-5.82708887344388,
21.5634566994412));
#47862=CARTESIAN_POINT('Ctrl Pts',(0.089895468356049,-4.36961084196237,
24.1600984966641));
#47863=CARTESIAN_POINT('Ctrl Pts',(-0.049016022132584,-1.8470232551417,
25.7437316612543));
#47864=CARTESIAN_POINT('Ctrl Pts',(-0.141623682458342,0.133898761891108,
25.8656596766911));
#47865=CARTESIAN_POINT('Ctrl Pts',(-0.187927512621222,1.07922963693981,
25.6862389549904));
#47866=CARTESIAN_POINT('Ctrl Pts',(50.5637825378637,4.61752854196214,24.0062770406782));
#47867=CARTESIAN_POINT('Ctrl Pts',(50.5174787077008,5.28356762518215,23.2386180781043));
#47868=CARTESIAN_POINT('Ctrl Pts',(50.424871047375,6.22471038456146,21.3654729984245));
#47869=CARTESIAN_POINT('Ctrl Pts',(50.2859595568864,6.11925893083018,18.221252859719));
#47870=CARTESIAN_POINT('Ctrl Pts',(50.1470480663978,4.52315605456026,15.511157237809));
#47871=CARTESIAN_POINT('Ctrl Pts',(50.0081365759091,1.82495675592641,13.894325809954));
#47872=CARTESIAN_POINT('Ctrl Pts',(49.8692250854205,-1.31781499742106,13.7652351533052));
#47873=CARTESIAN_POINT('Ctrl Pts',(49.7303135949318,-4.13954687382562,15.1550528216166));
#47874=CARTESIAN_POINT('Ctrl Pts',(49.5914021044433,-5.95272957145251,17.7253150705105));
#47875=CARTESIAN_POINT('Ctrl Pts',(49.4524906139545,-6.31562862148528,20.849744422951));
#47876=CARTESIAN_POINT('Ctrl Pts',(49.313579123466,-5.13981947893865,23.7671592113954));
#47877=CARTESIAN_POINT('Ctrl Pts',(49.1746676329772,-2.71177477849166,25.7667577971016));
#47878=CARTESIAN_POINT('Ctrl Pts',(49.0357561424887,0.376952608096762,26.3613785707909));
#47879=CARTESIAN_POINT('Ctrl Pts',(48.896844652,3.37384090977041,25.4061465625371));
#47880=CARTESIAN_POINT('Ctrl Pts',(48.7579331615114,5.54874546123675,23.1337916855913));
#47881=CARTESIAN_POINT('Ctrl Pts',(48.6190216710227,6.37178419535544,20.0979366854017));
#47882=CARTESIAN_POINT('Ctrl Pts',(48.4801101805342,5.64243666772738,17.0382211455748));
#47883=CARTESIAN_POINT('Ctrl Pts',(48.3411986900455,3.53839699735355,14.7000969433883));
#47884=CARTESIAN_POINT('Ctrl Pts',(48.2022871995569,0.572281835046422,13.653211912598));
#47885=CARTESIAN_POINT('Ctrl Pts',(48.0633757090682,-2.53326092100598,14.1526232585264));
#47886=CARTESIAN_POINT('Ctrl Pts',(47.9244642185796,-5.02161397036119,16.0766572005871));
#47887=CARTESIAN_POINT('Ctrl Pts',(47.7855527280909,-6.28652872164122,18.9565527116423));
#47888=CARTESIAN_POINT('Ctrl Pts',(47.6466412376024,-6.01982832642006,22.0906679621073));
#47889=CARTESIAN_POINT('Ctrl Pts',(47.5077297471136,-4.28649019781716,24.71542441243));
#47890=CARTESIAN_POINT('Ctrl Pts',(47.3688182566251,-1.50881526580176,26.1913408969229));
#47891=CARTESIAN_POINT('Ctrl Pts',(47.2299067661364,1.63645908624929,26.1588332714235));
#47892=CARTESIAN_POINT('Ctrl Pts',(47.0909952756477,4.38303558259688,24.6258215150332));
#47893=CARTESIAN_POINT('Ctrl Pts',(46.9520837851591,6.06175349129441,21.9658001469101));
#47894=CARTESIAN_POINT('Ctrl Pts',(46.8131722946704,6.26361925046179,18.8268420855787));
#47895=CARTESIAN_POINT('Ctrl Pts',(46.6742608041818,4.93945140114888,15.9737057406808));
#47896=CARTESIAN_POINT('Ctrl Pts',(46.5353493136932,2.41186288654182,14.1015134972249));
#47897=CARTESIAN_POINT('Ctrl Pts',(46.3964378232046,-0.703338584205735,
13.6663959357331));
#47898=CARTESIAN_POINT('Ctrl Pts',(46.257526332716,-3.64718252590797,14.7743626963189));
#47899=CARTESIAN_POINT('Ctrl Pts',(46.1186148422273,-5.70244705557887,17.1554748752666));
#47900=CARTESIAN_POINT('Ctrl Pts',(45.9797033517387,-6.36839887172476,20.2296114490435));
#47901=CARTESIAN_POINT('Ctrl Pts',(45.84079186125,-5.48278915103411,23.2478067572163));
#47902=CARTESIAN_POINT('Ctrl Pts',(45.7018803707614,-3.26138295580096,25.4747243604157));
#47903=CARTESIAN_POINT('Ctrl Pts',(45.5629688802727,-0.245391425534477,
26.3678103501275));
#47904=CARTESIAN_POINT('Ctrl Pts',(45.4240573897841,2.83038591667594,25.7094781871552));
#47905=CARTESIAN_POINT('Ctrl Pts',(45.2851458992955,5.21658366263703,23.6601202845843));
#47906=CARTESIAN_POINT('Ctrl Pts',(45.1462344088069,6.33184176934682,20.719030885896));
#47907=CARTESIAN_POINT('Ctrl Pts',(45.0073229183182,5.90444490978662,17.6027607724275));
#47908=CARTESIAN_POINT('Ctrl Pts',(44.8684114278296,4.03852169487032,15.0705407875732));
#47909=CARTESIAN_POINT('Ctrl Pts',(44.7294999373409,1.18867535364643,13.7393070263308));
#47910=CARTESIAN_POINT('Ctrl Pts',(44.5905884468523,-1.95077328725316,13.9333939316404));
#47911=CARTESIAN_POINT('Ctrl Pts',(44.4516769563636,-4.61494629599519,15.6055152415786));
#47912=CARTESIAN_POINT('Ctrl Pts',(44.3127654658751,-6.15475927144461,18.3482845531133));
#47913=CARTESIAN_POINT('Ctrl Pts',(44.1738539753864,-6.19506068261978,21.4934686958809));
#47914=CARTESIAN_POINT('Ctrl Pts',(44.0349424848978,-4.72603171623352,24.2747923720425));
#47915=CARTESIAN_POINT('Ctrl Pts',(43.8960309944091,-2.10557847814608,26.0146292387217));
#47916=CARTESIAN_POINT('Ctrl Pts',(43.7571195039205,1.02786627402308,26.2890950485458));
#47917=CARTESIAN_POINT('Ctrl Pts',(43.6182080134318,3.91088736273947,25.0313204671222));
#47918=CARTESIAN_POINT('Ctrl Pts',(43.4792965229432,5.84108144907249,22.5477427484381));
#47919=CARTESIAN_POINT('Ctrl Pts',(43.3403850324546,6.34818670374496,19.4434470543486));
#47920=CARTESIAN_POINT('Ctrl Pts',(43.2014735419659,5.30865480258217,16.4747468468295));
#47921=CARTESIAN_POINT('Ctrl Pts',(43.0625620514773,2.9757515580194,14.3649198522237));
#47922=CARTESIAN_POINT('Ctrl Pts',(42.9236505609886,-0.0821473649868688,
13.6279926697042));
#47923=CARTESIAN_POINT('Ctrl Pts',(42.7847390705,-3.12003235757933,14.4435061689429));
#47924=CARTESIAN_POINT('Ctrl Pts',(42.6458275800114,-5.39776989439614,16.6127731439911));
#47925=CARTESIAN_POINT('Ctrl Pts',(42.5069160895228,-6.36042457890855,19.6072853670493));
#47926=CARTESIAN_POINT('Ctrl Pts',(42.3680045990341,-5.77346053925448,22.6974764148346));
#47927=CARTESIAN_POINT('Ctrl Pts',(42.2290931085455,-3.77988245302682,25.1304692035152));
#47928=CARTESIAN_POINT('Ctrl Pts',(42.0901816180568,-0.865394677250782,
26.3135028042683));
#47929=CARTESIAN_POINT('Ctrl Pts',(41.9512701275682,2.25993307925686,25.9583494429412));
#47930=CARTESIAN_POINT('Ctrl Pts',(41.8123586370795,4.83466321896507,24.151536723444));
#47931=CARTESIAN_POINT('Ctrl Pts',(41.673447146591,6.23150270747516,21.3332665201104));
#47932=CARTESIAN_POINT('Ctrl Pts',(41.5345356561023,6.11013328470932,18.1901666236902));
#47933=CARTESIAN_POINT('Ctrl Pts',(41.3956241656137,4.5001247266669,15.4880045377507));
#47934=CARTESIAN_POINT('Ctrl Pts',(41.256712675125,1.79373062847491,13.8851201124316));
#47935=CARTESIAN_POINT('Ctrl Pts',(41.1178011846364,-1.34967809562946,13.7720312585004));
#47936=CARTESIAN_POINT('Ctrl Pts',(40.9788896941477,-4.16425870100727,15.1762903198884));
#47937=CARTESIAN_POINT('Ctrl Pts',(40.8399782036591,-5.96428231018196,17.7557713727501));
#47938=CARTESIAN_POINT('Ctrl Pts',(40.7010667131705,-6.31120111017131,20.8820238964393));
#47939=CARTESIAN_POINT('Ctrl Pts',(40.5621552226819,-5.12049372012104,23.793384988255));
#47940=CARTESIAN_POINT('Ctrl Pts',(40.4232437321932,-2.68225751383601,25.7805467073961));
#47941=CARTESIAN_POINT('Ctrl Pts',(40.2843322417046,0.409469102548303,26.3593679450851));
#47942=CARTESIAN_POINT('Ctrl Pts',(40.145420751216,3.4014349277457,25.388827891038));
#47943=CARTESIAN_POINT('Ctrl Pts',(40.0065092607273,5.56469392878752,23.1053835650098));
#47944=CARTESIAN_POINT('Ctrl Pts',(39.8675977702387,6.37220162748716,20.0653607341416));
#47945=CARTESIAN_POINT('Ctrl Pts',(39.72868627975,5.62722130693377,17.0094137749083));
#47946=CARTESIAN_POINT('Ctrl Pts',(39.5897747892614,3.51125585888291,14.6820767304917));
#47947=CARTESIAN_POINT('Ctrl Pts',(39.4508632987728,0.539827421410421,13.6503691475795));
#47948=CARTESIAN_POINT('Ctrl Pts',(39.3119518082841,-2.56312158825944,14.1656505649116));
#47949=CARTESIAN_POINT('Ctrl Pts',(39.1730403177955,-5.04160580690685,16.1023806631893));
#47950=CARTESIAN_POINT('Ctrl Pts',(39.0341288273068,-6.29178102490108,18.9887052152749));
#47951=CARTESIAN_POINT('Ctrl Pts',(38.8952173368182,-6.0090614551994,22.1214160446631));
#47952=CARTESIAN_POINT('Ctrl Pts',(38.7563058463296,-4.26232733267651,24.7372767827135));
#47953=CARTESIAN_POINT('Ctrl Pts',(38.6173943558409,-1.47714331403435,26.1989735631571));
#47954=CARTESIAN_POINT('Ctrl Pts',(38.4784828653523,1.66792374532418,26.1503866534309));
#47955=CARTESIAN_POINT('Ctrl Pts',(38.3395713748636,4.40662707311566,24.6033534999391));
#47956=CARTESIAN_POINT('Ctrl Pts',(38.200659884375,6.0717241128045,21.9347847179741));
#47957=CARTESIAN_POINT('Ctrl Pts',(38.0617483938864,6.25753981577645,18.7948356705868));
#47958=CARTESIAN_POINT('Ctrl Pts',(37.9228369033978,4.91880307017454,15.9485062058842));
#47959=CARTESIAN_POINT('Ctrl Pts',(37.7839254129091,2.3816763046193,14.0892603181216));
#47960=CARTESIAN_POINT('Ctrl Pts',(37.6450139224205,-0.735708924935337,
13.6700744092298));
#47961=CARTESIAN_POINT('Ctrl Pts',(37.5061024319318,-3.67385009436911,14.7930766194401));
#47962=CARTESIAN_POINT('Ctrl Pts',(37.3671909414432,-5.71691471264096,17.1846648911174));
#47963=CARTESIAN_POINT('Ctrl Pts',(37.2282794509546,-6.36714179730726,20.2621658633391));
#47964=CARTESIAN_POINT('Ctrl Pts',(37.0893679604659,-5.46611361180679,23.2757941922132));
#47965=CARTESIAN_POINT('Ctrl Pts',(36.9504564699773,-3.23335168806423,25.4913261119888));
#47966=CARTESIAN_POINT('Ctrl Pts',(36.8115449794887,-0.212833812579934,
26.3689816591933));
#47967=CARTESIAN_POINT('Ctrl Pts',(36.672633489,2.85953771780081,25.6949336824402));
#47968=CARTESIAN_POINT('Ctrl Pts',(36.5337219985114,5.23522726807311,23.6334035089075));
#47969=CARTESIAN_POINT('Ctrl Pts',(36.3948105080228,6.33543495400973,20.6866509669615));
#47970=CARTESIAN_POINT('Ctrl Pts',(36.2558990175341,5.8921122500055,17.572606574893));
#47971=CARTESIAN_POINT('Ctrl Pts',(36.1169875270455,4.01326785177723,15.0499589136242));
#47972=CARTESIAN_POINT('Ctrl Pts',(35.9780760365568,1.15665303412888,13.7333119300896));
#47973=CARTESIAN_POINT('Ctrl Pts',(35.8391645460682,-1.98176234208496,13.9434462252522));
#47974=CARTESIAN_POINT('Ctrl Pts',(35.7002530555796,-4.63735208393372,15.6291658397334));
#47975=CARTESIAN_POINT('Ctrl Pts',(35.5613415650909,-6.16312297003413,18.3797713546678));
#47976=CARTESIAN_POINT('Ctrl Pts',(35.4224300746023,-6.18734460651764,21.5251204303643));
#47977=CARTESIAN_POINT('Ctrl Pts',(35.2835185841137,-4.70411576761554,24.2988975856361));
#47978=CARTESIAN_POINT('Ctrl Pts',(35.144607093625,-2.07480213772069,26.025315070287));
#47979=CARTESIAN_POINT('Ctrl Pts',(35.0056956031364,1.06000482861184,26.2837580610839));
#47980=CARTESIAN_POINT('Ctrl Pts',(34.8667841126477,3.93655807151044,25.0112609347891));
#47981=CARTESIAN_POINT('Ctrl Pts',(34.7278726221591,5.85403004228618,22.5178478649292));
#47982=CARTESIAN_POINT('Ctrl Pts',(34.5889611316705,6.34525845764879,19.4110002440119));
#47983=CARTESIAN_POINT('Ctrl Pts',(34.4500496411818,5.29056313888617,16.4476532713745));
#47984=CARTESIAN_POINT('Ctrl Pts',(34.3111381506932,2.94690422977004,14.3497804407721));
#47985=CARTESIAN_POINT('Ctrl Pts',(34.1722266602045,-0.114722154020674,
13.6284959048672));
#47986=CARTESIAN_POINT('Ctrl Pts',(34.033315169716,-3.14839826566498,14.459529445284));
#47987=CARTESIAN_POINT('Ctrl Pts',(33.8944036792273,-5.41501600831516,16.6404126389379));
#47988=CARTESIAN_POINT('Ctrl Pts',(33.7554921887387,-6.36234915069327,19.6398071466696));
#47989=CARTESIAN_POINT('Ctrl Pts',(33.61658069825,-5.75959467686212,22.7269570523165));
#47990=CARTESIAN_POINT('Ctrl Pts',(33.4776692077614,-3.75360435860782,25.1497261991253));
#47991=CARTESIAN_POINT('Ctrl Pts',(33.3387577172728,-0.833106600630097,
26.3178444899273));
#47992=CARTESIAN_POINT('Ctrl Pts',(33.1998462267841,2.29036464937583,25.9467180343284));
#47993=CARTESIAN_POINT('Ctrl Pts',(33.0609347362955,4.855824102872,24.1267660327289));
#47994=CARTESIAN_POINT('Ctrl Pts',(32.9220232458069,6.2382373842586,21.301391541603));
#47995=CARTESIAN_POINT('Ctrl Pts',(32.7831117553182,6.10080095490451,18.1589532011506));
#47996=CARTESIAN_POINT('Ctrl Pts',(32.6442002648296,4.47699906757734,15.4650573370957));
#47997=CARTESIAN_POINT('Ctrl Pts',(32.5052887743409,1.76244584798862,13.8760298629218));
#47998=CARTESIAN_POINT('Ctrl Pts',(32.3663772838523,-1.38149994633938,13.779012658333));
#47999=CARTESIAN_POINT('Ctrl Pts',(32.2274657933637,-4.18886472194398,15.197642459357));
#48000=CARTESIAN_POINT('Ctrl Pts',(32.088554302875,-5.97567762627104,17.7862921344945));
#48001=CARTESIAN_POINT('Ctrl Pts',(31.9496428123864,-6.30660942952213,20.9142773705939));
#48002=CARTESIAN_POINT('Ctrl Pts',(31.8107313218978,-5.10103373445315,23.8195131164703));
#48003=CARTESIAN_POINT('Ctrl Pts',(31.6718198314091,-2.65267034660569,25.7941837767848));
#48004=CARTESIAN_POINT('Ctrl Pts',(31.5329083409205,0.441974997287937,26.357191495361));
#48005=CARTESIAN_POINT('Ctrl Pts',(31.3939968504318,3.4289399932875,25.3713681803941));
#48006=CARTESIAN_POINT('Ctrl Pts',(31.2550853599432,5.58049698283711,23.0768943809405));
#48007=CARTESIAN_POINT('Ctrl Pts',(31.1161738694545,6.37245250121533,20.0327830241454));
#48008=CARTESIAN_POINT('Ctrl Pts',(30.977262378966,5.6118588788506,16.9806845923648));
#48009=CARTESIAN_POINT('Ctrl Pts',(30.8383508884773,3.48402294614019,14.6641954948025));
#48010=CARTESIAN_POINT('Ctrl Pts',(30.6994393979887,0.507358900497252,13.6476923442733));
#48011=CARTESIAN_POINT('Ctrl Pts',(30.5605279075,-2.59291526618855,14.1788303555657));
#48012=CARTESIAN_POINT('Ctrl Pts',(30.4216164170114,-5.06146587467247,16.1282059963831));
#48013=CARTESIAN_POINT('Ctrl Pts',(30.2827049265227,-6.29686888525375,19.0208841494284));
#48014=CARTESIAN_POINT('Ctrl Pts',(30.1437934360341,-5.99813752993638,22.1521086819411));
#48015=CARTESIAN_POINT('Ctrl Pts',(30.0048819455455,-4.23805306663042,24.7590053384444));
#48016=CARTESIAN_POINT('Ctrl Pts',(29.8659704550568,-1.4454327553499,26.2064442120009));
#48017=CARTESIAN_POINT('Ctrl Pts',(29.7270589645682,1.69934481122473,26.1417792877538));
#48018=CARTESIAN_POINT('Ctrl Pts',(29.5881474740796,4.43010339123342,24.5807651707875));
#48019=CARTESIAN_POINT('Ctrl Pts',(29.4492359835909,6.08153604262198,21.9037187211369));
#48020=CARTESIAN_POINT('Ctrl Pts',(29.3103244931023,6.2512968328913,18.762860753997));
#48021=CARTESIAN_POINT('Ctrl Pts',(29.1714130026136,4.89802618046513,15.9234125616644));
#48022=CARTESIAN_POINT('Ctrl Pts',(29.032501512125,2.35142747477107,14.0771616231904));
#48023=CARTESIAN_POINT('Ctrl Pts',(28.8935900216364,-0.76806003704259,13.673918322815));
#48024=CARTESIAN_POINT('Ctrl Pts',(28.7546785311478,-3.70042164241411,14.8119266316608));
#48025=CARTESIAN_POINT('Ctrl Pts',(28.6157670406591,-5.73123295137762,17.2139284890799));
#48026=CARTESIAN_POINT('Ctrl Pts',(28.4768555501705,-6.36571831011055,20.29471342562));
#48027=CARTESIAN_POINT('Ctrl Pts',(28.3379440596818,-5.4492952092373,23.3036960104557));
#48028=CARTESIAN_POINT('Ctrl Pts',(28.1990325691932,-3.2052359128581,25.5077843412612));
#48029=CARTESIAN_POINT('Ctrl Pts',(28.0601210787046,-0.180270636962042,
26.3699865073929));
#48030=CARTESIAN_POINT('Ctrl Pts',(27.9212095882159,2.88861478152641,25.6802403339));
#48031=CARTESIAN_POINT('Ctrl Pts',(27.7822980977273,5.2537340446546,23.6065917699339));
#48032=CARTESIAN_POINT('Ctrl Pts',(27.6433866072386,6.33886255458932,20.6542531015921));
#48033=CARTESIAN_POINT('Ctrl Pts',(27.50447511675,5.87962559290408,17.5425158201557));
#48034=CARTESIAN_POINT('Ctrl Pts',(27.3655636262614,3.98790911718367,15.0295064148517));
#48035=CARTESIAN_POINT('Ctrl Pts',(27.2266521357728,1.12460048411671,13.7274806211505));
#48036=CARTESIAN_POINT('Ctrl Pts',(27.0877406452841,-2.01269960121476,13.953656814058));
#48037=CARTESIAN_POINT('Ctrl Pts',(26.9488291547955,-4.65963666919246,15.6529306748069));
#48038=CARTESIAN_POINT('Ctrl Pts',(26.8099176643068,-6.17132558811776,18.4113005028136));
#48039=CARTESIAN_POINT('Ctrl Pts',(26.6710061738182,-6.17946681684849,21.556732304022));
#48040=CARTESIAN_POINT('Ctrl Pts',(26.5320946833296,-4.68207687136995,24.3228904424587));
#48041=CARTESIAN_POINT('Ctrl Pts',(26.3931831928409,-2.04397156988813,26.0358434231188));
#48042=CARTESIAN_POINT('Ctrl Pts',(26.2542717023523,1.09211567872115,26.2782568401754));
#48043=CARTESIAN_POINT('Ctrl Pts',(26.1153602118636,3.96212589368178,24.9910704272264));
#48044=CARTESIAN_POINT('Ctrl Pts',(25.976448721375,5.86682563350311,22.4878871744893));
#48045=CARTESIAN_POINT('Ctrl Pts',(25.8375372308864,6.34216437072042,19.3785688278802));
#48046=CARTESIAN_POINT('Ctrl Pts',(25.6986257403977,5.27233320006711,16.4206525407014));
#48047=CARTESIAN_POINT('Ctrl Pts',(25.5597142499091,2.91797988069426,14.3347887044894));
#48048=CARTESIAN_POINT('Ctrl Pts',(25.4208027594205,-0.147293944655354,
13.6291656668231));
#48049=CARTESIAN_POINT('Ctrl Pts',(25.2818912689318,-3.17668188663938,14.4756975283739));
#48050=CARTESIAN_POINT('Ctrl Pts',(25.1429797784432,-5.43212059438828,16.6681399406727));
#48051=CARTESIAN_POINT('Ctrl Pts',(25.0040682879545,-6.3641074349603,19.672338340356));
#48052=CARTESIAN_POINT('Ctrl Pts',(24.8651567974659,-5.74557828065295,22.7563664175516));
#48053=CARTESIAN_POINT('Ctrl Pts',(24.7262453069773,-3.72722815930074,25.1688486005525));
#48054=CARTESIAN_POINT('Ctrl Pts',(24.5873338164887,-0.800796749783299,
26.3220210512505));
#48055=CARTESIAN_POINT('Ctrl Pts',(24.448422326,2.32073635810671,25.9349312012086));
#48056=CARTESIAN_POINT('Ctrl Pts',(24.3095108355114,4.87685807407465,24.1018874841042));
#48057=CARTESIAN_POINT('Ctrl Pts',(24.1705993450227,6.24480901733213,21.2694825496889));
#48058=CARTESIAN_POINT('Ctrl Pts',(24.0316878545341,6.09130917345336,18.1277878965458));
#48059=CARTESIAN_POINT('Ctrl Pts',(23.8927763640454,4.45375639682368,15.4422286625293));
#48060=CARTESIAN_POINT('Ctrl Pts',(23.7538648735569,1.73111500389623,13.8670996706124));
#48061=CARTESIAN_POINT('Ctrl Pts',(23.6149533830682,-1.41328568991475,13.7861566510251));
#48062=CARTESIAN_POINT('Ctrl Pts',(23.4760418925796,-4.21336126194841,15.2191201141181));
#48063=CARTESIAN_POINT('Ctrl Pts',(23.3371304020909,-5.98691676095991,17.8168707541113));
#48064=CARTESIAN_POINT('Ctrl Pts',(23.1982189116023,-6.30185291817879,20.9465069490283));
#48065=CARTESIAN_POINT('Ctrl Pts',(23.0593074211136,-5.08144042723737,23.8455414171941));
#48066=CARTESIAN_POINT('Ctrl Pts',(22.920395930625,-2.62301384869953,25.8076694083296));
#48067=CARTESIAN_POINT('Ctrl Pts',(22.7814844401364,0.474469340488402,26.3548488929206));
#48068=CARTESIAN_POINT('Ctrl Pts',(22.6425729496477,3.45635543942831,25.353768082692));
#48069=CARTESIAN_POINT('Ctrl Pts',(22.5036614591591,5.59615418399987,23.0483247785986));
#48070=CARTESIAN_POINT('Ctrl Pts',(22.3647499686705,6.37253682336279,20.0002044573261));
#48071=CARTESIAN_POINT('Ctrl Pts',(22.2258384781818,5.59634977820039,16.9520343231995));
#48072=CARTESIAN_POINT('Ctrl Pts',(22.0869269876932,3.45669897433838,14.6464537166729));
#48073=CARTESIAN_POINT('Ctrl Pts',(21.9480154972045,0.474877119159393,13.6451815660385));
#48074=CARTESIAN_POINT('Ctrl Pts',(21.8091040067159,-2.62264117521137,14.1921622893711));
#48075=CARTESIAN_POINT('Ctrl Pts',(21.6701925162273,-5.08119365504295,16.1541325234911));
#48076=CARTESIAN_POINT('Ctrl Pts',(21.5312810257387,-6.30179216949294,19.0530886739324));
#48077=CARTESIAN_POINT('Ctrl Pts',(21.39236953525,-5.98705683625699,22.1827450713141));
#48078=CARTESIAN_POINT('Ctrl Pts',(21.2534580447614,-4.21366803405649,24.7806095119438));
#48079=CARTESIAN_POINT('Ctrl Pts',(21.1145465542727,-1.41368441857138,26.2137526480868));
#48080=CARTESIAN_POINT('Ctrl Pts',(20.9756350637841,1.73072146273936,26.1330113994131));
#48081=CARTESIAN_POINT('Ctrl Pts',(20.8367235732955,4.453463923361,24.5580571179221));
#48082=CARTESIAN_POINT('Ctrl Pts',(20.6978120828068,6.09118902430437,21.8726029683601));
#48083=CARTESIAN_POINT('Ctrl Pts',(20.5589005923182,6.2448904649721,18.7309181715043));
#48084=CARTESIAN_POINT('Ctrl Pts',(20.4199891018296,4.87712127505025,15.8984254638773));
#48085=CARTESIAN_POINT('Ctrl Pts',(20.2810776113409,2.32111718758555,14.0652177286431));
#48086=CARTESIAN_POINT('Ctrl Pts',(20.1421661208523,-0.800391074992589,
13.6779275760247));
#48087=CARTESIAN_POINT('Ctrl Pts',(20.0032546303637,-3.72689647556414,14.8309122403131));
#48088=CARTESIAN_POINT('Ctrl Pts',(19.864343139875,-5.74540139756466,17.2432649043154));
#48089=CARTESIAN_POINT('Ctrl Pts',(19.7254316493864,-6.36412844733921,20.3272532852169));
#48090=CARTESIAN_POINT('Ctrl Pts',(19.5865201588977,-5.43233438289444,23.3315114826968));
#48091=CARTESIAN_POINT('Ctrl Pts',(19.4476086684091,-3.17703636502164,25.5240986180776));
#48092=CARTESIAN_POINT('Ctrl Pts',(19.3086971779205,-0.14770274975791,26.3708248684634));
#48093=CARTESIAN_POINT('Ctrl Pts',(19.1697856874318,2.91761634788927,25.6653985255625));
#48094=CARTESIAN_POINT('Ctrl Pts',(19.0308741969432,5.27210350868496,23.5796857684201));
#48095=CARTESIAN_POINT('Ctrl Pts',(18.8919627064546,6.34212448150116,20.6218381365444));
#48096=CARTESIAN_POINT('Ctrl Pts',(18.7530512159659,5.86698526483596,17.5124892946733));
#48097=CARTESIAN_POINT('Ctrl Pts',(18.6141397254773,3.96244615387019,15.0091838258059));
#48098=CARTESIAN_POINT('Ctrl Pts',(18.4752282349886,1.09251854134113,13.7218132519219));
#48099=CARTESIAN_POINT('Ctrl Pts',(18.3363167445,-2.0435842560608,13.9640254311919));
#48100=CARTESIAN_POINT('Ctrl Pts',(18.1974052540114,-4.68179946933745,15.6768091256771));
#48101=CARTESIAN_POINT('Ctrl Pts',(18.0584937635227,-6.17936691131037,18.4428711734991));
#48102=CARTESIAN_POINT('Ctrl Pts',(17.9195822730341,-6.17142751950771,21.5883034906404));
#48103=CARTESIAN_POINT('Ctrl Pts',(17.7806707825455,-4.65991560350942,24.3467703154281));
#48104=CARTESIAN_POINT('Ctrl Pts',(17.6417592920568,-2.01308758044197,26.0462140220462));
#48105=CARTESIAN_POINT('Ctrl Pts',(17.5028478015682,1.12419798509589,26.2725915296011));
#48106=CARTESIAN_POINT('Ctrl Pts',(17.3639363110796,3.98759016100821,24.9707494721368));
#48107=CARTESIAN_POINT('Ctrl Pts',(17.2250248205909,5.87946788829534,22.4578614601765));
#48108=CARTESIAN_POINT('Ctrl Pts',(17.0861133301023,6.33890452382744,19.3461536535871));
#48109=CARTESIAN_POINT('Ctrl Pts',(16.9472018396136,5.25396546258616,16.3937453605064));
#48110=CARTESIAN_POINT('Ctrl Pts',(16.808290349125,2.88897926676432,14.3199450352023));
#48111=CARTESIAN_POINT('Ctrl Pts',(16.6693788586364,-0.179861885588608,
13.630001938067));
#48112=CARTESIAN_POINT('Ctrl Pts',(16.5304673681478,-3.2048824812767,14.4920099956406));
#48113=CARTESIAN_POINT('Ctrl Pts',(16.3915558776591,-5.44908320556687,16.6959543245097));
#48114=CARTESIAN_POINT('Ctrl Pts',(16.2526443871705,-6.36569938575479,19.7048780978672));
#48115=CARTESIAN_POINT('Ctrl Pts',(16.1137328966818,-5.73141171696209,22.7857037418913));
#48116=CARTESIAN_POINT('Ctrl Pts',(15.9748214061932,-3.70075454447885,25.1878359080099));
#48117=CARTESIAN_POINT('Ctrl Pts',(15.8359099157046,-0.768465969166765,
26.3260323790785));
#48118=CARTESIAN_POINT('Ctrl Pts',(15.6969984252159,2.35104741164878,25.9229892516446));
#48119=CARTESIAN_POINT('Ctrl Pts',(15.5580869347273,4.89776458282526,24.0769017278002));
#48120=CARTESIAN_POINT('Ctrl Pts',(15.4191754442386,6.25121743493832,21.2375403783475));
#48121=CARTESIAN_POINT('Ctrl Pts',(15.28026395375,6.08165818843483,18.096671524418));
#48122=CARTESIAN_POINT('Ctrl Pts',(15.1413524632613,4.43039732188061,15.4195191107057));
#48123=CARTESIAN_POINT('Ctrl Pts',(15.0024409727728,1.69973891506645,13.8583297689044));
#48124=CARTESIAN_POINT('Ctrl Pts',(14.8635294822841,-1.44503449559759,13.7934630498602));
#48125=CARTESIAN_POINT('Ctrl Pts',(14.7246179917955,-4.23774768077446,15.2407227228278));
#48126=CARTESIAN_POINT('Ctrl Pts',(14.5857065013068,-5.99799942050051,17.8475064323922));
#48127=CARTESIAN_POINT('Ctrl Pts',(14.4467950108182,-6.29693170045833,20.9787117893846));
#48128=CARTESIAN_POINT('Ctrl Pts',(14.3078835203295,-5.06171431056786,23.8714692101462));
#48129=CARTESIAN_POINT('Ctrl Pts',(14.1689720298409,-2.59328879522498,25.8210032495677));
#48130=CARTESIAN_POINT('Ctrl Pts',(14.0300605393523,0.506951282871708,26.3523401989906));
#48131=CARTESIAN_POINT('Ctrl Pts',(13.8911490488636,3.48368054963307,25.3360280579309));
#48132=CARTESIAN_POINT('Ctrl Pts',(13.752237558375,5.6116651230563,23.0196755046844));
#48133=CARTESIAN_POINT('Ctrl Pts',(13.6133260678864,6.37245459172572,19.967625885163));
#48134=CARTESIAN_POINT('Ctrl Pts',(13.4744145773977,5.58069441033177,16.9234637162209));
#48135=CARTESIAN_POINT('Ctrl Pts',(13.3355030869091,3.42928465762181,14.6288518598053));
#48136=CARTESIAN_POINT('Ctrl Pts',(13.1965915964205,0.442382926346631,13.6428368784973));
#48137=CARTESIAN_POINT('Ctrl Pts',(13.0576801059318,-2.65229853840607,14.205646017882));
#48138=CARTESIAN_POINT('Ctrl Pts',(12.9187686154432,-5.10078863240939,16.1801595668928));
#48139=CARTESIAN_POINT('Ctrl Pts',(12.7798571249545,-6.30655074894272,19.0853179470835));
#48140=CARTESIAN_POINT('Ctrl Pts',(12.6409456344659,-5.97581966376832,22.2133244120638));
#48141=CARTESIAN_POINT('Ctrl Pts',(12.5020341439773,-4.1891728722864,24.8020887385612));
#48142=CARTESIAN_POINT('Ctrl Pts',(12.3631226534886,-1.38189913347912,26.2208986804004));
#48143=CARTESIAN_POINT('Ctrl Pts',(12.224211163,1.76205287980219,26.124083217568));
#48144=CARTESIAN_POINT('Ctrl Pts',(12.0852996725114,4.4767080589433,24.5352299348445));
#48145=CARTESIAN_POINT('Ctrl Pts',(11.9463881820227,6.1006828055596,21.8414382728907));
#48146=CARTESIAN_POINT('Ctrl Pts',(11.8074766915341,6.23832087945686,18.6990087579656));
#48147=CARTESIAN_POINT('Ctrl Pts',(11.6685652010455,4.85608890030431,15.8735455655904));
#48148=CARTESIAN_POINT('Ctrl Pts',(11.5296537105568,2.29074623525794,14.0534289466476));
#48149=CARTESIAN_POINT('Ctrl Pts',(11.3907422200682,-0.832701193775514,
13.6821020640721));
#48150=CARTESIAN_POINT('Ctrl Pts',(11.2518307295795,-3.75327390186831,14.8500329491858));
#48151=CARTESIAN_POINT('Ctrl Pts',(11.1129192390909,-5.75941968089301,17.272673370082));
#48152=CARTESIAN_POINT('Ctrl Pts',(10.9740077486023,-6.36237225054617,20.3597845916624));
#48153=CARTESIAN_POINT('Ctrl Pts',(10.8350962581136,-5.41523157606947,23.3592398819462));
#48154=CARTESIAN_POINT('Ctrl Pts',(10.696184767625,-3.14875378158332,25.5402685160452));
#48155=CARTESIAN_POINT('Ctrl Pts',(10.5572732771364,-0.115131002167762,
26.3714967204933));
#48156=CARTESIAN_POINT('Ctrl Pts',(10.4183617866477,2.94654165889923,25.6504086453361));
#48157=CARTESIAN_POINT('Ctrl Pts',(10.2794502961591,5.29033518005657,23.5526862075862));
#48158=CARTESIAN_POINT('Ctrl Pts',(10.1405388056704,6.34522064949098,20.5894069190218));
#48159=CARTESIAN_POINT('Ctrl Pts',(10.0016273151818,5.854191596171,17.4825277832241));
#48160=CARTESIAN_POINT('Ctrl Pts',(9.86271582469318,3.9368796273414,14.9889916776419));
#48161=CARTESIAN_POINT('Ctrl Pts',(9.72380433420454,1.06040804430175,13.716309970527));
#48162=CARTESIAN_POINT('Ctrl Pts',(9.58489284371591,-2.07441549941601,13.974551805658));
#48163=CARTESIAN_POINT('Ctrl Pts',(9.44598135322726,-4.70383990511773,15.7008005682523));
#48164=CARTESIAN_POINT('Ctrl Pts',(9.30706986273865,-6.18724672944247,18.4744825415877));
#48165=CARTESIAN_POINT('Ctrl Pts',(9.16815837224999,-6.16322692461181,21.6198331650691));
#48166=CARTESIAN_POINT('Ctrl Pts',(9.02924688176137,-4.63763254324486,24.3705365804159));
#48167=CARTESIAN_POINT('Ctrl Pts',(8.89033539127272,-1.98215097657166,26.0564265960212));
#48168=CARTESIAN_POINT('Ctrl Pts',(8.7514239007841,1.15625090922707,26.2667622774308));
#48169=CARTESIAN_POINT('Ctrl Pts',(8.61251241029546,4.01295020795098,24.9502986006324));
#48170=CARTESIAN_POINT('Ctrl Pts',(8.47360091980683,5.8919564762427,22.4277715067483));
#48171=CARTESIAN_POINT('Ctrl Pts',(8.33468942931819,6.33547900216983,19.3137555683411));
#48172=CARTESIAN_POINT('Ctrl Pts',(8.19577793882954,5.23546040650557,16.3669324340401));
#48173=CARTESIAN_POINT('Ctrl Pts',(8.05686644834092,2.85990314594527,14.3052498208675));
#48174=CARTESIAN_POINT('Ctrl Pts',(7.91795495785227,-0.212425125618811,
13.6310046967419));
#48175=CARTESIAN_POINT('Ctrl Pts',(7.77904346736364,-3.23299931252101,14.5084664207386));
#48176=CARTESIAN_POINT('Ctrl Pts',(7.64013197687499,-5.46590339851313,16.7238550634869));
#48177=CARTESIAN_POINT('Ctrl Pts',(7.50122048638637,-6.3671249614693,19.7374255687385));
#48178=CARTESIAN_POINT('Ctrl Pts',(7.36230899589772,-5.71709535604924,22.8149682585701));
#48179=CARTESIAN_POINT('Ctrl Pts',(7.2233975054091,-3.67418420606118,25.206687625242));
#48180=CARTESIAN_POINT('Ctrl Pts',(7.08448601492046,-0.73611510378342,26.3298783685707));
#48181=CARTESIAN_POINT('Ctrl Pts',(6.94557452443182,2.38129701778703,25.9108924977533));
#48182=CARTESIAN_POINT('Ctrl Pts',(6.80666303394318,4.91854308270761,24.0518094168491));
#48183=CARTESIAN_POINT('Ctrl Pts',(6.66775154345454,6.2574624695857,21.2055658624248));
#48184=CARTESIAN_POINT('Ctrl Pts',(6.5288400529659,6.07184825208871,18.0656048980302));
#48185=CARTESIAN_POINT('Ctrl Pts',(6.38992856247727,4.40692245326515,15.3969292751659));
#48186=CARTESIAN_POINT('Ctrl Pts',(6.25101707198863,1.66831840155036,13.8497203870096));
#48187=CARTESIAN_POINT('Ctrl Pts',(6.11210558150001,-1.47674553359532,13.8009316638769));
#48188=CARTESIAN_POINT('Ctrl Pts',(5.97319409101137,-4.26202334105436,15.2624497208763));
#48189=CARTESIAN_POINT('Ctrl Pts',(5.83428260052273,-6.0089253152344,17.8781983686375));
#48190=CARTESIAN_POINT('Ctrl Pts',(5.6953711100341,-6.29184590498261,21.0108910499511));
#48191=CARTESIAN_POINT('Ctrl Pts',(5.55645961954546,-5.04185590001004,23.897295817673));
#48192=CARTESIAN_POINT('Ctrl Pts',(5.41754812905682,-2.56349596308158,25.8341849520033));
#48193=CARTESIAN_POINT('Ctrl Pts',(5.27863663856818,0.539419975483812,26.3496654791388));
#48194=CARTESIAN_POINT('Ctrl Pts',(5.13972514807955,3.51091460972764,25.3181485697674));
#48195=CARTESIAN_POINT('Ctrl Pts',(5.00081365759091,5.62702939460967,22.9909473079805));
#48196=CARTESIAN_POINT('Ctrl Pts',(4.86190216710228,6.37220580845331,19.9350481591359));
#48197=CARTESIAN_POINT('Ctrl Pts',(4.72299067661364,5.56489318441634,16.8949735181558));
#48198=CARTESIAN_POINT('Ctrl Pts',(4.584079186125,3.40178071249615,14.6113903842451));
#48199=CARTESIAN_POINT('Ctrl Pts',(4.44516769563636,0.409877171332637,13.6406583429304));
#48200=CARTESIAN_POINT('Ctrl Pts',(4.30625620514773,-2.68188658064232,14.2192811886858));
#48201=CARTESIAN_POINT('Ctrl Pts',(4.16734471465908,-5.12025029463462,16.2062864463399));
#48202=CARTESIAN_POINT('Ctrl Pts',(4.02843322417046,-6.31114449923059,19.1175711265328));
#48203=CARTESIAN_POINT('Ctrl Pts',(3.88952173368181,-5.96442630616995,22.24384590496));
#48204=CARTESIAN_POINT('Ctrl Pts',(3.75061024319318,-4.16456822152471,24.8234424569172));
#48205=CARTESIAN_POINT('Ctrl Pts',(3.61169875270454,-1.35007773082975,26.2278821221607));
#48206=CARTESIAN_POINT('Ctrl Pts',(3.47278726221591,1.79333824355105,26.1149949755885));
#48207=CARTESIAN_POINT('Ctrl Pts',(3.33387577172728,4.49983519042547,24.5122842181282));
#48208=CARTESIAN_POINT('Ctrl Pts',(3.19496428123863,6.11001713833909,21.8102254493376));
#48209=CARTESIAN_POINT('Ctrl Pts',(3.05605279075,6.23158824788668,18.6671333472082));
#48210=CARTESIAN_POINT('Ctrl Pts',(2.91714130026136,4.83492960625386,15.8487735173902));
#48211=CARTESIAN_POINT('Ctrl Pts',(2.77822980977273,2.26031541093747,14.041795584685));
#48212=CARTESIAN_POINT('Ctrl Pts',(2.63931831928409,-0.864989547684349,
13.6864416790982));
#48213=CARTESIAN_POINT('Ctrl Pts',(2.50040682879546,-3.77955323437126,14.8692882560822));
#48214=CARTESIAN_POINT('Ctrl Pts',(2.36149533830682,-5.7732874301525,17.3021531225892));
#48215=CARTESIAN_POINT('Ctrl Pts',(2.22258384781818,-6.36044977513704,20.3923064851901));
#48216=CARTESIAN_POINT('Ctrl Pts',(2.08367235732954,-5.39798721704175,23.3868805022452));
#48217=CARTESIAN_POINT('Ctrl Pts',(1.94476086684091,-3.12038893862028,25.556293575601));
#48218=CARTESIAN_POINT('Ctrl Pts',(1.80584937635227,-0.0825561728535726,
26.3720021186908));
#48219=CARTESIAN_POINT('Ctrl Pts',(1.66693788586364,2.97538981548086,25.6352709416678));
#48220=CARTESIAN_POINT('Ctrl Pts',(1.528026395375,5.30842886408474,23.5255940754177));
#48221=CARTESIAN_POINT('Ctrl Pts',(1.38911490488636,6.34815042253135,20.5569597405651));
#48222=CARTESIAN_POINT('Ctrl Pts',(1.25020341439772,5.84124601468089,17.4526331642158));
#48223=CARTESIAN_POINT('Ctrl Pts',(1.11129192390908,3.91120805214414,14.9689283406313));
#48224=CARTESIAN_POINT('Ctrl Pts',(0.972380433420452,1.02827407433471,13.7109751703986));
#48225=CARTESIAN_POINT('Ctrl Pts',(0.833468942931815,-2.10520088120389,
13.985227291767));
#48226=CARTESIAN_POINT('Ctrl Pts',(0.694557452443171,-4.72574094137507,
15.7249208643558));
#48227=CARTESIAN_POINT('Ctrl Pts',(0.555645961954543,-6.19499726498531,
18.5061012876301));
#48228=CARTESIAN_POINT('Ctrl Pts',(0.416734471465905,-6.15480127088778,
21.6513846776137));
#48229=CARTESIAN_POINT('Ctrl Pts',(0.277822980977271,-4.61535544548857,
24.3940602366606));
#48230=CARTESIAN_POINT('Ctrl Pts',(0.138911490488638,-1.95089886648438,
26.0667560931559));
#48231=CARTESIAN_POINT('Ctrl Pts',(0.0463038301628798,0.141429157467205,
26.1955412757171));
#48232=CARTESIAN_POINT('Ctrl Pts',(0.,1.1399249411295,26.0060300274883));
#48233=CARTESIAN_POINT('Ctrl Pts',(0.,1.1399249411295,26.0060300274883));
#48234=CARTESIAN_POINT('Ctrl Pts',(-4.24882758481919E-16,0.972331625605204,
26.024339235968));
#48235=CARTESIAN_POINT('Ctrl Pts',(-9.68713354198481E-15,0.804333349730088,
26.0355246893388));
#48236=CARTESIAN_POINT('Ctrl Pts',(-7.21644966006352E-15,0.636361653837589,
26.0397009622082));
#48237=CARTESIAN_POINT('Ctrl Pts',(-4.72622945714007E-15,0.467061763353201,
26.0439102579212));
#48238=CARTESIAN_POINT('Ctrl Pts',(7.46066107244459E-15,0.297788121924876,
26.0409989699337));
#48239=CARTESIAN_POINT('Ctrl Pts',(6.88338275267597E-15,0.128984633759083,
26.0310315656805));
#48240=CARTESIAN_POINT('Ctrl Pts',(6.30997977578734E-15,-0.038685655092656,
26.0211310738815));
#48241=CARTESIAN_POINT('Ctrl Pts',(-8.19789119918948E-15,-0.205892792351831,
26.0042686578037));
#48242=CARTESIAN_POINT('Ctrl Pts',(-7.105427357601E-15,-0.372188805166806,
25.9804583393351));
#48243=CARTESIAN_POINT('Ctrl Pts',(-6.02607596443286E-15,-0.536488827077978,
25.9569338075084));
#48244=CARTESIAN_POINT('Ctrl Pts',(1.21781657491819E-14,-0.699900099394016,
25.9266269150383));
#48245=CARTESIAN_POINT('Ctrl Pts',(1.3988810110277E-14,-0.861967977673184,
25.8895065880249));
#48246=CARTESIAN_POINT('Ctrl Pts',(1.48816567000726E-14,-0.941885246655507,
25.8712021887192));
#48247=CARTESIAN_POINT('Ctrl Pts',(-8.6069672340652E-15,-1.02147545165873,
25.8512403873111));
#48248=CARTESIAN_POINT('Ctrl Pts',(-8.60422844084496E-15,-1.10068130521252,
25.8296136588393));
#48249=CARTESIAN_POINT('Ctrl Pts',(-8.60343716793459E-15,-1.12356490438221,
25.8233654162727));
#48250=CARTESIAN_POINT('Ctrl Pts',(1.17899233680487E-14,-1.14641640818171,
25.8169781854097));
#48251=CARTESIAN_POINT('Ctrl Pts',(1.21569421196455E-14,-1.16923440163958,
25.8104517468483));
#48252=CARTESIAN_POINT('Ctrl Pts',(1.24890717527468E-14,-1.18988329699519,
25.8045457171552));
#48253=CARTESIAN_POINT('Ctrl Pts',(-4.94407272871347E-15,-1.21049718097962,
25.7985278328021));
#48254=CARTESIAN_POINT('Ctrl Pts',(-4.94049245958195E-15,-1.23107002624393,
25.7923997285709));
#48255=CARTESIAN_POINT('Ctrl Pts',(-4.91294908986661E-15,-1.38933898938462,
25.7452556077536));
#48256=CARTESIAN_POINT('Ctrl Pts',(-6.72206345910563E-15,-1.54527720466299,
25.6915646759272));
#48257=CARTESIAN_POINT('Ctrl Pts',(-5.71764857681956E-15,-1.69847023449156,
25.6313756857849));
#48258=CARTESIAN_POINT('Ctrl Pts',(-5.49877947596065E-15,-1.73185207827719,
25.6182600794887));
#48259=CARTESIAN_POINT('Ctrl Pts',(1.85007413129516E-16,-1.76510349913815,
25.6048357400391));
#48260=CARTESIAN_POINT('Ctrl Pts',(4.44089209850063E-16,-1.79822007618261,
25.5911028699638));
#48261=CARTESIAN_POINT('Ctrl Pts',(1.63842330494031E-15,-1.95076548408182,
25.5278449352909));
#48262=CARTESIAN_POINT('Ctrl Pts',(7.40213603062554E-15,-2.10045211587673,
25.45804398787));
#48263=CARTESIAN_POINT('Ctrl Pts',(8.27116153345742E-15,-2.24691457271093,
25.3819733194664));
#48264=CARTESIAN_POINT('Ctrl Pts',(9.13853574229822E-15,-2.39309872634908,
25.3060471980723));
#48265=CARTESIAN_POINT('Ctrl Pts',(-3.10245225034387E-15,-2.53607151765369,
25.2238746247319));
#48266=CARTESIAN_POINT('Ctrl Pts',(-5.05151476204446E-15,-2.67543507353407,
25.1356889048841));
#48267=CARTESIAN_POINT('Ctrl Pts',(-6.91182822640314E-15,-2.80845281816195,
25.0515186532825));
#48268=CARTESIAN_POINT('Ctrl Pts',(2.53114930940398E-15,-2.9381827322964,
24.9618697543865));
#48269=CARTESIAN_POINT('Ctrl Pts',(3.88578058618805E-15,-3.064242236503,
24.866918929929));
#48270=CARTESIAN_POINT('Ctrl Pts',(4.27484187305284E-15,-3.10044756688972,
24.8396482692071));
#48271=CARTESIAN_POINT('Ctrl Pts',(-4.44149303582884E-16,-3.13634988015047,
24.8119401207576));
#48272=CARTESIAN_POINT('Ctrl Pts',(-8.88178419700125E-16,-3.17193948309244,
24.7837983555989));
#48273=CARTESIAN_POINT('Ctrl Pts',(-1.0931195317057E-15,-3.18836582212746,
24.770809557261));
#48274=CARTESIAN_POINT('Ctrl Pts',(7.56942218681223E-15,-3.20471920206644,
24.757733375776));
#48275=CARTESIAN_POINT('Ctrl Pts',(7.27196081129478E-15,-3.22099520798022,
24.7445733686326));
#48276=CARTESIAN_POINT('Ctrl Pts',(4.97510987807207E-15,-3.34667054753367,
24.6429582441954));
#48277=CARTESIAN_POINT('Ctrl Pts',(-7.27529725750927E-15,-3.46780653688132,
24.536292406256));
#48278=CARTESIAN_POINT('Ctrl Pts',(-8.32667268468867E-15,-3.58406520205367,
24.4248373445186));
#48279=CARTESIAN_POINT('Ctrl Pts',(-9.36930803468661E-15,-3.69935740968825,
24.3143088079944));
#48280=CARTESIAN_POINT('Ctrl Pts',(-7.79923338847808E-15,-3.8098535192748,
24.1990697852018));
#48281=CARTESIAN_POINT('Ctrl Pts',(-4.55191440096314E-15,-3.91518516086881,
24.0793423741378));
#48282=CARTESIAN_POINT('Ctrl Pts',(-2.81924743660761E-15,-3.97138680178951,
24.0154596047899));
#48283=CARTESIAN_POINT('Ctrl Pts',(-9.87932414299166E-15,-4.02611744048476,
23.9502985023543));
#48284=CARTESIAN_POINT('Ctrl Pts',(-9.76996261670138E-15,-4.07931584475367,
23.8838897354569));
#48285=CARTESIAN_POINT('Ctrl Pts',(-9.55902562552653E-15,-4.17974198312324,
23.7585255237847));
#48286=CARTESIAN_POINT('Ctrl Pts',(-1.21509664281812E-14,-4.27471073087482,
23.628715679372));
#48287=CARTESIAN_POINT('Ctrl Pts',(-1.31006316905768E-14,-4.36398437993495,
23.4948506002188));
#48288=CARTESIAN_POINT('Ctrl Pts',(-1.36609359328008E-14,-4.41665599620636,
23.4158699586126));
#48289=CARTESIAN_POINT('Ctrl Pts',(7.87054257710942E-15,-4.46734420575991,
23.3354773858304));
#48290=CARTESIAN_POINT('Ctrl Pts',(7.49400541621981E-15,-4.51599174705983,
23.2537516282698));
#48291=CARTESIAN_POINT('Ctrl Pts',(7.35114473953617E-15,-4.53444894435924,
23.2227443380464));
#48292=CARTESIAN_POINT('Ctrl Pts',(-7.55359812461929E-15,-4.55261232233179,
23.1915451316209));
#48293=CARTESIAN_POINT('Ctrl Pts',(-8.02136135291676E-15,-4.57047850650274,
23.1601583000966));
#48294=CARTESIAN_POINT('Ctrl Pts',(-8.37371801685389E-15,-4.58393674492536,
23.1365152290332));
#48295=CARTESIAN_POINT('Ctrl Pts',(1.01309155042277E-14,-4.59722854667126,
23.1127615325227));
#48296=CARTESIAN_POINT('Ctrl Pts',(1.00475183728577E-14,-4.61033840937547,
23.0889249821437));
#48297=CARTESIAN_POINT('Ctrl Pts',(9.56418682075062E-15,-4.68631716529486,
22.9507792605549));
#48298=CARTESIAN_POINT('Ctrl Pts',(2.3597456518294E-14,-4.75627611708813,
22.8097036647301));
#48299=CARTESIAN_POINT('Ctrl Pts',(2.0344836926256E-14,-4.82005887673718,
22.6660968272704));
#48300=CARTESIAN_POINT('Ctrl Pts',(1.71010815115263E-14,-4.88366781289573,
22.5228813532745));
#48301=CARTESIAN_POINT('Ctrl Pts',(1.36041559436968E-15,-4.94113438033816,
22.3771476702801));
#48302=CARTESIAN_POINT('Ctrl Pts',(1.11022302462516E-15,-4.99225431533367,
22.2292753801568));
#48303=CARTESIAN_POINT('Ctrl Pts',(8.64348697063786E-16,-5.04249193691787,
22.08395531755));
#48304=CARTESIAN_POINT('Ctrl Pts',(-1.64081607249733E-14,-5.08660018806323,
21.9365691476464));
#48305=CARTESIAN_POINT('Ctrl Pts',(-1.94566585065559E-14,-5.12433580930953,
21.7874725054075));
#48306=CARTESIAN_POINT('Ctrl Pts',(-2.2091841268231E-14,-5.15695523885615,
21.6585903707951));
#48307=CARTESIAN_POINT('Ctrl Pts',(-7.63174605915859E-15,-5.18481220829848,
21.5284298183699));
#48308=CARTESIAN_POINT('Ctrl Pts',(-7.52176099183544E-15,-5.20771827252021,
21.3972234452764));
#48309=CARTESIAN_POINT('Ctrl Pts',(-7.50414181272803E-15,-5.21716825578637,
21.3430937607464));
#48310=CARTESIAN_POINT('Ctrl Pts',(-4.48361323931463E-15,-5.22577522782904,
21.2887861341176));
#48311=CARTESIAN_POINT('Ctrl Pts',(-4.30211422042248E-15,-5.2335367160805,
21.2343205788571));
#48312=CARTESIAN_POINT('Ctrl Pts',(-4.19823060416723E-15,-5.23797911732325,
21.2031464222344));
#48313=CARTESIAN_POINT('Ctrl Pts',(-1.42660523996842E-14,-5.24214452334437,
21.1719205330544));
#48314=CARTESIAN_POINT('Ctrl Pts',(-1.46271883494364E-14,-5.24603236151472,
21.1406467100027));
#48315=CARTESIAN_POINT('Ctrl Pts',(-1.48771345015575E-14,-5.24872317695809,
21.1190017540263));
#48316=CARTESIAN_POINT('Ctrl Pts',(-6.99848150814512E-16,-5.2512806964718,
21.0973361625274));
#48317=CARTESIAN_POINT('Ctrl Pts',(-1.16573417585641E-15,-5.25370371263287,
21.0756621094304));
#48318=CARTESIAN_POINT('Ctrl Pts',(-4.46481939510917E-15,-5.27086185083263,
20.9221813343688));
#48319=CARTESIAN_POINT('Ctrl Pts',(-7.07482054458005E-15,-5.28129916922496,
20.7681211137086));
#48320=CARTESIAN_POINT('Ctrl Pts',(-4.09394740330526E-15,-5.28504682504941,
20.6139250846838));
#48321=CARTESIAN_POINT('Ctrl Pts',(-1.11160171993656E-15,-5.28879633220422,
20.4596528832985));
#48322=CARTESIAN_POINT('Ctrl Pts',(6.57889777690792E-15,-5.28584942273906,
20.305243947736));
#48323=CARTESIAN_POINT('Ctrl Pts',(9.49240686054509E-15,-5.27618637882583,
20.1511539648283));
#48324=CARTESIAN_POINT('Ctrl Pts',(1.0584972766909E-14,-5.27256273735838,
20.093370221238));
#48325=CARTESIAN_POINT('Ctrl Pts',(-8.75513436052681E-15,-5.26799413779765,
20.0356315059054));
#48326=CARTESIAN_POINT('Ctrl Pts',(-9.64506252643105E-15,-5.26247775735231,
19.9779626095996));
#48327=CARTESIAN_POINT('Ctrl Pts',(-1.01099037057859E-14,-5.25959635535805,
19.9478400909538));
#48328=CARTESIAN_POINT('Ctrl Pts',(-4.21799155701331E-16,-5.25645635018643,
19.9177366294551));
#48329=CARTESIAN_POINT('Ctrl Pts',(-1.33226762955019E-15,-5.25305723633443,
19.887655815811));
#48330=CARTESIAN_POINT('Ctrl Pts',(-2.13988741696045E-15,-5.25004209447572,
19.8609730024922));
#48331=CARTESIAN_POINT('Ctrl Pts',(-1.97866480786439E-17,-5.24682284854293,
19.8343067979969));
#48332=CARTESIAN_POINT('Ctrl Pts',(2.77555756156289E-17,-5.24340155368231,
19.8076771713483));
#48333=CARTESIAN_POINT('Ctrl Pts',(2.95714117697871E-16,-5.22411837524327,
19.6575866753963));
#48334=CARTESIAN_POINT('Ctrl Pts',(-1.67002099626319E-14,-5.19840717094589,
19.5085293113512));
#48335=CARTESIAN_POINT('Ctrl Pts',(-1.40998324127395E-14,-5.16626585321672,
19.3609354592565));
#48336=CARTESIAN_POINT('Ctrl Pts',(-1.15393273258269E-14,-5.13461736911524,
19.2156047133035));
#48337=CARTESIAN_POINT('Ctrl Pts',(-3.45941278228998E-15,-5.09673418838306,
19.0716922997645));
#48338=CARTESIAN_POINT('Ctrl Pts',(-2.55004350968591E-15,-5.05256917177841,
18.9296313323074));
#48339=CARTESIAN_POINT('Ctrl Pts',(-2.25598581474793E-15,-5.0382877754624,
18.8836938656593));
#48340=CARTESIAN_POINT('Ctrl Pts',(-1.39822119446523E-14,-5.02334918104501,
18.8379502101177));
#48341=CARTESIAN_POINT('Ctrl Pts',(-1.50521956010508E-14,-5.00775082964022,
18.7924156868194));
#48342=CARTESIAN_POINT('Ctrl Pts',(-1.61762705543893E-14,-4.99145691331742,
18.7448506786229));
#48343=CARTESIAN_POINT('Ctrl Pts',(-8.99370074056487E-17,-4.97444308272645,
18.697513865944));
#48344=CARTESIAN_POINT('Ctrl Pts',(8.32667268468867E-17,-4.95671627827806,
18.6504206457069));
#48345=CARTESIAN_POINT('Ctrl Pts',(50.,3.87994761181434,23.3663343702128));
#48346=CARTESIAN_POINT('Ctrl Pts',(50.,3.98673757809611,23.2643222420238));
#48347=CARTESIAN_POINT('Ctrl Pts',(50.,4.08880253645321,23.1578171274895));
#48348=CARTESIAN_POINT('Ctrl Pts',(50.,4.18601999315063,23.0472591141687));
#48349=CARTESIAN_POINT('Ctrl Pts',(50.,4.28495878527548,22.9347435570942));
#48350=CARTESIAN_POINT('Ctrl Pts',(50.,4.37887739050272,22.8180299104541));
#48351=CARTESIAN_POINT('Ctrl Pts',(50.,4.46762356605889,22.6975330565356));
#48352=CARTESIAN_POINT('Ctrl Pts',(50.,4.55766271640646,22.5752806408298));
#48353=CARTESIAN_POINT('Ctrl Pts',(50.,4.64237816685758,22.4491334930856));
#48354=CARTESIAN_POINT('Ctrl Pts',(50.,4.72157940439616,22.3194816713432));
#48355=CARTESIAN_POINT('Ctrl Pts',(50.,4.80065560169515,22.1900345395192));
#48356=CARTESIAN_POINT('Ctrl Pts',(50.,4.87423546656432,22.0570931764291));
#48357=CARTESIAN_POINT('Ctrl Pts',(50.,4.94209057403842,21.9210114696859));
#48358=CARTESIAN_POINT('Ctrl Pts',(50.,4.96154268599091,21.8820007497446));
#48359=CARTESIAN_POINT('Ctrl Pts',(50.,4.98052406523496,21.8427317710976));
#48360=CARTESIAN_POINT('Ctrl Pts',(50.,4.99902865333407,21.8032124599192));
#48361=CARTESIAN_POINT('Ctrl Pts',(50.,5.00999309769487,21.7797962516647));
#48362=CARTESIAN_POINT('Ctrl Pts',(50.,5.02079014100455,21.756292151844));
#48363=CARTESIAN_POINT('Ctrl Pts',(50.,5.03141846895726,21.73270178382));
#48364=CARTESIAN_POINT('Ctrl Pts',(50.,5.03934295940047,21.7151127851751));
#48365=CARTESIAN_POINT('Ctrl Pts',(50.,5.04717318872179,21.6974767538246));
#48366=CARTESIAN_POINT('Ctrl Pts',(50.,5.05490365729456,21.6798060792548));
#48367=CARTESIAN_POINT('Ctrl Pts',(50.,5.11733467588189,21.5370982728475));
#48368=CARTESIAN_POINT('Ctrl Pts',(50.,5.17335281141187,21.3919340172648));
#48369=CARTESIAN_POINT('Ctrl Pts',(50.,5.22279492351638,21.2447432489076));
#48370=CARTESIAN_POINT('Ctrl Pts',(50.,5.23314291494296,21.2139369434283));
#48371=CARTESIAN_POINT('Ctrl Pts',(50.,5.24320272739019,21.1830417306106));
#48372=CARTESIAN_POINT('Ctrl Pts',(50.,5.2529726674319,21.1520613441281));
#48373=CARTESIAN_POINT('Ctrl Pts',(50.,5.2991582979104,21.0056071513642));
#48374=CARTESIAN_POINT('Ctrl Pts',(50.,5.33886957351671,20.857251867747));
#48375=CARTESIAN_POINT('Ctrl Pts',(50.,5.37217407103346,20.7074371580895));
#48376=CARTESIAN_POINT('Ctrl Pts',(50.,5.40587044985943,20.5558596359311));
#48377=CARTESIAN_POINT('Ctrl Pts',(50.,5.43300860662334,20.4027874704091));
#48378=CARTESIAN_POINT('Ctrl Pts',(50.,5.45361092314426,20.2486538959499));
#48379=CARTESIAN_POINT('Ctrl Pts',(50.,5.47374677556284,20.0980101125235));
#48380=CARTESIAN_POINT('Ctrl Pts',(50.,5.48763934473341,19.9463517039926));
#48381=CARTESIAN_POINT('Ctrl Pts',(50.,5.4952635449959,19.794070763421));
#48382=CARTESIAN_POINT('Ctrl Pts',(50.,5.49686470975424,19.7620901140394));
#48383=CARTESIAN_POINT('Ctrl Pts',(50.,5.49818924741761,19.7300819857573));
#48384=CARTESIAN_POINT('Ctrl Pts',(50.,5.49923666289681,19.6980499851575));
#48385=CARTESIAN_POINT('Ctrl Pts',(50.,5.49987642324748,19.6784848705075));
#48386=CARTESIAN_POINT('Ctrl Pts',(50.,5.50041270196756,19.6589123700862));
#48387=CARTESIAN_POINT('Ctrl Pts',(50.,5.50084527831566,19.6393453886745));
#48388=CARTESIAN_POINT('Ctrl Pts',(50.,5.50435921646177,19.4803973493558));
#48389=CARTESIAN_POINT('Ctrl Pts',(50.,5.50104151508177,19.3215990804738));
#48390=CARTESIAN_POINT('Ctrl Pts',(50.,5.4909705479201,19.1634131964696));
#48391=CARTESIAN_POINT('Ctrl Pts',(50.,5.48078634391211,19.0034486877963));
#48392=CARTESIAN_POINT('Ctrl Pts',(50.,5.46369634889609,18.8441096739535));
#48393=CARTESIAN_POINT('Ctrl Pts',(50.,5.43973189107444,18.6858559372003));
#48394=CARTESIAN_POINT('Ctrl Pts',(50.,5.42686001032611,18.6008540881027));
#48395=CARTESIAN_POINT('Ctrl Pts',(50.,5.41200396913525,18.5161650932381));
#48396=CARTESIAN_POINT('Ctrl Pts',(50.,5.39516250342907,18.4318591808605));
#48397=CARTESIAN_POINT('Ctrl Pts',(50.,5.36396597336624,18.2756939173468));
#48398=CARTESIAN_POINT('Ctrl Pts',(50.,5.32596009918743,18.1208426670828));
#48399=CARTESIAN_POINT('Ctrl Pts',(50.,5.28136854987424,17.9676705715706));
#48400=CARTESIAN_POINT('Ctrl Pts',(50.,5.25350309477334,17.8719526560474));
#48401=CARTESIAN_POINT('Ctrl Pts',(50.,5.22306483730966,17.7768905017353));
#48402=CARTESIAN_POINT('Ctrl Pts',(50.,5.19009824063749,17.6825750879815));
#48403=CARTESIAN_POINT('Ctrl Pts',(50.,5.17761685929209,17.6468666204828));
#48404=CARTESIAN_POINT('Ctrl Pts',(50.,5.16477298038166,17.6112652149274));
#48405=CARTESIAN_POINT('Ctrl Pts',(50.,5.15156873790798,17.5757759000135));
#48406=CARTESIAN_POINT('Ctrl Pts',(50.,5.14404034706544,17.5555416886274));
#48407=CARTESIAN_POINT('Ctrl Pts',(50.,5.13639438080441,17.5353429478627));
#48408=CARTESIAN_POINT('Ctrl Pts',(50.,5.12863752106129,17.5151965619237));
#48409=CARTESIAN_POINT('Ctrl Pts',(50.,5.07015508167858,17.3633039361097));
#48410=CARTESIAN_POINT('Ctrl Pts',(50.,5.00529636697242,17.2141769687293));
#48411=CARTESIAN_POINT('Ctrl Pts',(50.,4.93436661664131,17.0681831171989));
#48412=CARTESIAN_POINT('Ctrl Pts',(50.,4.86274846547203,16.9207723385076));
#48413=CARTESIAN_POINT('Ctrl Pts',(50.,4.78494068080824,16.7765550865127));
#48414=CARTESIAN_POINT('Ctrl Pts',(50.,4.70120368491443,16.6359121753525));
#48415=CARTESIAN_POINT('Ctrl Pts',(50.,4.61735315197323,16.4950785697364));
#48416=CARTESIAN_POINT('Ctrl Pts',(50.,4.52755705979088,16.3578282816204));
#48417=CARTESIAN_POINT('Ctrl Pts',(50.,4.43202664990479,16.2245569418224));
#48418=CARTESIAN_POINT('Ctrl Pts',(50.,4.34556725909594,16.1039402830544));
#48419=CARTESIAN_POINT('Ctrl Pts',(50.,4.25441008172596,15.9865825841098));
#48420=CARTESIAN_POINT('Ctrl Pts',(50.,4.15867898536816,15.8727940124341));
#48421=CARTESIAN_POINT('Ctrl Pts',(50.,4.11861293335795,15.8251704188017));
#48422=CARTESIAN_POINT('Ctrl Pts',(50.,4.07774532870654,15.7781722486037));
#48423=CARTESIAN_POINT('Ctrl Pts',(50.,4.03609486664093,15.7318124329449));
#48424=CARTESIAN_POINT('Ctrl Pts',(50.,4.01339708741421,15.7065482507815));
#48425=CARTESIAN_POINT('Ctrl Pts',(50.,3.9904668008218,15.6814736593072));
#48426=CARTESIAN_POINT('Ctrl Pts',(50.,3.96730693292679,15.6565908429678));
#48427=CARTESIAN_POINT('Ctrl Pts',(50.,3.95229484852802,15.6404619539491));
#48428=CARTESIAN_POINT('Ctrl Pts',(50.,3.93719275896563,15.6244205832957));
#48429=CARTESIAN_POINT('Ctrl Pts',(50.,3.92200238339549,15.6084678404505));
#48430=CARTESIAN_POINT('Ctrl Pts',(50.,3.80788414784779,15.4886222936937));
#48431=CARTESIAN_POINT('Ctrl Pts',(50.,3.68877507270694,15.3737638929061));
#48432=CARTESIAN_POINT('Ctrl Pts',(50.,3.56510260126303,15.2640814626229));
#48433=CARTESIAN_POINT('Ctrl Pts',(50.,3.43994735694197,15.1530839932624));
#48434=CARTESIAN_POINT('Ctrl Pts',(50.,3.31011817858053,15.0473868234606));
#48435=CARTESIAN_POINT('Ctrl Pts',(50.,3.17601311849488,14.947214065385));
#48436=CARTESIAN_POINT('Ctrl Pts',(50.,3.12100973291315,14.9061280628605));
#48437=CARTESIAN_POINT('Ctrl Pts',(50.,3.06528655998735,14.8659717741899));
#48438=CARTESIAN_POINT('Ctrl Pts',(50.,3.00886919673059,14.8267623442652));
#48439=CARTESIAN_POINT('Ctrl Pts',(50.,2.96664655543823,14.7974180856998));
#48440=CARTESIAN_POINT('Ctrl Pts',(50.,2.92403507641734,14.7686041826055));
#48441=CARTESIAN_POINT('Ctrl Pts',(50.,2.88104513961241,14.7403282232461));
#48442=CARTESIAN_POINT('Ctrl Pts',(50.,2.85826547946661,14.7253452576412));
#48443=CARTESIAN_POINT('Ctrl Pts',(50.,2.8353875118122,14.7105185891356));
#48444=CARTESIAN_POINT('Ctrl Pts',(50.,2.81241516289751,14.6958504281824));
#48445=CARTESIAN_POINT('Ctrl Pts',(50.,2.66893410381596,14.6042357972118));
#48446=CARTESIAN_POINT('Ctrl Pts',(50.,2.52174774822922,14.518784282482));
#48447=CARTESIAN_POINT('Ctrl Pts',(50.,2.3712759493438,14.4397157364412));
#48448=CARTESIAN_POINT('Ctrl Pts',(50.,2.22051092714072,14.3604931100906));
#48449=CARTESIAN_POINT('Ctrl Pts',(50.,2.06644706727002,14.2876778434072));
#48450=CARTESIAN_POINT('Ctrl Pts',(50.,1.90947068911084,14.2215285485816));
#48451=CARTESIAN_POINT('Ctrl Pts',(50.,1.85559389300112,14.1988250557891));
#48452=CARTESIAN_POINT('Ctrl Pts',(50.,1.80137373893839,14.1769071549062));
#48453=CARTESIAN_POINT('Ctrl Pts',(50.,1.74682506104155,14.1557864850509));
#48454=CARTESIAN_POINT('Ctrl Pts',(50.,1.69123832588192,14.134263890427));
#48455=CARTESIAN_POINT('Ctrl Pts',(50.,1.63531044223963,14.1135691537265));
#48456=CARTESIAN_POINT('Ctrl Pts',(50.,1.57906037163134,14.0937031294847));
#48457=CARTESIAN_POINT('Ctrl Pts',(47.1759584946969,-5.13650480025366,19.9998861825852));
#48458=CARTESIAN_POINT('Ctrl Pts',(47.1912290598737,-5.13673309193899,19.718218970967));
#48459=CARTESIAN_POINT('Ctrl Pts',(47.2064996250505,-5.11395904926684,19.4365882959574));
#48460=CARTESIAN_POINT('Ctrl Pts',(47.2217701902273,-5.06785627834494,19.1588297576462));
#48461=CARTESIAN_POINT('Ctrl Pts',(47.2680740203902,-4.92806218100213,18.3166026340693));
#48462=CARTESIAN_POINT('Ctrl Pts',(47.314377850553,-4.57377431728328,17.5099775019703));
#48463=CARTESIAN_POINT('Ctrl Pts',(47.3606816807159,-4.04815105701765,16.8372152064567));
#48464=CARTESIAN_POINT('Ctrl Pts',(47.4069855108788,-3.52252779675202,16.164452910943));
#48465=CARTESIAN_POINT('Ctrl Pts',(47.4532893410417,-2.82556913993962,15.6255534520147));
#48466=CARTESIAN_POINT('Ctrl Pts',(47.4995931712046,-2.04217666516686,15.2861640769393));
#48467=CARTESIAN_POINT('Ctrl Pts',(47.5458970013674,-1.2587841903941,14.9467747018639));
#48468=CARTESIAN_POINT('Ctrl Pts',(47.5922008315303,-0.388957897660963,
14.8068954106414));
#48469=CARTESIAN_POINT('Ctrl Pts',(47.6385046616932,0.461342373938519,14.8835659064419));
#48470=CARTESIAN_POINT('Ctrl Pts',(47.6848084918561,1.311642645538,14.9602364022424));
#48471=CARTESIAN_POINT('Ctrl Pts',(47.7311123220189,2.14241689600384,15.2534566850659));
#48472=CARTESIAN_POINT('Ctrl Pts',(47.7774161521818,2.85246250286255,15.7275074812189));
#48473=CARTESIAN_POINT('Ctrl Pts',(47.8237199823447,3.56250810972125,16.2015582773719));
#48474=CARTESIAN_POINT('Ctrl Pts',(47.8700238125076,4.15182507297281,16.8564395868543));
#48475=CARTESIAN_POINT('Ctrl Pts',(47.9163276426705,4.54862442109196,17.6123755536693));
#48476=CARTESIAN_POINT('Ctrl Pts',(47.9626314728334,4.9454237692111,18.3683115204842));
#48477=CARTESIAN_POINT('Ctrl Pts',(48.0089353029962,5.14970550219783,19.2253021446315));
#48478=CARTESIAN_POINT('Ctrl Pts',(48.0552391331591,5.13658459528959,20.0789512393964));
#48479=CARTESIAN_POINT('Ctrl Pts',(48.101542963322,5.12346368838135,20.9326003341614));
#48480=CARTESIAN_POINT('Ctrl Pts',(48.1478467934848,4.89294014157814,21.7829078995439));
#48481=CARTESIAN_POINT('Ctrl Pts',(48.1941506236477,4.47309567335396,22.526291726651));
#48482=CARTESIAN_POINT('Ctrl Pts',(48.2404544538106,4.05325120512978,23.2696755537581));
#48483=CARTESIAN_POINT('Ctrl Pts',(48.2867582839735,3.44408581548462,23.9061356425898));
#48484=CARTESIAN_POINT('Ctrl Pts',(48.3330621141364,2.71980639678025,24.3581403572819));
#48485=CARTESIAN_POINT('Ctrl Pts',(48.3793659442993,1.99552697807589,24.810145071974));
#48486=CARTESIAN_POINT('Ctrl Pts',(48.4256697744621,1.15613353031231,25.0776944125265));
#48487=CARTESIAN_POINT('Ctrl Pts',(48.471973604625,0.30387855446258,25.1281959122511));
#48488=CARTESIAN_POINT('Ctrl Pts',(48.5182774347879,-0.548376421387151,
25.1786974119757));
#48489=CARTESIAN_POINT('Ctrl Pts',(48.5645812649507,-1.41349292532303,25.0121510708724));
#48490=CARTESIAN_POINT('Ctrl Pts',(48.6108850951136,-2.18608467324978,24.648845783331));
#48491=CARTESIAN_POINT('Ctrl Pts',(48.6571889252765,-2.95867642117653,24.2855404957896));
#48492=CARTESIAN_POINT('Ctrl Pts',(48.7034927554394,-3.63874341309414,23.7254762618102));
#48493=CARTESIAN_POINT('Ctrl Pts',(48.7497965856023,-4.1434421202193,23.0368772228465));
#48494=CARTESIAN_POINT('Ctrl Pts',(48.7961004157652,-4.64814082734447,22.3482781838828));
#48495=CARTESIAN_POINT('Ctrl Pts',(48.842404245928,-4.97747124967718,21.531144339935));
#48496=CARTESIAN_POINT('Ctrl Pts',(48.8887080760909,-5.09131456590888,20.685019313948));
#48497=CARTESIAN_POINT('Ctrl Pts',(48.9011248822929,-5.12184271854912,20.4581229549778));
#48498=CARTESIAN_POINT('Ctrl Pts',(48.9135416884949,-5.13687531170795,20.2291418560254));
#48499=CARTESIAN_POINT('Ctrl Pts',(48.9259584946969,-5.13665113575917,20.0001315872378));
#48500=CARTESIAN_POINT('Ctrl Pts',(50.,-1.57888188187519,14.0941590297752));
#48501=CARTESIAN_POINT('Ctrl Pts',(49.9536961698371,-2.56072134667313,14.356646379112));
#48502=CARTESIAN_POINT('Ctrl Pts',(49.8610885095113,-4.38996617743935,15.3805039208954));
#48503=CARTESIAN_POINT('Ctrl Pts',(49.7221770190227,-6.06480273625955,18.0436167196139));
#48504=CARTESIAN_POINT('Ctrl Pts',(49.5832655285342,-6.26179330940861,21.1826217130423));
#48505=CARTESIAN_POINT('Ctrl Pts',(49.4443540380453,-4.93332128443375,24.0338649607667));
#48506=CARTESIAN_POINT('Ctrl Pts',(49.3054425475569,-2.40285814042326,25.9021352451997));
#48507=CARTESIAN_POINT('Ctrl Pts',(49.1665310570681,0.712991615200806,26.332535419579));
#48508=CARTESIAN_POINT('Ctrl Pts',(49.0276195665795,3.65514852614605,25.2200641339167));
#48509=CARTESIAN_POINT('Ctrl Pts',(48.8887080760909,5.70677685429529,22.8358293701168));
#48510=CARTESIAN_POINT('Ctrl Pts',(48.7497965856023,6.36804183630338,19.7606765440198));
#48511=CARTESIAN_POINT('Ctrl Pts',(48.6108850951136,5.47783010606213,16.7438373869472));
#48512=CARTESIAN_POINT('Ctrl Pts',(48.471973604625,3.25303119352331,14.5203085482529));
#48513=CARTESIAN_POINT('Ctrl Pts',(48.3330621141364,0.235681165538501,13.6318230833962));
#48514=CARTESIAN_POINT('Ctrl Pts',(48.1941506236477,-2.83908863701214,14.2948442639057));
#48515=CARTESIAN_POINT('Ctrl Pts',(48.0552391331592,-5.22215870445453,16.3478385001443));
#48516=CARTESIAN_POINT('Ctrl Pts',(47.9163276426704,-6.33293078716528,19.2906249877314));
#48517=CARTESIAN_POINT('Ctrl Pts',(47.7774161521818,-5.90078261843499,22.4062397932344));
#48518=CARTESIAN_POINT('Ctrl Pts',(47.6385046616932,-4.03100033593876,24.9356115677216));
#48519=CARTESIAN_POINT('Ctrl Pts',(47.4995931712046,-1.17912739907028,26.2624982202955));
#48520=CARTESIAN_POINT('Ctrl Pts',(47.3606816807159,1.96002163140553,26.0636243719931));
#48521=CARTESIAN_POINT('Ctrl Pts',(47.2217701902273,4.62164181175045,24.387442570214));
#48522=CARTESIAN_POINT('Ctrl Pts',(47.0828586997386,6.15727070156947,21.6423284830756));
#48523=CARTESIAN_POINT('Ctrl Pts',(46.94394720925,6.19277615550858,18.4970865545706));
#48524=CARTESIAN_POINT('Ctrl Pts',(46.8050357187613,4.71950782178093,15.7180061583685));
#48525=CARTESIAN_POINT('Ctrl Pts',(46.6661242282728,2.09640466180927,13.9821670984087));
#48526=CARTESIAN_POINT('Ctrl Pts',(46.527212737784,-1.03745495420322,13.7124796177954));
#48527=CARTESIAN_POINT('Ctrl Pts',(46.3883012472955,-3.91855477371191,14.9746488855395));
#48528=CARTESIAN_POINT('Ctrl Pts',(46.2493897568068,-5.84495954514333,17.4611669503603));
#48529=CARTESIAN_POINT('Ctrl Pts',(46.1104782663183,-6.34733064701209,20.5662322807994));
#48530=CARTESIAN_POINT('Ctrl Pts',(45.9715667758295,-5.30327315797554,23.5333439048828));
#48531=CARTESIAN_POINT('Ctrl Pts',(45.832655285341,-2.96715547971806,25.6396111299885));
#48532=CARTESIAN_POINT('Ctrl Pts',(45.6937437948522,0.0918635759318163,
26.371874639516));
#48533=CARTESIAN_POINT('Ctrl Pts',(45.5548323043637,3.12850149718234,25.5517297953366));
#48534=CARTESIAN_POINT('Ctrl Pts',(45.4159208138749,5.40292858824861,23.3789921587039));
#48535=CARTESIAN_POINT('Ctrl Pts',(45.2770093233864,6.36101599132474,20.3830155302438));
#48536=CARTESIAN_POINT('Ctrl Pts',(45.1380978328977,5.76934058177901,17.2937231128846));
#48537=CARTESIAN_POINT('Ctrl Pts',(44.9991863424091,3.77205488934985,14.8637730531032));
#48538=CARTESIAN_POINT('Ctrl Pts',(44.8602748519205,0.855766571765285,13.6851849660543));
#48539=CARTESIAN_POINT('Ctrl Pts',(44.7213633614318,-2.26901598809372,14.0451035454785));
#48540=CARTESIAN_POINT('Ctrl Pts',(44.5824518709432,-4.84098802139722,15.8558402160407));
#48541=CARTESIAN_POINT('Ctrl Pts',(44.4435403804545,-6.23352846356157,18.6762370936362));
#48542=CARTESIAN_POINT('Ctrl Pts',(44.3046288899659,-6.10736645042269,21.819148256341));
#48543=CARTESIAN_POINT('Ctrl Pts',(44.1657173994773,-4.49323939823524,24.5188521826282));
#48544=CARTESIAN_POINT('Ctrl Pts',(44.0268059089887,-1.78440430929869,26.1176079148025));
#48545=CARTESIAN_POINT('Ctrl Pts',(43.8878944185,1.35917319264309,26.2259034340967));
#48546=CARTESIAN_POINT('Ctrl Pts',(43.7489829280113,4.1716092428508,24.8173542181636));
#48547=CARTESIAN_POINT('Ctrl Pts',(43.6100714375227,5.967697451428,22.2351314204129));
#48548=CARTESIAN_POINT('Ctrl Pts',(43.4711599470341,6.309848804664,19.1083535450766));
#48549=CARTESIAN_POINT('Ctrl Pts',(43.3322484565454,5.11470343610716,16.1988114886301));
#48550=CARTESIAN_POINT('Ctrl Pts',(43.1933369660568,2.67343996414062,14.2153700121414));
#48551=CARTESIAN_POINT('Ctrl Pts',(43.0544254755682,-0.419165658805117,
13.6412638450101));
#48552=CARTESIAN_POINT('Ctrl Pts',(42.9155139850796,-3.40964807513886,14.6163650437647));
#48553=CARTESIAN_POINT('Ctrl Pts',(42.7766024945909,-5.56942266143649,16.9031053365388));
#48554=CARTESIAN_POINT('Ctrl Pts',(42.6376910041023,-6.37229386307993,19.9443559450525));
#48555=CARTESIAN_POINT('Ctrl Pts',(42.4987795136136,-5.62265457369981,22.999163363865));
#48556=CARTESIAN_POINT('Ctrl Pts',(42.3598680231251,-3.5031427704913,25.3232711811303));
#48557=CARTESIAN_POINT('Ctrl Pts',(42.2209565326363,-0.530144605918972,
26.350446601233));
#48558=CARTESIAN_POINT('Ctrl Pts',(42.0820450421478,2.57201506314977,25.8304342765551));
#48559=CARTESIAN_POINT('Ctrl Pts',(41.943133551659,5.04754318408075,23.8899271385383));
#48560=CARTESIAN_POINT('Ctrl Pts',(41.8042220611705,6.2933157545682,21.001699631427));
#48561=CARTESIAN_POINT('Ctrl Pts',(41.6653105706818,6.00581962429792,17.869423557181));
#48562=CARTESIAN_POINT('Ctrl Pts',(41.5263990801932,4.25509876298692,15.256229363099));
#48563=CARTESIAN_POINT('Ctrl Pts',(41.3874875897045,1.46768913436197,13.7987812534008));
#48564=CARTESIAN_POINT('Ctrl Pts',(41.248576099216,-1.67730017084697,13.8521638379692));
#48565=CARTESIAN_POINT('Ctrl Pts',(41.1096646087272,-4.41364132394809,15.4033712786614));
#48566=CARTESIAN_POINT('Ctrl Pts',(40.9707531182387,-6.07466727560423,18.0744759599007));
#48567=CARTESIAN_POINT('Ctrl Pts',(40.83184162775,-6.25569483461017,21.2147046861393));
#48568=CARTESIAN_POINT('Ctrl Pts',(40.6929301372614,-4.91261944606622,24.0589894698594));
#48569=CARTESIAN_POINT('Ctrl Pts',(40.5540186467727,-2.37266058160269,25.91436447159));
#48570=CARTESIAN_POINT('Ctrl Pts',(40.4151071562841,0.745360205886424,26.3287963706994));
#48571=CARTESIAN_POINT('Ctrl Pts',(40.2761956657955,3.68178554845507,25.2013152676496));
#48572=CARTESIAN_POINT('Ctrl Pts',(40.1372841753068,5.72120098964531,22.806614432796));
#48573=CARTESIAN_POINT('Ctrl Pts',(39.9983726848182,6.36673461236813,19.728125554767));
#48574=CARTESIAN_POINT('Ctrl Pts',(39.8594611943296,5.46111216921441,16.7158746653705));
#48575=CARTESIAN_POINT('Ctrl Pts',(39.7205497038409,3.22497451167542,14.5037499386089));
#48576=CARTESIAN_POINT('Ctrl Pts',(39.5816382133523,0.203121871393965,13.6307012282624));
#48577=CARTESIAN_POINT('Ctrl Pts',(39.4427267228636,-2.86821826005961,14.3094333014226));
#48578=CARTESIAN_POINT('Ctrl Pts',(39.303815232375,-5.24076153202002,16.3745836235273));
#48579=CARTESIAN_POINT('Ctrl Pts',(39.1649037418863,-6.33647460213517,19.3230103732012));
#48580=CARTESIAN_POINT('Ctrl Pts',(39.0259922513978,-5.88840398818078,22.4363751374273));
#48581=CARTESIAN_POINT('Ctrl Pts',(38.8870807609091,-4.00571514043749,24.9561549160581));
#48582=CARTESIAN_POINT('Ctrl Pts',(38.7481692704204,-1.14709597416125,26.2684444772495));
#48583=CARTESIAN_POINT('Ctrl Pts',(38.6092577799318,1.990995321361,26.0535248383579));
#48584=CARTESIAN_POINT('Ctrl Pts',(38.4703462894431,4.64401151042891,24.3637578334849));
#48585=CARTESIAN_POINT('Ctrl Pts',(38.3314347989546,6.16558637784845,21.6108289653426));
#48586=CARTESIAN_POINT('Ctrl Pts',(38.1925233084659,6.18501182457331,18.4654466225688));
#48587=CARTESIAN_POINT('Ctrl Pts',(38.0536118179773,4.69755514202461,15.6939343913573));
#48588=CARTESIAN_POINT('Ctrl Pts',(37.9147003274886,2.06561206307644,13.9715282083127));
#48589=CARTESIAN_POINT('Ctrl Pts',(37.775788837,-1.06958533326773,13.7178656052934));
#48590=CARTESIAN_POINT('Ctrl Pts',(37.6368773465114,-3.94419486492413,14.9947475382551));
#48591=CARTESIAN_POINT('Ctrl Pts',(37.4979658560227,-5.85786253827827,17.4910815435863));
#48592=CARTESIAN_POINT('Ctrl Pts',(37.3590543655341,-6.34435292805762,20.5986745881895));
#48593=CARTESIAN_POINT('Ctrl Pts',(37.2201428750454,-5.2851402019413,23.5604098618166));
#48594=CARTESIAN_POINT('Ctrl Pts',(37.0812313845568,-2.93828509988496,25.6547065361601));
#48595=CARTESIAN_POINT('Ctrl Pts',(36.9423198940682,0.124437559632812,26.371321733522));
#48596=CARTESIAN_POINT('Ctrl Pts',(36.8034084035795,3.15684293922622,25.5356632841381));
#48597=CARTESIAN_POINT('Ctrl Pts',(36.6644969130909,5.42013253618787,23.3513263983764));
#48598=CARTESIAN_POINT('Ctrl Pts',(36.5255854226022,6.36289097027834,20.3504908538714));
#48599=CARTESIAN_POINT('Ctrl Pts',(36.3866739321137,5.75542978222766,17.2642636530279));
#48600=CARTESIAN_POINT('Ctrl Pts',(36.247762441625,3.74574746168526,14.844556149896));
#48601=CARTESIAN_POINT('Ctrl Pts',(36.1088509511364,0.823471912402398,13.6808925196843));
#48602=CARTESIAN_POINT('Ctrl Pts',(35.9699394606477,-2.29942978666854,14.0567813438779));
#48603=CARTESIAN_POINT('Ctrl Pts',(35.8310279701591,-4.86211110923449,15.8806431448883));
#48604=CARTESIAN_POINT('Ctrl Pts',(35.6921164796705,-6.24021452817564,18.7081223043017));
#48605=CARTESIAN_POINT('Ctrl Pts',(35.5532049891818,-6.09798653594926,21.8503474121577));
#48606=CARTESIAN_POINT('Ctrl Pts',(35.4142934986932,-4.47007877524375,24.5417640935448));
#48607=CARTESIAN_POINT('Ctrl Pts',(35.2753820082045,-1.7531057040892,26.1266504493554));
#48608=CARTESIAN_POINT('Ctrl Pts',(35.1364705177159,1.39098436071829,26.2188735190977));
#48609=CARTESIAN_POINT('Ctrl Pts',(34.9975590272273,4.19618267645299,24.7959645832859));
#48610=CARTESIAN_POINT('Ctrl Pts',(34.8586475367386,5.97904621488101,22.2045933181914));
#48611=CARTESIAN_POINT('Ctrl Pts',(34.7197360462499,6.3052079479044,19.0761071101149));
#48612=CARTESIAN_POINT('Ctrl Pts',(34.5808245557615,5.09520363185058,16.1727130642877));
#48613=CARTESIAN_POINT('Ctrl Pts',(34.4419130652726,2.64383203702432,14.2017780744179));
#48614=CARTESIAN_POINT('Ctrl Pts',(34.3030015747841,-0.451668196904035,
13.6434898585621));
#48615=CARTESIAN_POINT('Ctrl Pts',(34.1640900842954,-3.43712648530661,14.6338666749417));
#48616=CARTESIAN_POINT('Ctrl Pts',(34.0251785938068,-5.58518225554684,16.9316185845593));
#48617=CARTESIAN_POINT('Ctrl Pts',(33.8862671033181,-6.37249506064328,19.9769339996099));
#48618=CARTESIAN_POINT('Ctrl Pts',(33.7473556128295,-5.60724835605281,23.0278690876325));
#48619=CARTESIAN_POINT('Ctrl Pts',(33.6084441223409,-3.47588262343321,25.341110870073));
#48620=CARTESIAN_POINT('Ctrl Pts',(33.4695326318522,-0.497672041157185,
26.3530738920422));
#48621=CARTESIAN_POINT('Ctrl Pts',(33.3306211413636,2.60178860923987,25.8172090706048));
#48622=CARTESIAN_POINT('Ctrl Pts',(33.191709650875,5.0673638491298,23.8640715519811));
#48623=CARTESIAN_POINT('Ctrl Pts',(33.0527981603864,6.29835454118703,20.9695129766052));
#48624=CARTESIAN_POINT('Ctrl Pts',(32.9138866698977,5.99484891033732,17.8387476129511));
#48625=CARTESIAN_POINT('Ctrl Pts',(32.774975179409,4.23079139261945,15.2345378471302));
#48626=CARTESIAN_POINT('Ctrl Pts',(32.6360636889205,1.43596722108643,13.7913589668703));
#48627=CARTESIAN_POINT('Ctrl Pts',(32.4971521984318,-1.70870807523846,13.8608191057836));
#48628=CARTESIAN_POINT('Ctrl Pts',(32.3582407079432,-4.43708317105403,15.4259953791621));
#48629=CARTESIAN_POINT('Ctrl Pts',(32.2193292174545,-6.08443182323413,18.1055568821649));
#48630=CARTESIAN_POINT('Ctrl Pts',(32.0804177269659,-6.24940310229619,21.2466700458854));
#48631=CARTESIAN_POINT('Ctrl Pts',(31.9415062364773,-4.8918043167284,24.0840514033414));
#48632=CARTESIAN_POINT('Ctrl Pts',(31.8025947459886,-2.34239333841841,25.9264170277183));
#48633=CARTESIAN_POINT('Ctrl Pts',(31.6636832554999,0.777705418913837,26.3249031312495));
#48634=CARTESIAN_POINT('Ctrl Pts',(31.5247717650114,3.70832832222358,25.1824247599837));
#48635=CARTESIAN_POINT('Ctrl Pts',(31.3858602745226,5.73547458931472,22.7773290358944));
#48636=CARTESIAN_POINT('Ctrl Pts',(31.2469487840341,6.36526149692924,19.6955802010263));
#48637=CARTESIAN_POINT('Ctrl Pts',(31.1080372935454,5.44425124037868,16.6879985250709));
#48638=CARTESIAN_POINT('Ctrl Pts',(30.9691258030568,3.19683367304369,14.48733460065));
#48639=CARTESIAN_POINT('Ctrl Pts',(30.8302143125682,0.170557201505726,13.629746034944));
#48640=CARTESIAN_POINT('Ctrl Pts',(30.6913028220795,-2.8972728848445,14.3241709707707));
#48641=CARTESIAN_POINT('Ctrl Pts',(30.5523913315909,-5.25922740334937,16.4014235511586));
#48642=CARTESIAN_POINT('Ctrl Pts',(30.4134798411023,-6.33985279708097,19.3554134273491));
#48643=CARTESIAN_POINT('Ctrl Pts',(30.2745683506136,-5.87587146197975,22.4664468168986));
#48644=CARTESIAN_POINT('Ctrl Pts',(30.135656860125,-3.98032524857262,24.9765687229126));
#48645=CARTESIAN_POINT('Ctrl Pts',(29.9967453696363,-1.11503456969162,26.2742269043038));
#48646=CARTESIAN_POINT('Ctrl Pts',(29.8578338791477,2.02191697488329,26.0432670870131));
#48647=CARTESIAN_POINT('Ctrl Pts',(29.7189223886591,4.6662598320792,24.3399590456387));
#48648=CARTESIAN_POINT('Ctrl Pts',(29.5800108981704,6.17374090938801,21.5792873462565));
#48649=CARTESIAN_POINT('Ctrl Pts',(29.4410994076818,6.17708584096459,18.4338467981542));
#48650=CARTESIAN_POINT('Ctrl Pts',(29.3021879171932,4.6754796861493,15.6699751683504));
#48651=CARTESIAN_POINT('Ctrl Pts',(29.1632764267045,2.03476547711032,13.9610468795116));
#48652=CARTESIAN_POINT('Ctrl Pts',(29.0243649362159,-1.10168775744487,13.7234157837727));
#48653=CARTESIAN_POINT('Ctrl Pts',(28.8854534457272,-3.96973186994514,15.0149770091765));
#48654=CARTESIAN_POINT('Ctrl Pts',(28.7465419552386,-5.87061242924704,17.5210617103551));
#48655=CARTESIAN_POINT('Ctrl Pts',(28.60763046475,-6.34120939193935,20.6311012485152));
#48656=CARTESIAN_POINT('Ctrl Pts',(28.4687189742614,-5.26686911251823,23.587382763227));
#48657=CARTESIAN_POINT('Ctrl Pts',(28.3298074837727,-2.90933792449704,25.6696541498914));
#48658=CARTESIAN_POINT('Ctrl Pts',(28.1908959932841,0.157008291011193,26.3706023055007));
#48659=CARTESIAN_POINT('Ctrl Pts',(28.0519845027954,3.18510187344724,25.5194520918348));
#48660=CARTESIAN_POINT('Ctrl Pts',(27.9130730123068,5.43719482255474,23.3235730471709));
#48661=CARTESIAN_POINT('Ctrl Pts',(27.7741615218181,6.36459964755315,20.3179570170062));
#48662=CARTESIAN_POINT('Ctrl Pts',(27.6352500313296,5.74136855771394,17.2348756948754));
#48663=CARTESIAN_POINT('Ctrl Pts',(27.4963385408409,3.71934213448194,14.8254739903094));
#48664=CARTESIAN_POINT('Ctrl Pts',(27.3574270503523,0.791155730627478,13.6767652306598));
#48665=CARTESIAN_POINT('Ctrl Pts',(27.2185155598636,-2.3297834869271,14.0686144753238));
#48666=CARTESIAN_POINT('Ctrl Pts',(27.079604069375,-4.88310712004916,15.905553737998));
#48667=CARTESIAN_POINT('Ctrl Pts',(26.9406925788864,-6.24673749740478,18.7400412797182));
#48668=CARTESIAN_POINT('Ctrl Pts',(26.8017810883977,-6.08844724338766,21.881498206957));
#48669=CARTESIAN_POINT('Ctrl Pts',(26.6628695979091,-4.44680132145817,24.5645573000867));
#48670=CARTESIAN_POINT('Ctrl Pts',(26.5239581074204,-1.7217612793893,26.135532856655));
#48671=CARTESIAN_POINT('Ctrl Pts',(26.3850466169318,1.42275917377253,26.2116810664862));
#48672=CARTESIAN_POINT('Ctrl Pts',(26.2461351264432,4.22064643785949,24.7744496002033));
#48673=CARTESIAN_POINT('Ctrl Pts',(26.1072236359545,5.99023870889178,22.1739975963169));
#48674=CARTESIAN_POINT('Ctrl Pts',(25.968312145466,6.30040229708003,19.0438848221863));
#48675=CARTESIAN_POINT('Ctrl Pts',(25.8294006549772,5.07557065842261,16.1467146706146));
#48676=CARTESIAN_POINT('Ctrl Pts',(25.6904891644886,2.61415501023178,14.18833768008));
#48677=CARTESIAN_POINT('Ctrl Pts',(25.551577674,-0.484158930120513,13.6458820070224));
#48678=CARTESIAN_POINT('Ctrl Pts',(25.4126661835113,-3.46451506210964,14.6515085563579));
#48679=CARTESIAN_POINT('Ctrl Pts',(25.2737546930227,-5.60079587431515,16.960212028356));
#48680=CARTESIAN_POINT('Ctrl Pts',(25.1348432025341,-6.37252970551363,20.0095126570244));
#48681=CARTESIAN_POINT('Ctrl Pts',(24.9959317120454,-5.59169558634022,23.0564956744613));
#48682=CARTESIAN_POINT('Ctrl Pts',(24.8570202215568,-3.44853163007304,25.358810962768));
#48683=CARTESIAN_POINT('Ctrl Pts',(24.7181087310682,-0.465186469148229,
26.3555351377534));
#48684=CARTESIAN_POINT('Ctrl Pts',(24.5791972405795,2.63149415450833,25.8038318250175));
#48685=CARTESIAN_POINT('Ctrl Pts',(24.4402857500909,5.08705207263311,23.8381149733452));
#48686=CARTESIAN_POINT('Ctrl Pts',(24.3013742596023,6.30322871286294,20.9373009824156));
#48687=CARTESIAN_POINT('Ctrl Pts',(24.1624627691136,5.98372151391236,17.8081281556077));
#48688=CARTESIAN_POINT('Ctrl Pts',(24.023551278625,4.20637344551665,15.2129708821494));
#48689=CARTESIAN_POINT('Ctrl Pts',(23.8846397881363,1.40420777710976,13.784098950514));
#48690=CARTESIAN_POINT('Ctrl Pts',(23.7457282976477,-1.74007132052403,13.8696348283494));
#48691=CARTESIAN_POINT('Ctrl Pts',(23.6068168071591,-4.46040904974499,15.4487390266817));
#48692=CARTESIAN_POINT('Ctrl Pts',(23.4679053166705,-6.09403734704428,18.1366873179397));
#48693=CARTESIAN_POINT('Ctrl Pts',(23.3289938261818,-6.24294803444307,21.2786028224357));
#48694=CARTESIAN_POINT('Ctrl Pts',(23.1900823356932,-4.87086133430093,24.109006595311));
#48695=CARTESIAN_POINT('Ctrl Pts',(23.0511708452045,-2.31206487401468,25.9383146899305));
#48696=CARTESIAN_POINT('Ctrl Pts',(22.9122593547159,0.810030305690605,26.3208445829778));
#48697=CARTESIAN_POINT('Ctrl Pts',(22.7733478642273,3.73477417444681,25.1633988035191));
#48698=CARTESIAN_POINT('Ctrl Pts',(22.6344363737386,5.74959828557432,22.7479710502147));
#48699=CARTESIAN_POINT('Ctrl Pts',(22.49552488325,6.36362201785506,19.6630428036569));
#48700=CARTESIAN_POINT('Ctrl Pts',(22.3566133927613,5.42724801959969,16.6602089478459));
#48701=CARTESIAN_POINT('Ctrl Pts',(22.2177019022727,3.16860928138414,14.4710633427192));
#48702=CARTESIAN_POINT('Ctrl Pts',(22.0787904117841,0.137988073903447,13.628957335745));
#48703=CARTESIAN_POINT('Ctrl Pts',(21.9398789212955,-2.9262517859769,14.3390569846214));
#48704=CARTESIAN_POINT('Ctrl Pts',(21.8009674308068,-5.27755581855221,16.4283575318402));
#48705=CARTESIAN_POINT('Ctrl Pts',(21.6620559403182,-6.34306529247789,19.3878333285293));
#48706=CARTESIAN_POINT('Ctrl Pts',(21.5231444498295,-5.86318536293062,22.496454032866));
#48707=CARTESIAN_POINT('Ctrl Pts',(21.3842329593409,-3.95483132620118,24.9968524612595));
#48708=CARTESIAN_POINT('Ctrl Pts',(21.2453214688522,-1.08294402247514,26.2798453470195));
#48709=CARTESIAN_POINT('Ctrl Pts',(21.1064099783636,2.05278578321474,26.0328513877377));
#48710=CARTESIAN_POINT('Ctrl Pts',(20.967498487875,4.68838619551153,24.3160468278314));
#48711=CARTESIAN_POINT('Ctrl Pts',(20.8285869973864,6.18173408290928,21.5477044506284));
#48712=CARTESIAN_POINT('Ctrl Pts',(20.6896755068977,6.16899841191383,18.4022879070052));
#48713=CARTESIAN_POINT('Ctrl Pts',(20.5507640164091,4.65328203108421,15.646129115662));
#48714=CARTESIAN_POINT('Ctrl Pts',(20.4118525259204,2.00386571014259,13.9507233858905));
#48715=CARTESIAN_POINT('Ctrl Pts',(20.2729410354318,-1.13376138770991,13.7291300082018));
#48716=CARTESIAN_POINT('Ctrl Pts',(20.1340295449432,-3.99516512133005,15.0353367695678));
#48717=CARTESIAN_POINT('Ctrl Pts',(19.9951180544545,-5.88320888481873,17.5511066671072));
#48718=CARTESIAN_POINT('Ctrl Pts',(19.8562065639659,-6.33790012081599,20.6635114142635));
#48719=CARTESIAN_POINT('Ctrl Pts',(19.7172950734772,-5.24846036724355,23.6142619041474));
#48720=CARTESIAN_POINT('Ctrl Pts',(19.5783835829886,-2.8803147101225,25.6844535805079));
#48721=CARTESIAN_POINT('Ctrl Pts',(19.4394720925,0.189574918792307,26.3697163742558));
#48722=CARTESIAN_POINT('Ctrl Pts',(19.3005606020113,3.21327756126488,25.5030966421251));
#48723=CARTESIAN_POINT('Ctrl Pts',(19.1616491115227,5.45411500140619,23.2957328304541));
#48724=CARTESIAN_POINT('Ctrl Pts',(19.0227376210341,6.36614197849088,20.2854148699583));
#48725=CARTESIAN_POINT('Ctrl Pts',(18.8838261305454,5.72715727574455,17.2055600065159));
#48726=CARTESIAN_POINT('Ctrl Pts',(18.7449146400568,3.69283959787427,14.8065270730783));
#48727=CARTESIAN_POINT('Ctrl Pts',(18.6060031495682,0.758818871062057,13.6728032068524));
#48728=CARTESIAN_POINT('Ctrl Pts',(18.4670916590795,-2.36007629553962,14.0806026305434));
#48729=CARTESIAN_POINT('Ctrl Pts',(18.3281801685909,-4.90397550508568,15.9305713443019));
#48730=CARTESIAN_POINT('Ctrl Pts',(18.1892686781022,-6.2530972007635,18.7719931856456));
#48731=CARTESIAN_POINT('Ctrl Pts',(18.0503571876136,-6.07874882205854,21.9125998265761));
#48732=CARTESIAN_POINT('Ctrl Pts',(17.911445697125,-4.42340764526233,24.5872312065266));
#48733=CARTESIAN_POINT('Ctrl Pts',(17.7725342066364,-1.6903718544226,26.1442549045489));
#48734=CARTESIAN_POINT('Ctrl Pts',(17.6336227161477,1.45449680133364,26.2043262642456));
#48735=CARTESIAN_POINT('Ctrl Pts',(17.4947112256591,4.24499988768104,24.7528098312351));
#48736=CARTESIAN_POINT('Ctrl Pts',(17.3557997351704,6.00127464093126,22.1433450544447));
#48737=CARTESIAN_POINT('Ctrl Pts',(17.2168882446818,6.29543197779222,19.0116875234582));
#48738=CARTESIAN_POINT('Ctrl Pts',(17.0779767541932,5.05580502895429,16.1208169871096));
#48739=CARTESIAN_POINT('Ctrl Pts',(16.9390652637045,2.5844096594071,14.1750491804084));
#48740=CARTESIAN_POINT('Ctrl Pts',(16.8001537732159,-0.516637009270994,
13.6484402278693));
#48741=CARTESIAN_POINT('Ctrl Pts',(16.6612422827273,-3.49181308971526,14.6692902269219));
#48742=CARTESIAN_POINT('Ctrl Pts',(16.5223307922386,-5.61626310966114,16.9888849206056));
#48743=CARTESIAN_POINT('Ctrl Pts',(16.38341930175,-6.37239779678543,20.0420910658145));
#48744=CARTESIAN_POINT('Ctrl Pts',(16.2445078112613,-5.57599667105201,23.0850423761618));
#48745=CARTESIAN_POINT('Ctrl Pts',(16.1055963207727,-3.42109050526117,25.3763709966026));
#48746=CARTESIAN_POINT('Ctrl Pts',(15.9666848302841,-0.432688738940727,
26.3578302740393));
#48747=CARTESIAN_POINT('Ctrl Pts',(15.8277733397954,2.66113092256575,25.7903028894231));
#48748=CARTESIAN_POINT('Ctrl Pts',(15.6888618493068,5.10660734001576,23.8120580810363));
#48749=CARTESIAN_POINT('Ctrl Pts',(15.5499503588182,6.30793814220377,20.9050644907565));
#48750=CARTESIAN_POINT('Ctrl Pts',(15.4110388683295,5.97243772585063,17.7775659854265));
#48751=CARTESIAN_POINT('Ctrl Pts',(15.2721273778409,4.1818455598703,15.1915290318346));
#48752=CARTESIAN_POINT('Ctrl Pts',(15.1332158873523,1.37241163250246,13.777001394081));
#48753=CARTESIAN_POINT('Ctrl Pts',(14.9943043968636,-1.77138908698832,13.8786107752573));
#48754=CARTESIAN_POINT('Ctrl Pts',(14.855392906375,-4.48361835037166,15.4716016267882));
#48755=CARTESIAN_POINT('Ctrl Pts',(14.7164814158863,-6.10348359598301,18.1678664535947));
#48756=CARTESIAN_POINT('Ctrl Pts',(14.5775699253977,-6.2363297997616,21.3105021811896));
#48757=CARTESIAN_POINT('Ctrl Pts',(14.4386584349091,-4.84979104615329,24.133854393535));
#48758=CARTESIAN_POINT('Ctrl Pts',(14.2997469444204,-2.28167598106183,25.950057147267));
#48759=CARTESIAN_POINT('Ctrl Pts',(14.1608354539318,0.842334021367499,26.3166208319594));
#48760=CARTESIAN_POINT('Ctrl Pts',(14.0219239634432,3.7611224139311,25.1442378955218));
#48761=CARTESIAN_POINT('Ctrl Pts',(13.8830124729545,5.76357170928461,22.7185412430624));
#48762=CARTESIAN_POINT('Ctrl Pts',(13.7441009824659,6.36181621799531,19.6305142130623));
#48763=CARTESIAN_POINT('Ctrl Pts',(13.6051894919773,5.41010295127669,16.6325066600089));
#48764=CARTESIAN_POINT('Ctrl Pts',(13.4662780014886,3.14030207437455,14.4549365900852));
#48765=CARTESIAN_POINT('Ctrl Pts',(13.327366511,0.105415339819669,13.6283351512789));
#48766=CARTESIAN_POINT('Ctrl Pts',(13.1884550205113,-2.95515420605895,14.354090953911));
#48767=CARTESIAN_POINT('Ctrl Pts',(13.0495435300227,-5.29574629859371,16.4553848616206));
#48768=CARTESIAN_POINT('Ctrl Pts',(12.9106320395341,-6.34611200436357,19.4202692294091));
#48769=CARTESIAN_POINT('Ctrl Pts',(12.7717205490454,-5.8503460225996,22.5263960010557));
#48770=CARTESIAN_POINT('Ctrl Pts',(12.6328090585568,-3.92923403963699,25.0170056009591));
#48771=CARTESIAN_POINT('Ctrl Pts',(12.4938975680681,-1.05082517123617,26.285299658552));
#48772=CARTESIAN_POINT('Ctrl Pts',(12.3549860775795,2.0836009395627,26.0222780127582));
#48773=CARTESIAN_POINT('Ctrl Pts',(12.2160745870909,4.71039002242726,24.2920218050372));
#48774=CARTESIAN_POINT('Ctrl Pts',(12.0771630966022,6.1895656895012,21.5160811039145));
#48775=CARTESIAN_POINT('Ctrl Pts',(11.9382516061136,6.1607497487956,18.370770773951));
#48776=CARTESIAN_POINT('Ctrl Pts',(11.799340115625,4.63096275699136,15.6223968565371));
#48777=CARTESIAN_POINT('Ctrl Pts',(11.6604286251363,1.97291356977519,13.9405579972662));
#48778=CARTESIAN_POINT('Ctrl Pts',(11.5215171346477,-1.1658053857806,13.7350081292326));
#48779=CARTESIAN_POINT('Ctrl Pts',(11.3826056441591,-4.02049395435078,15.0558262873028));
#48780=CARTESIAN_POINT('Ctrl Pts',(11.2436941536704,-5.89565157577014,17.5812156285819));
#48781=CARTESIAN_POINT('Ctrl Pts',(11.1047826631818,-6.33442520117924,20.6959042383565));
#48782=CARTESIAN_POINT('Ctrl Pts',(10.9658711726931,-5.22991444725156,23.6410465820594));
#48783=CARTESIAN_POINT('Ctrl Pts',(10.8269596822045,-2.85121621531744,25.699104441209));
#48784=CARTESIAN_POINT('Ctrl Pts',(10.6880481917159,0.222136591808738,26.3686639629421));
#48785=CARTESIAN_POINT('Ctrl Pts',(10.5491367012273,3.24136926627416,25.486597362478));
#48786=CARTESIAN_POINT('Ctrl Pts',(10.4102252107386,5.47089263051329,23.267806475863));
#48787=CARTESIAN_POINT('Ctrl Pts',(10.27131372025,6.36751792278091,20.2528652632554));
#48788=CARTESIAN_POINT('Ctrl Pts',(10.1324022297613,5.71279630774815,17.1763173541497));
#48789=CARTESIAN_POINT('Ctrl Pts',(9.99349073927272,3.66624054453745,14.7877158934027));
#48790=CARTESIAN_POINT('Ctrl Pts',(9.85457924878407,0.726462178868265,13.6690065518142));
#48791=CARTESIAN_POINT('Ctrl Pts',(9.71566775829543,-2.39030742076759,14.0927454962123));
#48792=CARTESIAN_POINT('Ctrl Pts',(9.5767562678068,-4.92471571892393,15.9556953099351));
#48793=CARTESIAN_POINT('Ctrl Pts',(9.43784477731815,-6.25929347203341,18.803977186983));
#48794=CARTESIAN_POINT('Ctrl Pts',(9.29893328682952,-6.06889152544171,21.9436514581372));
#48795=CARTESIAN_POINT('Ctrl Pts',(9.16002179634088,-4.39989835807759,24.6097852202552));
#48796=CARTESIAN_POINT('Ctrl Pts',(9.02111030585225,-1.65893824958895,26.152816365076));
#48797=CARTESIAN_POINT('Ctrl Pts',(8.88219881536361,1.48619641390095,26.1968093046023));
#48798=CARTESIAN_POINT('Ctrl Pts',(8.74328732487498,4.26924238941132,24.7310458419625));
#48799=CARTESIAN_POINT('Ctrl Pts',(8.60437583438633,6.01215372256228,22.1126364937154));
#48800=CARTESIAN_POINT('Ctrl Pts',(8.4654643438977,6.29029711994617,18.9795160554453));
#48801=CARTESIAN_POINT('Ctrl Pts',(8.32655285340906,5.03590726004376,16.0950206906393));
#48802=CARTESIAN_POINT('Ctrl Pts',(8.18764136292043,2.55459676198038,14.1619129227137));
#48803=CARTESIAN_POINT('Ctrl Pts',(8.04872987243179,-0.549101585502231,
13.6511644542408));
#48804=CARTESIAN_POINT('Ctrl Pts',(7.90981838194317,-3.51901985465715,14.6872112218886));
#48805=CARTESIAN_POINT('Ctrl Pts',(7.77090689145451,-5.63158355733028,17.017636511908));
#48806=CARTESIAN_POINT('Ctrl Pts',(7.63199540096589,-6.37209933790631,20.0746683745047));
#48807=CARTESIAN_POINT('Ctrl Pts',(7.49308391047725,-5.56015202049796,23.1135084466321));
#48808=CARTESIAN_POINT('Ctrl Pts',(7.35417241998862,-3.39355996620412,25.3937905126241));
#48809=CARTESIAN_POINT('Ctrl Pts',(7.21526092949997,-0.400179699901651,
26.3599592409137));
#48810=CARTESIAN_POINT('Ctrl Pts',(7.07634943901134,2.69069813882,25.7766226174165));
#48811=CARTESIAN_POINT('Ctrl Pts',(6.93743794852271,5.12602914017768,23.7859015560823));
#48812=CARTESIAN_POINT('Ctrl Pts',(6.79852645803408,6.31248270612288,20.8728043441669));
#48813=CARTESIAN_POINT('Ctrl Pts',(6.65961496754543,5.96099784106742,17.7470619011862));
#48814=CARTESIAN_POINT('Ctrl Pts',(6.5207034770568,4.15720837674583,15.1702128565938));
#48815=CARTESIAN_POINT('Ctrl Pts',(6.38179198656816,1.34057961829449,13.7700664830746));
#48816=CARTESIAN_POINT('Ctrl Pts',(6.24288049607952,-1.80266055610438,13.8877467119104));
#48817=CARTESIAN_POINT('Ctrl Pts',(6.10396900559088,-4.50671046633138,15.4945825819403));
#48818=CARTESIAN_POINT('Ctrl Pts',(5.96505751510225,-6.11277032316134,18.1990934742261));
#48819=CARTESIAN_POINT('Ctrl Pts',(5.82614602461361,-6.22954857122723,21.3423672884193));
#48820=CARTESIAN_POINT('Ctrl Pts',(5.68723453412497,-4.82859400298248,24.1585941485866));
#48821=CARTESIAN_POINT('Ctrl Pts',(5.54832304363634,-2.25122745380935,25.9616440928248));
#48822=CARTESIAN_POINT('Ctrl Pts',(5.4094115531477,0.874615721648888,26.3122319885871));
#48823=CARTESIAN_POINT('Ctrl Pts',(5.27050006265906,3.78737235203403,25.1249425367847));
#48824=CARTESIAN_POINT('Ctrl Pts',(5.13158857217043,5.77739449523354,22.6890403836206));
#48825=CARTESIAN_POINT('Ctrl Pts',(4.99267708168179,6.35984414454672,19.5979952794158));
#48826=CARTESIAN_POINT('Ctrl Pts',(4.85376559119316,5.39281648351639,16.604892385592));
#48827=CARTESIAN_POINT('Ctrl Pts',(4.71485410070452,3.11191279185723,14.4389547642397));
#48828=CARTESIAN_POINT('Ctrl Pts',(4.57594261021589,0.0728398505813112,
13.6278794978073));
#48829=CARTESIAN_POINT('Ctrl Pts',(4.43703111972725,-2.98397938969178,14.3692724857092));
#48830=CARTESIAN_POINT('Ctrl Pts',(4.29811962923861,-5.31379836804421,16.4825048341088));
#48831=CARTESIAN_POINT('Ctrl Pts',(4.15920813874997,-6.34899285310857,19.4527202822382));
#48832=CARTESIAN_POINT('Ctrl Pts',(4.02029664826134,-5.83735377655805,22.5562719388986));
#48833=CARTESIAN_POINT('Ctrl Pts',(3.8813851577727,-3.90353405789533,25.0370276152856));
#48834=CARTESIAN_POINT('Ctrl Pts',(3.74247366728407,-1.01867885543911,26.2905896963458));
#48835=CARTESIAN_POINT('Ctrl Pts',(3.60356217679543,2.11436163853657,26.0115472384233));
#48836=CARTESIAN_POINT('Ctrl Pts',(3.46465068630679,4.73227073773,24.2678846051763));
#48837=CARTESIAN_POINT('Ctrl Pts',(3.32573919581815,6.19723552447633,21.4844181326321));
#48838=CARTESIAN_POINT('Ctrl Pts',(3.18682770532951,6.15234006719685,18.3392962227209));
#48839=CARTESIAN_POINT('Ctrl Pts',(3.04791621484088,4.60852244721424,15.5987790112615));
#48840=CARTESIAN_POINT('Ctrl Pts',(2.90900472435224,1.94190986497335,13.9305509792932));
#48841=CARTESIAN_POINT('Ctrl Pts',(2.77009323386361,-1.19781891413772,13.7410499932924));
#48842=CARTESIAN_POINT('Ctrl Pts',(2.63118174337496,-4.04571770703044,15.0764450267472));
#48843=CARTESIAN_POINT('Ctrl Pts',(2.49227025288634,-5.90794017685321,17.6113878080752));
#48844=CARTESIAN_POINT('Ctrl Pts',(2.3533587623977,-6.33078472393609,20.7282788737186));
#48845=CARTESIAN_POINT('Ctrl Pts',(2.21444727190907,-5.2112318370928,23.6677360978016));
#48846=CARTESIAN_POINT('Ctrl Pts',(2.07553578142043,-2.82204320093811,25.7136063473297));
#48847=CARTESIAN_POINT('Ctrl Pts',(1.93662429093179,0.254692459677778,26.3674451025059));
#48848=CARTESIAN_POINT('Ctrl Pts',(1.79771280044316,3.26937625297555,25.4699546773483));
#48849=CARTESIAN_POINT('Ctrl Pts',(1.65880130995452,5.48752727391192,23.2397947266211));
#48850=CARTESIAN_POINT('Ctrl Pts',(1.51988981946589,6.36872743946243,20.220309021366));
#48851=CARTESIAN_POINT('Ctrl Pts',(1.38097832897725,5.69828603890732,17.1471485537567));
#48852=CARTESIAN_POINT('Ctrl Pts',(1.24206683848861,3.63954565029315,14.7690408411714));
#48853=CARTESIAN_POINT('Ctrl Pts',(1.10315534799997,0.694086537873731,13.6653755651264));
#48854=CARTESIAN_POINT('Ctrl Pts',(0.964243857511333,-2.4204761475888,14.1050423605135));
#48855=CARTESIAN_POINT('Ctrl Pts',(0.8253323670227,-4.94532707163062,15.9809257548385));
#48856=CARTESIAN_POINT('Ctrl Pts',(0.686420876534066,-6.26532644037927,
18.8359909188598));
#48857=CARTESIAN_POINT('Ctrl Pts',(0.547509386045428,-6.05887503803249,
21.9746553002093));
#48858=CARTESIAN_POINT('Ctrl Pts',(0.408597895556788,-4.37627520273034,
24.6322128254603));
#48859=CARTESIAN_POINT('Ctrl Pts',(0.269686405068149,-1.62745906490466,
26.1612286823026));
#48860=CARTESIAN_POINT('Ctrl Pts',(0.13077491457951,1.51785280933213,26.1891074109947));
#48861=CARTESIAN_POINT('Ctrl Pts',(-0.00813657590912298,4.29338191907513,
24.7092034479418));
#48862=CARTESIAN_POINT('Ctrl Pts',(-0.147048066397757,6.02285873175444,
22.0817834333193));
#48863=CARTESIAN_POINT('Ctrl Pts',(-0.285959556886395,6.28503105744338,
18.9475493472432));
#48864=CARTESIAN_POINT('Ctrl Pts',(-0.42487104737502,5.01581409828515,16.0689497592415));
#48865=CARTESIAN_POINT('Ctrl Pts',(-0.51747870770078,3.35514622044529,14.789651859508));
#48866=CARTESIAN_POINT('Ctrl Pts',(-0.563782537863657,2.4219910006092,14.3869985608885));
#48867=CARTESIAN_POINT('Ctrl Pts',(50.1879275126212,-1.49481431510623,14.4086155358576));
#48868=CARTESIAN_POINT('Ctrl Pts',(50.1416236824583,-2.42437573699871,14.657126746118));
#48869=CARTESIAN_POINT('Ctrl Pts',(50.0490160221326,-4.15622242562869,15.626468992461));
#48870=CARTESIAN_POINT('Ctrl Pts',(49.9101045316439,-5.74188231084713,18.1477843485781));
#48871=CARTESIAN_POINT('Ctrl Pts',(49.7711930411553,-5.92838412080803,21.119653019206));
#48872=CARTESIAN_POINT('Ctrl Pts',(49.6322815506666,-4.67064658961787,23.8190818184562));
#48873=CARTESIAN_POINT('Ctrl Pts',(49.4933700601781,-2.27491795726246,25.5878760504486));
#48874=CARTESIAN_POINT('Ctrl Pts',(49.3544585696894,0.675028376212077,25.9953595672789));
#48875=CARTESIAN_POINT('Ctrl Pts',(49.2155470792007,3.46053014062925,24.9421218159042));
#48876=CARTESIAN_POINT('Ctrl Pts',(49.0766355887121,5.40291951718768,22.6848356335654));
#48877=CARTESIAN_POINT('Ctrl Pts',(48.9377240982235,6.02897544482311,19.7734193215803));
#48878=CARTESIAN_POINT('Ctrl Pts',(48.7988126077348,5.18616303870463,16.9172117672766));
#48879=CARTESIAN_POINT('Ctrl Pts',(48.6599011172463,3.07982354562869,14.8120747229625));
#48880=CARTESIAN_POINT('Ctrl Pts',(48.5209896267576,0.223132321734829,13.9708966672272));
#48881=CARTESIAN_POINT('Ctrl Pts',(48.3820781362689,-2.68792136079287,14.5986152845737));
#48882=CARTESIAN_POINT('Ctrl Pts',(48.2431666457803,-4.94410486103247,16.5422978414445));
#48883=CARTESIAN_POINT('Ctrl Pts',(48.1042551552916,-5.99573388351791,19.3283956606948));
#48884=CARTESIAN_POINT('Ctrl Pts',(47.965343664803,-5.58659544429675,22.2781195539676));
#48885=CARTESIAN_POINT('Ctrl Pts',(47.8264321743144,-3.81636972057899,24.6728149267706));
#48886=CARTESIAN_POINT('Ctrl Pts',(47.6875206838257,-1.11634475998348,25.9290514987144));
#48887=CARTESIAN_POINT('Ctrl Pts',(47.5486091933372,1.85566027843902,25.7407666885868));
#48888=CARTESIAN_POINT('Ctrl Pts',(47.4096977028485,4.37556249064878,24.1538331878717));
#48889=CARTESIAN_POINT('Ctrl Pts',(47.2707862123599,5.8294268192874,21.5548827019868));
#48890=CARTESIAN_POINT('Ctrl Pts',(47.1318747218713,5.86304178530974,18.5771091818944));
#48891=CARTESIAN_POINT('Ctrl Pts',(46.9929632313825,4.46821762491516,15.9460009230928));
#48892=CARTESIAN_POINT('Ctrl Pts',(46.854051740894,1.98478159430525,14.3025866149454));
#48893=CARTESIAN_POINT('Ctrl Pts',(46.7151402504053,-0.982215664530275,
14.0472586444028));
#48894=CARTESIAN_POINT('Ctrl Pts',(46.5762287599167,-3.70991132238189,15.2422237087116));
#48895=CARTESIAN_POINT('Ctrl Pts',(46.437317269428,-5.53374467057676,17.5963471176458));
#48896=CARTESIAN_POINT('Ctrl Pts',(46.2984057789394,-6.00936702281833,20.5360832426609));
#48897=CARTESIAN_POINT('Ctrl Pts',(46.1594942884507,-5.02090037542599,23.3452110064999));
#48898=CARTESIAN_POINT('Ctrl Pts',(46.0205827979622,-2.80916928438035,25.3393300319128));
#48899=CARTESIAN_POINT('Ctrl Pts',(45.8816713074734,0.0869722997749769,
26.0326041704263));
#48900=CARTESIAN_POINT('Ctrl Pts',(45.7427598169849,2.96192443304577,25.2561279389783));
#48901=CARTESIAN_POINT('Ctrl Pts',(45.6038483264962,5.11524965225304,23.1990777191409));
#48902=CARTESIAN_POINT('Ctrl Pts',(45.4649368360076,6.02232369096466,20.362621868101));
#48903=CARTESIAN_POINT('Ctrl Pts',(45.3260253455189,5.46215203896315,17.4378188273991));
#48904=CARTESIAN_POINT('Ctrl Pts',(45.1871138550303,3.57121182445256,15.1372514600414));
#48905=CARTESIAN_POINT('Ctrl Pts',(45.0482023645417,0.810201280126699,14.0214172964104));
#48906=CARTESIAN_POINT('Ctrl Pts',(44.909290874053,-2.14820223041581,14.3621720108524));
#48907=CARTESIAN_POINT('Ctrl Pts',(44.7703793835644,-4.58322961122835,16.0764960062797));
#48908=CARTESIAN_POINT('Ctrl Pts',(44.6314678930757,-5.90162423669546,18.7467208503976));
#48909=CARTESIAN_POINT('Ctrl Pts',(44.4925564025871,-5.78217972002354,21.7222877063162));
#48910=CARTESIAN_POINT('Ctrl Pts',(44.3536449120985,-4.25399686371996,24.2782458953922));
#48911=CARTESIAN_POINT('Ctrl Pts',(44.2147334216098,-1.68939370075548,25.7918758776261));
#48912=CARTESIAN_POINT('Ctrl Pts',(44.0758219311212,1.28680401516706,25.8944052019291));
#48913=CARTESIAN_POINT('Ctrl Pts',(43.9369104406326,3.94949190615626,24.5608541898624));
#48914=CARTESIAN_POINT('Ctrl Pts',(43.7979989501439,5.649947396966,22.1161218465619));
#48915=CARTESIAN_POINT('Ctrl Pts',(43.6590874596554,5.97388090118906,19.1558292611159));
#48916=CARTESIAN_POINT('Ctrl Pts',(43.5201759691666,4.84237104851417,16.4012057732497));
#48917=CARTESIAN_POINT('Ctrl Pts',(43.3812644786781,2.53109265161001,14.5233726393934));
#48918=CARTESIAN_POINT('Ctrl Pts',(43.2423529881893,-0.396847183044917,
13.9798347554831));
#48919=CARTESIAN_POINT('Ctrl Pts',(43.1034414977008,-3.22810136128653,14.9030166903119));
#48920=CARTESIAN_POINT('Ctrl Pts',(42.9645300072121,-5.27287874841191,17.0679994947944));
#48921=CARTESIAN_POINT('Ctrl Pts',(42.8256185167235,-6.03300107243133,19.9473187127923));
#48922=CARTESIAN_POINT('Ctrl Pts',(42.6867070262348,-5.32327632747411,22.8394729087162));
#48923=CARTESIAN_POINT('Ctrl Pts',(42.5477955357463,-3.31661793152758,25.0398336038256));
#48924=CARTESIAN_POINT('Ctrl Pts',(42.4088840452575,-0.501917056051616,
26.0123170680549));
#48925=CARTESIAN_POINT('Ctrl Pts',(42.269972554769,2.43506811953463,25.5199927999233));
#48926=CARTESIAN_POINT('Ctrl Pts',(42.1310610642802,4.7787867441481,23.6828079656607));
#48927=CARTESIAN_POINT('Ctrl Pts',(41.9921495737917,5.95822815335576,20.9483641339372));
#48928=CARTESIAN_POINT('Ctrl Pts',(41.853238083303,5.68603975471807,17.9828661011859));
#48929=CARTESIAN_POINT('Ctrl Pts',(41.7143265928144,4.02853602674152,15.5088114335707));
#48930=CARTESIAN_POINT('Ctrl Pts',(41.5754151023257,1.38954202550255,14.1289651493675));
#48931=CARTESIAN_POINT('Ctrl Pts',(41.4365036118372,-1.58799232222133,14.1795053781877));
#48932=CARTESIAN_POINT('Ctrl Pts',(41.2975921213485,-4.17863698894705,15.6481187777488));
#48933=CARTESIAN_POINT('Ctrl Pts',(41.1586806308599,-5.75122161278835,18.177000488597));
#48934=CARTESIAN_POINT('Ctrl Pts',(41.0197691403712,-5.92261035930397,21.1500277343807));
#48935=CARTESIAN_POINT('Ctrl Pts',(40.8808576498826,-4.65104702064691,23.8428685730469));
#48936=CARTESIAN_POINT('Ctrl Pts',(40.7419461593939,-2.24632826747982,25.5994541316722));
#48937=CARTESIAN_POINT('Ctrl Pts',(40.6030346689053,0.705673501266786,25.9918196040593));
#48938=CARTESIAN_POINT('Ctrl Pts',(40.4641231784166,3.48574887466908,24.924371233033));
#48939=CARTESIAN_POINT('Ctrl Pts',(40.3252116879281,5.41657563944215,22.6571762456001));
#48940=CARTESIAN_POINT('Ctrl Pts',(40.1863001974394,6.02773782402709,19.7426015097702));
#48941=CARTESIAN_POINT('Ctrl Pts',(40.0473887069508,5.17033524841463,16.8907379208274));
#48942=CARTESIAN_POINT('Ctrl Pts',(39.9084772164621,3.05326074182299,14.7963977764992));
#48943=CARTESIAN_POINT('Ctrl Pts',(39.7695657259735,0.192306647226999,13.9698345452706));
#48944=CARTESIAN_POINT('Ctrl Pts',(39.6306542354848,-2.71549997704331,14.6124275287791));
#48945=CARTESIAN_POINT('Ctrl Pts',(39.4917427449962,-4.96171718103282,16.5676189207165));
#48946=CARTESIAN_POINT('Ctrl Pts',(39.3528312545075,-5.99908900805755,19.3590566862954));
#48947=CARTESIAN_POINT('Ctrl Pts',(39.213919764019,-5.57487591421802,22.3066503417405));
#48948=CARTESIAN_POINT('Ctrl Pts',(39.0750082735303,-3.7924308353277,24.6922644445124));
#48949=CARTESIAN_POINT('Ctrl Pts',(38.9360967830417,-1.08601884831338,25.9346811472132));
#48950=CARTESIAN_POINT('Ctrl Pts',(38.797185292553,1.88498477425381,25.7312049046261));
#48951=CARTESIAN_POINT('Ctrl Pts',(38.6582738020644,4.39674111470739,24.1314095449642));
#48952=CARTESIAN_POINT('Ctrl Pts',(38.5193623115757,5.8372997273778,21.5250603760948));
#48953=CARTESIAN_POINT('Ctrl Pts',(38.3804508210871,5.85569086617989,18.5471539180915));
#48954=CARTESIAN_POINT('Ctrl Pts',(38.2415393305985,4.44743381560593,15.9232108573309));
#48955=CARTESIAN_POINT('Ctrl Pts',(38.1026278401099,1.95562854751085,14.292514192559));
#48956=CARTESIAN_POINT('Ctrl Pts',(37.9637163496212,-1.01263526154179,14.0523578549931));
#48957=CARTESIAN_POINT('Ctrl Pts',(37.8248048591326,-3.73418620692178,15.2612522086511));
#48958=CARTESIAN_POINT('Ctrl Pts',(37.6858933686439,-5.54596064383431,17.6246689083371));
#48959=CARTESIAN_POINT('Ctrl Pts',(37.5469818781554,-6.00654785251142,20.5667981593741));
#48960=CARTESIAN_POINT('Ctrl Pts',(37.4080703876666,-5.00373290864692,23.3708358365401));
#48961=CARTESIAN_POINT('Ctrl Pts',(37.2691588971781,-2.78183610793918,25.3536216831735));
#48962=CARTESIAN_POINT('Ctrl Pts',(37.1302474066894,0.11781188169383,26.0320807039123));
#48963=CARTESIAN_POINT('Ctrl Pts',(36.9913359162008,2.98875683499064,25.2409168891785));
#48964=CARTESIAN_POINT('Ctrl Pts',(36.8524244257121,5.13153757597372,23.1728850222391));
#48965=CARTESIAN_POINT('Ctrl Pts',(36.7135129352235,6.02409883666274,20.331828968142));
#48966=CARTESIAN_POINT('Ctrl Pts',(36.5746014447349,5.44898191994243,17.4099279365006));
#48967=CARTESIAN_POINT('Ctrl Pts',(36.4356899542462,3.54630513579011,15.1190577608572));
#48968=CARTESIAN_POINT('Ctrl Pts',(36.2967784637576,0.779626149921396,14.01735340135));
#48969=CARTESIAN_POINT('Ctrl Pts',(36.1578669732689,-2.17699664626686,14.3732280248688));
#48970=CARTESIAN_POINT('Ctrl Pts',(36.0189554827803,-4.60322800024078,16.0999783031656));
#48971=CARTESIAN_POINT('Ctrl Pts',(35.8800439922917,-5.90795430179505,18.7769083330016));
#48972=CARTESIAN_POINT('Ctrl Pts',(35.741132501803,-5.773299239102,21.7518256630623));
#48973=CARTESIAN_POINT('Ctrl Pts',(35.6022210113144,-4.23206942811386,24.299937861598));
#48974=CARTESIAN_POINT('Ctrl Pts',(35.4633095208257,-1.65976158979958,25.8004369424213));
#48975=CARTESIAN_POINT('Ctrl Pts',(35.3243980303371,1.31692139757858,25.8877495947585));
#48976=CARTESIAN_POINT('Ctrl Pts',(35.1854865398485,3.97275692727123,24.5406034461069));
#48977=CARTESIAN_POINT('Ctrl Pts',(35.0465750493599,5.66069189550199,22.0872097456119));
#48978=CARTESIAN_POINT('Ctrl Pts',(34.9076635588712,5.96948714685048,19.1252997876036));
#48979=CARTESIAN_POINT('Ctrl Pts',(34.7687520683826,4.82390951134718,16.3764969595275));
#48980=CARTESIAN_POINT('Ctrl Pts',(34.6298405778939,2.50306119859119,14.5105044044023));
#48981=CARTESIAN_POINT('Ctrl Pts',(34.4909290874054,-0.427619123482817,
13.9819422449422));
#48982=CARTESIAN_POINT('Ctrl Pts',(34.3520175969166,-3.25411668348805,14.9195864471262));
#48983=CARTESIAN_POINT('Ctrl Pts',(34.2131061064281,-5.28779922292417,17.0949945549067));
#48984=CARTESIAN_POINT('Ctrl Pts',(34.0741946159393,-6.03319155723031,19.9781621488148));
#48985=CARTESIAN_POINT('Ctrl Pts',(33.9352831254508,-5.30869041389517,22.8666501962041));
#48986=CARTESIAN_POINT('Ctrl Pts',(33.7963716349621,-3.29080925101633,25.0567234185196));
#48987=CARTESIAN_POINT('Ctrl Pts',(33.6574601444735,-0.471173493020488,
26.0148044687633));
#48988=CARTESIAN_POINT('Ctrl Pts',(33.5185486539849,2.4632563731449,25.507471770072));
#48989=CARTESIAN_POINT('Ctrl Pts',(33.3796371634962,4.79755205787445,23.6583290598256));
#48990=CARTESIAN_POINT('Ctrl Pts',(33.2407256730076,5.96299864977798,20.9178912575711));
#48991=CARTESIAN_POINT('Ctrl Pts',(33.1018141825189,5.67565317642903,17.9538234976253));
#48992=CARTESIAN_POINT('Ctrl Pts',(32.9629026920303,4.00552290232418,15.488274882383));
#48993=CARTESIAN_POINT('Ctrl Pts',(32.8239912015417,1.35950914551882,14.1219380624878));
#48994=CARTESIAN_POINT('Ctrl Pts',(32.685079711053,-1.61772791272423,14.187699796262));
#48995=CARTESIAN_POINT('Ctrl Pts',(32.5461682205644,-4.20083067488945,15.6695382580044));
#48996=CARTESIAN_POINT('Ctrl Pts',(32.4072567300758,-5.76046624707371,18.2064265071361));
#48997=CARTESIAN_POINT('Ctrl Pts',(32.2683452395871,-5.91665363028091,21.1802910985275));
#48998=CARTESIAN_POINT('Ctrl Pts',(32.1294337490985,-4.63134019288346,23.8665960838652));
#48999=CARTESIAN_POINT('Ctrl Pts',(31.9905222586099,-2.21767260367744,25.6108649494421));
#49000=CARTESIAN_POINT('Ctrl Pts',(31.8516107681212,0.736296493406706,25.9881336601462));
#49001=CARTESIAN_POINT('Ctrl Pts',(31.7126992776326,3.51087837843202,24.9064865504593));
#49002=CARTESIAN_POINT('Ctrl Pts',(31.5737877871439,5.4300892412884,22.6294501496745));
#49003=CARTESIAN_POINT('Ctrl Pts',(31.4348762966553,6.02634314462065,19.7117890334094));
#49004=CARTESIAN_POINT('Ctrl Pts',(31.2959648061666,5.1543720797451,16.8643460456352));
#49005=CARTESIAN_POINT('Ctrl Pts',(31.157053315678,3.02661826216146,14.7808564732199));
#49006=CARTESIAN_POINT('Ctrl Pts',(31.0181418251894,0.161475883206934,13.9689302112211));
#49007=CARTESIAN_POINT('Ctrl Pts',(30.8792303347008,-2.74300758831371,14.6263804909137));
#49008=CARTESIAN_POINT('Ctrl Pts',(30.7403188442121,-4.9791998370319,16.5930297563846));
#49009=CARTESIAN_POINT('Ctrl Pts',(30.6014073537235,-6.00228733101139,19.3897344398054));
#49010=CARTESIAN_POINT('Ctrl Pts',(30.4624958632348,-5.56301068238225,22.3351208546198));
#49011=CARTESIAN_POINT('Ctrl Pts',(30.3235843727462,-3.76839282827076,24.7115913182084));
#49012=CARTESIAN_POINT('Ctrl Pts',(30.1846728822576,-1.0556645533444,25.9401556889354));
#49013=CARTESIAN_POINT('Ctrl Pts',(30.0457613917689,1.91426000431534,25.721493327258));
#49014=CARTESIAN_POINT('Ctrl Pts',(29.9068499012803,4.41780482445776,24.1088779235914));
#49015=CARTESIAN_POINT('Ctrl Pts',(29.7679384107917,5.84502007088054,21.4951981905363));
#49016=CARTESIAN_POINT('Ctrl Pts',(29.629026920303,5.84818690157327,18.5172366263472));
#49017=CARTESIAN_POINT('Ctrl Pts',(29.4901154298144,4.42653376739224,15.9005273431677));
#49018=CARTESIAN_POINT('Ctrl Pts',(29.3512039393257,1.92642438803342,14.2825909421164));
#49019=CARTESIAN_POINT('Ctrl Pts',(29.2122924488371,-1.04302839212392,14.0576125142159));
#49020=CARTESIAN_POINT('Ctrl Pts',(29.0733809583485,-3.75836349409478,15.2804045613808));
#49021=CARTESIAN_POINT('Ctrl Pts',(28.9344694678598,-5.55803166685062,17.6530527811079));
#49022=CARTESIAN_POINT('Ctrl Pts',(28.7955579773712,-6.00357169397569,20.5974982621509));
#49023=CARTESIAN_POINT('Ctrl Pts',(28.6566464868826,-4.9864346633914,23.3963725657984));
#49024=CARTESIAN_POINT('Ctrl Pts',(28.5177349963939,-2.75443022492254,25.3677734112025));
#49025=CARTESIAN_POINT('Ctrl Pts',(28.3788235059053,0.148648384459986,26.0313995818365));
#49026=CARTESIAN_POINT('Ctrl Pts',(28.2399120154167,3.01551112224173,25.2255688618193));
#49027=CARTESIAN_POINT('Ctrl Pts',(28.101000524928,5.14769138089252,23.1466093982356));
#49028=CARTESIAN_POINT('Ctrl Pts',(27.9620890344394,6.02571653541499,20.3010273954406));
#49029=CARTESIAN_POINT('Ctrl Pts',(27.8231775439507,5.43566938533659,17.3821047401979));
#49030=CARTESIAN_POINT('Ctrl Pts',(27.6842660534621,3.52130576024992,15.1009916308696));
#49031=CARTESIAN_POINT('Ctrl Pts',(27.5453545629735,0.749030643264908,14.0134458698321));
#49032=CARTESIAN_POINT('Ctrl Pts',(27.4064430724849,-2.20573416373653,14.3844311012236));
#49033=CARTESIAN_POINT('Ctrl Pts',(27.2675315819962,-4.62310607844673,16.1235625317299));
#49034=CARTESIAN_POINT('Ctrl Pts',(27.1286200915076,-5.91412995552358,18.8071277825525));
#49035=CARTESIAN_POINT('Ctrl Pts',(26.9897086010189,-5.76426786617869,21.7813178337734));
#49036=CARTESIAN_POINT('Ctrl Pts',(26.8507971105303,-4.21003138236937,24.3215174438436));
#49037=CARTESIAN_POINT('Ctrl Pts',(26.7118856200417,-1.63008609901205,25.8088464059387));
#49038=CARTESIAN_POINT('Ctrl Pts',(26.572974129553,1.34700436069226,25.8809401042907));
#49039=CARTESIAN_POINT('Ctrl Pts',(26.4340626390644,3.99591811568663,24.5202340283117));
#49040=CARTESIAN_POINT('Ctrl Pts',(26.2951511485758,5.67128844516229,22.0582430929674));
#49041=CARTESIAN_POINT('Ctrl Pts',(26.1562396580871,5.9649373729072,19.0947931754155));
#49042=CARTESIAN_POINT('Ctrl Pts',(26.0173281675985,4.80532189560143,16.3518828503414));
#49043=CARTESIAN_POINT('Ctrl Pts',(25.8784166771098,2.47496432510841,14.4977796438692));
#49044=CARTESIAN_POINT('Ctrl Pts',(25.7395051866212,-0.458379887589252,
13.9842070234562));
#49045=CARTESIAN_POINT('Ctrl Pts',(25.6005936961326,-3.28004695550241,14.9362889865555));
#49046=CARTESIAN_POINT('Ctrl Pts',(25.4616822056439,-5.30258149455159,17.1220655407709));
#49047=CARTESIAN_POINT('Ctrl Pts',(25.3227707151553,-6.03322435743451,20.0090061555954));
#49048=CARTESIAN_POINT('Ctrl Pts',(25.1838592246667,-5.29396575141546,22.8937525603996));
#49049=CARTESIAN_POINT('Ctrl Pts',(25.044947734178,-3.2649145613144,25.0734810697683));
#49050=CARTESIAN_POINT('Ctrl Pts',(24.9060362436894,-0.440417615313074,
26.0171346654451));
#49051=CARTESIAN_POINT('Ctrl Pts',(24.7671247532008,2.49138024663732,25.4948067959342));
#49052=CARTESIAN_POINT('Ctrl Pts',(24.6282132627121,4.81619198190525,23.633754539235));
#49053=CARTESIAN_POINT('Ctrl Pts',(24.4893017722235,5.96761329618002,20.8873943910319));
#49054=CARTESIAN_POINT('Ctrl Pts',(24.3503902817348,5.66511825823355,17.9248343733069));
#49055=CARTESIAN_POINT('Ctrl Pts',(24.2114787912462,3.98240508882984,15.4678562504658));
#49056=CARTESIAN_POINT('Ctrl Pts',(24.0725673007576,1.32944073315618,14.1150646057068));
#49057=CARTESIAN_POINT('Ctrl Pts',(23.9336558102689,-1.64742122199533,14.1960461256744));
#49058=CARTESIAN_POINT('Ctrl Pts',(23.7947443197803,-4.2229145671552,15.6910709199979));
#49059=CARTESIAN_POINT('Ctrl Pts',(23.6558328292916,-5.7695603247627,18.235899402839));
#49060=CARTESIAN_POINT('Ctrl Pts',(23.516921338803,-5.91054226251958,21.2105236143708));
#49061=CARTESIAN_POINT('Ctrl Pts',(23.3780098483144,-4.61151231956818,23.8902225366231));
#49062=CARTESIAN_POINT('Ctrl Pts',(23.2390983578258,-2.1889589783795,25.6221291206225));
#49063=CARTESIAN_POINT('Ctrl Pts',(23.1001868673371,0.766900241567219,25.9842912092798));
#49064=CARTESIAN_POINT('Ctrl Pts',(22.9612753768485,3.5359161212374,24.8884736310584));
#49065=CARTESIAN_POINT('Ctrl Pts',(22.8223638863598,5.44346092133198,22.6016553299603));
#49066=CARTESIAN_POINT('Ctrl Pts',(22.6834523958712,6.02479095961078,19.6809840897829));
#49067=CARTESIAN_POINT('Ctrl Pts',(22.5445409053826,5.13827419546692,16.8380361244666));
#49068=CARTESIAN_POINT('Ctrl Pts',(22.4056294148939,2.99989667825315,14.7654515784277));
#49069=CARTESIAN_POINT('Ctrl Pts',(22.2667179244053,0.130640898823814,13.9681835063114));
#49070=CARTESIAN_POINT('Ctrl Pts',(22.1278064339167,-2.77044350783753,14.6404738989477));
#49071=CARTESIAN_POINT('Ctrl Pts',(21.988894943428,-4.99655235575603,16.6185296372483));
#49072=CARTESIAN_POINT('Ctrl Pts',(21.8499834529394,-6.00532877708893,19.4204281433272));
#49073=CARTESIAN_POINT('Ctrl Pts',(21.7110719624507,-5.55100005468478,22.3635303363547));
#49074=CARTESIAN_POINT('Ctrl Pts',(21.5721604719621,-3.74425632981162,24.7307950488945));
#49075=CARTESIAN_POINT('Ctrl Pts',(21.4332489814735,-1.02528266733415,25.9454749776653));
#49076=CARTESIAN_POINT('Ctrl Pts',(21.2943374909848,1.94348520292825,25.7116322118969));
#49077=CARTESIAN_POINT('Ctrl Pts',(21.1554260004962,4.43875306965556,24.0862389118361));
#49078=CARTESIAN_POINT('Ctrl Pts',(21.0165145100075,5.85258764787277,21.4652969262053));
#49079=CARTESIAN_POINT('Ctrl Pts',(20.877603019519,5.84053008768728,18.4873580883768));
#49080=CARTESIAN_POINT('Ctrl Pts',(20.7386915290303,4.4055180264847,15.8779509735693));
#49081=CARTESIAN_POINT('Ctrl Pts',(20.5997800385417,1.89716987917683,14.2728171229195));
#49082=CARTESIAN_POINT('Ctrl Pts',(20.460868548053,-1.07339426192582,14.0630224847618));
#49083=CARTESIAN_POINT('Ctrl Pts',(20.3219570575644,-3.78244255199411,15.2996802663177));
#49084=CARTESIAN_POINT('Ctrl Pts',(20.1830455670757,-5.56995742413767,17.6814979941192));
#49085=CARTESIAN_POINT('Ctrl Pts',(20.0441340765871,-6.00043862499533,20.628182748604));
#49086=CARTESIAN_POINT('Ctrl Pts',(19.9052225860985,-4.96900609177015,23.421820526844));
#49087=CARTESIAN_POINT('Ctrl Pts',(19.7663110956098,-2.72695235161518,25.3817848461268));
#49088=CARTESIAN_POINT('Ctrl Pts',(19.6273996051212,0.179481002124917,26.0305608220012));
#49089=CARTESIAN_POINT('Ctrl Pts',(19.4884881146326,3.04218659554424,25.2100842580395));
#49090=CARTESIAN_POINT('Ctrl Pts',(19.3495766241439,5.16371064481064,23.1202515338749));
#49091=CARTESIAN_POINT('Ctrl Pts',(19.2106651336553,6.02717674494101,20.2702179550323));
#49092=CARTESIAN_POINT('Ctrl Pts',(19.0717536431667,5.42221478308436,17.3543499656831));
#49093=CARTESIAN_POINT('Ctrl Pts',(18.932842152678,3.49621435122019,15.083053542258));
#49094=CARTESIAN_POINT('Ctrl Pts',(18.7939306621894,0.718415559806878,14.0096948039848));
#49095=CARTESIAN_POINT('Ctrl Pts',(18.6550191717007,-2.23441403173588,14.3957809471112));
#49096=CARTESIAN_POINT('Ctrl Pts',(18.5161076812121,-4.6428633263092,16.1472480755708));
#49097=CARTESIAN_POINT('Ctrl Pts',(18.3771961907235,-5.92015103647305,18.8373784092292));
#49098=CARTESIAN_POINT('Ctrl Pts',(18.2382847002349,-5.7550858372992,21.8107634476368));
#49099=CARTESIAN_POINT('Ctrl Pts',(18.0993732097462,-4.18788330247692,24.3429840781212));
#49100=CARTESIAN_POINT('Ctrl Pts',(17.9604617192576,-1.60036800399696,25.8171040483872));
#49101=CARTESIAN_POINT('Ctrl Pts',(17.8215502287689,1.37705211825441,25.8739769084999));
#49102=CARTESIAN_POINT('Ctrl Pts',(17.6826387382803,4.01897486605748,24.4997464688555));
#49103=CARTESIAN_POINT('Ctrl Pts',(17.5437272477917,5.68173676899357,22.029222645706));
#49104=CARTESIAN_POINT('Ctrl Pts',(17.404815757303,5.96023169827291,19.0643102218779));
#49105=CARTESIAN_POINT('Ctrl Pts',(17.2659042668144,4.78660868708628,16.3273640890105));
#49106=CARTESIAN_POINT('Ctrl Pts',(17.1269927763257,2.44680276550663,14.4851986903707));
#49107=CARTESIAN_POINT('Ctrl Pts',(16.9880812858371,-0.489128671395442,
13.9866290318326));
#49108=CARTESIAN_POINT('Ctrl Pts',(16.8491697953485,-3.30589149961142,14.9531238720594));
#49109=CARTESIAN_POINT('Ctrl Pts',(16.7102583048598,-5.31722517694209,17.149211744855));
#49110=CARTESIAN_POINT('Ctrl Pts',(16.5713468143712,-6.03309947218664,20.0398499269894));
#49111=CARTESIAN_POINT('Ctrl Pts',(16.4324353238826,-5.27910272488139,22.9207792929506));
#49112=CARTESIAN_POINT('Ctrl Pts',(16.2935238333939,-3.23893453920998,25.0901061195905));
#49113=CARTESIAN_POINT('Ctrl Pts',(16.1546123429053,-0.409650226770401,
26.019307597198));
#49114=CARTESIAN_POINT('Ctrl Pts',(16.0157008524167,2.51943900496133,25.4819982085239));
#49115=CARTESIAN_POINT('Ctrl Pts',(15.876789361928,4.83470602906412,23.6090850461731));
#49116=CARTESIAN_POINT('Ctrl Pts',(15.7378778714394,5.9720719719527,20.856874331391));
#49117=CARTESIAN_POINT('Ctrl Pts',(15.5989663809507,5.65443527547411,17.8958994858958));
#49118=CARTESIAN_POINT('Ctrl Pts',(15.4600548904621,3.95918319046976,15.4475560714841));
#49119=CARTESIAN_POINT('Ctrl Pts',(15.3211433999735,1.299337574288,14.1083449586705));
#49120=CARTESIAN_POINT('Ctrl Pts',(15.1822319094849,-1.67707147396502,14.2045441482838));
#49121=CARTESIAN_POINT('Ctrl Pts',(15.0433204189962,-4.24488808855577,15.7127162009476));
#49122=CARTESIAN_POINT('Ctrl Pts',(14.9044089285076,-5.77850360817088,18.265418405397));
#49123=CARTESIAN_POINT('Ctrl Pts',(14.7654974380189,-5.90427641574779,21.2407244917482));
#49124=CARTESIAN_POINT('Ctrl Pts',(14.6265859475303,-4.59156391892589,23.9137473138154));
#49125=CARTESIAN_POINT('Ctrl Pts',(14.4876744570417,-2.16018814205056,25.6332463508108));
#49126=CARTESIAN_POINT('Ctrl Pts',(14.348762966553,0.797483945883081,25.980292351887));
#49127=CARTESIAN_POINT('Ctrl Pts',(14.2098514760644,3.56086144869418,24.8703329456191));
#49128=CARTESIAN_POINT('Ctrl Pts',(14.0709399855757,5.45669033008824,22.573792512908));
#49129=CARTESIAN_POINT('Ctrl Pts',(13.9320284950871,6.02308130956567,19.6501874840145));
#49130=CARTESIAN_POINT('Ctrl Pts',(13.7931170045985,5.12204201631729,16.8118088449625));
#49131=CARTESIAN_POINT('Ctrl Pts',(13.6542055141098,2.97309668849815,14.7501834947476));
#49132=CARTESIAN_POINT('Ctrl Pts',(13.5152940236212,0.0998024999863045,
13.9675944500576));
#49133=CARTESIAN_POINT('Ctrl Pts',(13.3763825331326,-2.79780701854458,14.6547073845334));
#49134=CARTESIAN_POINT('Ctrl Pts',(13.2374710426439,-5.01377428367657,16.644117896838));
#49135=CARTESIAN_POINT('Ctrl Pts',(13.0985595521553,-6.00821326679838,19.4511369946448));
#49136=CARTESIAN_POINT('Ctrl Pts',(12.9596480616667,-5.53884434503756,22.3918780444297));
#49137=CARTESIAN_POINT('Ctrl Pts',(12.820736571178,-3.72002197078624,24.7498751346585));
#49138=CARTESIAN_POINT('Ctrl Pts',(12.6818250806894,-0.994873984349104,
25.9506388743768));
#49139=CARTESIAN_POINT('Ctrl Pts',(12.5429135902007,1.97265960625756,25.7016218162747));
#49140=CARTESIAN_POINT('Ctrl Pts',(12.4040020997121,4.45958530279366,24.0634931013951));
#49141=CARTESIAN_POINT('Ctrl Pts',(12.2650906092235,5.8600022605669,21.4353573646065));
#49142=CARTESIAN_POINT('Ctrl Pts',(12.1261791187349,5.83272062464183,18.4575190850913));
#49143=CARTESIAN_POINT('Ctrl Pts',(11.9872676282462,4.38438714215463,15.8554823385961));
#49144=CARTESIAN_POINT('Ctrl Pts',(11.8483561377576,1.86786578554228,14.2631929904188));
#49145=CARTESIAN_POINT('Ctrl Pts',(11.7094446472689,-1.10373207729958,14.0685876252347));
#49146=CARTESIAN_POINT('Ctrl Pts',(11.5705331567803,-3.80642275128512,15.3190788196683));
#49147=CARTESIAN_POINT('Ctrl Pts',(11.4316216662916,-5.58173760400173,17.7100038039218));
#49148=CARTESIAN_POINT('Ctrl Pts',(11.292710175803,-5.99714872745679,20.6588508167584));
#49149=CARTESIAN_POINT('Ctrl Pts',(11.1537986853144,-4.9514476492995,23.4471790545641));
#49150=CARTESIAN_POINT('Ctrl Pts',(11.0148871948257,-2.69940320618387,25.3956556217409));
#49151=CARTESIAN_POINT('Ctrl Pts',(10.8759757043371,0.210308928841623,26.0295644463285));
#49152=CARTESIAN_POINT('Ctrl Pts',(10.7370642138485,3.06878255770306,25.1944634825473));
#49153=CARTESIAN_POINT('Ctrl Pts',(10.5981527233599,5.17959494904565,23.0938121180512));
#49154=CARTESIAN_POINT('Ctrl Pts',(10.4592412328712,6.02847942707646,20.2394014521583));
#49155=CARTESIAN_POINT('Ctrl Pts',(10.3203297423826,5.40861846483775,17.3266643383601));
#49156=CARTESIAN_POINT('Ctrl Pts',(10.1814182518939,3.4710315644946,15.0652439638558));
#49157=CARTESIAN_POINT('Ctrl Pts',(10.0425067614053,0.687781699708797,14.0061003018464));
#49158=CARTESIAN_POINT('Ctrl Pts',(9.90359527091665,-2.26303550068255,14.4072772658901));
#49159=CARTESIAN_POINT('Ctrl Pts',(9.76468378042802,-4.66249922744889,16.1710343156385));
#49160=CARTESIAN_POINT('Ctrl Pts',(9.62577228993938,-5.92601738727541,18.8676594223957));
#49161=CARTESIAN_POINT('Ctrl Pts',(9.48686079945074,-5.74575339244678,21.8401617350564));
#49162=CARTESIAN_POINT('Ctrl Pts',(9.34794930896211,-4.16562576730276,24.364337203375));
#49163=CARTESIAN_POINT('Ctrl Pts',(9.20903781847347,-1.57060808147196,25.8252096539433));
#49164=CARTESIAN_POINT('Ctrl Pts',(9.07012632798484,1.40706388493112,25.8668601893775));
#49165=CARTESIAN_POINT('Ctrl Pts',(8.9312148374962,4.04192657576827,24.4791413032051));
#49166=CARTESIAN_POINT('Ctrl Pts',(8.79230334700756,5.69203659391647,22.0001491623115));
#49167=CARTESIAN_POINT('Ctrl Pts',(8.65339185651892,5.95537024593603,19.0338517236991));
#49168=CARTESIAN_POINT('Ctrl Pts',(8.51448036603028,4.7677703748936,16.3029413163616));
#49169=CARTESIAN_POINT('Ctrl Pts',(8.37556887554165,2.41857725582169,14.472761872725));
#49170=CARTESIAN_POINT('Ctrl Pts',(8.23665738505301,-0.519864671245333,
13.9892082067692));
#49171=CARTESIAN_POINT('Ctrl Pts',(8.09774589456439,-3.33164964033728,14.9700906636381));
#49172=CARTESIAN_POINT('Ctrl Pts',(7.95883440407574,-5.3317298873657,17.1764324576609));
#49173=CARTESIAN_POINT('Ctrl Pts',(7.8199229135871,-6.03281690475071,20.0706926568584));
#49174=CARTESIAN_POINT('Ctrl Pts',(7.68101142309848,-5.26410172275582,22.9477296874813));
#49175=CARTESIAN_POINT('Ctrl Pts',(7.54209993260984,-3.21286986372191,25.1065981334708));
#49176=CARTESIAN_POINT('Ctrl Pts',(7.4031884421212,-0.378872131534907,26.0213232072299));
#49177=CARTESIAN_POINT('Ctrl Pts',(7.26427695163256,2.547431914768,25.4690463426086));
#49178=CARTESIAN_POINT('Ctrl Pts',(7.12536546114393,4.8530937154645,23.5843212254063));
#49179=CARTESIAN_POINT('Ctrl Pts',(6.98645397065529,5.97637456056316,20.8263318763263));
#49180=CARTESIAN_POINT('Ctrl Pts',(6.84754248016666,5.64360450736318,17.8670195916395));
#49181=CARTESIAN_POINT('Ctrl Pts',(6.70863098967801,3.93585781417588,15.4273748760072));
#49182=CARTESIAN_POINT('Ctrl Pts',(6.56971949918939,1.26920045569606,14.1017792970049));
#49183=CARTESIAN_POINT('Ctrl Pts',(6.43080800870073,-1.7066778936888,14.2131936419841));
#49184=CARTESIAN_POINT('Ctrl Pts',(6.29189651821211,-4.26675066478705,15.7344735351286));
#49185=CARTESIAN_POINT('Ctrl Pts',(6.15298502772347,-5.7872958635549,18.2949827432956));
#49186=CARTESIAN_POINT('Ctrl Pts',(6.01407353723484,-5.8978562537309,21.270892941324));
#49187=CARTESIAN_POINT('Ctrl Pts',(5.87516204674619,-4.57149551233171,23.9371698005941));
#49188=CARTESIAN_POINT('Ctrl Pts',(5.73625055625756,-2.13136084665032,25.6442163494453));
#49189=CARTESIAN_POINT('Ctrl Pts',(5.59733906576892,0.82804680701318,25.9761371924827));
#49190=CARTESIAN_POINT('Ctrl Pts',(5.45842757528028,3.58571370882673,24.8520649682698));
#49191=CARTESIAN_POINT('Ctrl Pts',(5.31951608479165,5.46977712179084,22.5458624267452));
#49192=CARTESIAN_POINT('Ctrl Pts',(5.18060459430302,6.02121423916907,19.6194000210098));
#49193=CARTESIAN_POINT('Ctrl Pts',(5.04169310381438,5.10567596654349,16.7856648926038));
#49194=CARTESIAN_POINT('Ctrl Pts',(4.90278161332574,2.94621899334588,14.735052621229));
#49195=CARTESIAN_POINT('Ctrl Pts',(4.76387012283711,0.0689614926924268,
13.9671630578554));
#49196=CARTESIAN_POINT('Ctrl Pts',(4.62495863234847,-2.8250974052572,14.6690805756616));
#49197=CARTESIAN_POINT('Ctrl Pts',(4.48604714185984,-5.03086517067809,16.6697938663744));
#49198=CARTESIAN_POINT('Ctrl Pts',(4.34713565137119,-6.01094072475019,19.4818601911461));
#49199=CARTESIAN_POINT('Ctrl Pts',(4.20822416088256,-5.52654387114446,22.4201632379438));
#49200=CARTESIAN_POINT('Ctrl Pts',(4.06931267039393,-3.69569038458819,24.76883107682));
#49201=CARTESIAN_POINT('Ctrl Pts',(3.93040117990529,-0.964439299156375,
25.9556472441051));
#49202=CARTESIAN_POINT('Ctrl Pts',(3.79148968941666,2.0017824517957,25.6914624020259));
#49203=CARTESIAN_POINT('Ctrl Pts',(3.65257819892801,4.48030097939669,24.0406410867557));
#49204=CARTESIAN_POINT('Ctrl Pts',(3.51366670843938,5.86726371517407,21.4053802882495));
#49205=CARTESIAN_POINT('Ctrl Pts',(3.37475521795074,5.82475871654497,18.4277203963609));
#49206=CARTESIAN_POINT('Ctrl Pts',(3.2358437274621,4.36314166668535,15.8331220255067));
#49207=CARTESIAN_POINT('Ctrl Pts',(3.09693223697347,1.83851287302163,14.2537187961239));
#49208=CARTESIAN_POINT('Ctrl Pts',(2.95802074648483,-1.13404104531969,14.074307790239));
#49209=CARTESIAN_POINT('Ctrl Pts',(2.81910925599619,-3.83030346523787,15.3385997143183));
#49210=CARTESIAN_POINT('Ctrl Pts',(2.68019776550755,-5.5933718985126,17.7385694656995));
#49211=CARTESIAN_POINT('Ctrl Pts',(2.54128627501892,-5.99370208742667,20.6895016646407));
#49212=CARTESIAN_POINT('Ctrl Pts',(2.40237478453029,-4.93375979473011,23.4724474870243));
#49213=CARTESIAN_POINT('Ctrl Pts',(2.26346329404166,-2.67178350897306,25.4093853738612));
#49214=CARTESIAN_POINT('Ctrl Pts',(2.12455180355301,0.241131359505999,26.028410484117));
#49215=CARTESIAN_POINT('Ctrl Pts',(1.98564031306438,3.09529831238036,25.1787069371976));
#49216=CARTESIAN_POINT('Ctrl Pts',(1.84672882257574,5.19534388084631,23.0672918544148));
#49217=CARTESIAN_POINT('Ctrl Pts',(1.70781733208711,6.02962454304153,20.2085786673882));
#49218=CARTESIAN_POINT('Ctrl Pts',(1.56890584159847,5.39488079527025,17.2990486307619));
#49219=CARTESIAN_POINT('Ctrl Pts',(1.42999435110983,3.44575803991071,15.047563264792));
#49220=CARTESIAN_POINT('Ctrl Pts',(1.2910828606212,0.65712989973888,14.0026626470471));
#49221=CARTESIAN_POINT('Ctrl Pts',(1.15217137013255,-2.29159789362567,14.4189193836441));
#49222=CARTESIAN_POINT('Ctrl Pts',(1.01325987964392,-4.68201312866807,16.1949213654875));
#49223=CARTESIAN_POINT('Ctrl Pts',(0.874348389155287,-5.93172913021799,
18.8979685830992));
#49224=CARTESIAN_POINT('Ctrl Pts',(0.735436898666651,-5.73627023291581,
21.8695147775384));
#49225=CARTESIAN_POINT('Ctrl Pts',(0.596525408178009,-4.14326042687647,
24.3855706507271));
#49226=CARTESIAN_POINT('Ctrl Pts',(0.457613917689371,-1.54080500599549,
25.833174057334));
#49227=CARTESIAN_POINT('Ctrl Pts',(0.318702427200732,1.43703473556815,25.8595683830997));
#49228=CARTESIAN_POINT('Ctrl Pts',(0.179790936712099,4.06478079616032,24.4584619074674));
#49229=CARTESIAN_POINT('Ctrl Pts',(0.0408794462234644,5.70217161488762,
21.9709388731352));
#49230=CARTESIAN_POINT('Ctrl Pts',(-0.0980320442651723,5.95038457493443,
19.0035870828949));
#49231=CARTESIAN_POINT('Ctrl Pts',(-0.236943534753798,4.74874707354515,
16.278258531722));
#49232=CARTESIAN_POINT('Ctrl Pts',(-0.329551195079558,3.17650145787956,
15.0670768494447));
#49233=CARTESIAN_POINT('Ctrl Pts',(-0.375855025242435,2.29303208829606,
14.6858628259571));
#49234=CARTESIAN_POINT('Ctrl Pts',(50.3758550252424,-1.41074674833726,14.7230720419399));
#49235=CARTESIAN_POINT('Ctrl Pts',(50.3295511950796,-2.2880301273243,14.9576071131239));
#49236=CARTESIAN_POINT('Ctrl Pts',(50.2369435347538,-3.92247867381803,15.8724340640267));
#49237=CARTESIAN_POINT('Ctrl Pts',(50.0980320442652,-5.41896188543471,18.2519519775424));
#49238=CARTESIAN_POINT('Ctrl Pts',(49.9591205537766,-5.59497493220745,21.0566843253696));
#49239=CARTESIAN_POINT('Ctrl Pts',(49.8202090632879,-4.40797189480199,23.6042986761457));
#49240=CARTESIAN_POINT('Ctrl Pts',(49.6812975727993,-2.14697777410166,25.2736168556974));
#49241=CARTESIAN_POINT('Ctrl Pts',(49.5423860823106,0.637065137223345,25.6581837149789));
#49242=CARTESIAN_POINT('Ctrl Pts',(49.403474591822,3.26591175511246,24.6641794978917));
#49243=CARTESIAN_POINT('Ctrl Pts',(49.2645631013333,5.09906218008006,22.533841897014));
#49244=CARTESIAN_POINT('Ctrl Pts',(49.1256516108447,5.68990905334285,19.7861620991407));
#49245=CARTESIAN_POINT('Ctrl Pts',(48.9867401203561,4.89449597134713,17.090586147606));
#49246=CARTESIAN_POINT('Ctrl Pts',(48.8478286298675,2.90661589773406,15.1038408976722));
#49247=CARTESIAN_POINT('Ctrl Pts',(48.7089171393788,0.210583477931158,14.3099702510581));
#49248=CARTESIAN_POINT('Ctrl Pts',(48.5700056488901,-2.5367540845736,14.9023863052417));
#49249=CARTESIAN_POINT('Ctrl Pts',(48.4310941584015,-4.6660510176104,16.7367571827446));
#49250=CARTESIAN_POINT('Ctrl Pts',(48.2921826679129,-5.65853697987053,19.3661663336582));
#49251=CARTESIAN_POINT('Ctrl Pts',(48.1532711774243,-5.27240827015851,22.1499993147008));
#49252=CARTESIAN_POINT('Ctrl Pts',(48.0143596869356,-3.60173910521923,24.4100182858197));
#49253=CARTESIAN_POINT('Ctrl Pts',(47.8754481964471,-1.05356212089668,25.5956047771332));
#49254=CARTESIAN_POINT('Ctrl Pts',(47.7365367059583,1.75129892547251,25.4179090051804));
#49255=CARTESIAN_POINT('Ctrl Pts',(47.5976252154698,4.12948316954712,23.9202238055293));
#49256=CARTESIAN_POINT('Ctrl Pts',(47.458713724981,5.50158293700532,21.467436920898));
#49257=CARTESIAN_POINT('Ctrl Pts',(47.3198022344925,5.53330741511091,18.6571318092182));
#49258=CARTESIAN_POINT('Ctrl Pts',(47.1808907440037,4.21692742804939,16.1739956878171));
#49259=CARTESIAN_POINT('Ctrl Pts',(47.0419792535153,1.87315852680124,14.6230061314821));
#49260=CARTESIAN_POINT('Ctrl Pts',(46.9030677630264,-0.926976374857329,
14.3820376710101));
#49261=CARTESIAN_POINT('Ctrl Pts',(46.764156272538,-3.50126787105187,15.5097985318837));
#49262=CARTESIAN_POINT('Ctrl Pts',(46.6252447820492,-5.22252979601018,17.7315272849312));
#49263=CARTESIAN_POINT('Ctrl Pts',(46.4863332915607,-5.67140339862458,20.5059342045224));
#49264=CARTESIAN_POINT('Ctrl Pts',(46.3474218010719,-4.73852759287644,23.157078108117));
#49265=CARTESIAN_POINT('Ctrl Pts',(46.2085103105834,-2.65118308904264,25.0390489338371));
#49266=CARTESIAN_POINT('Ctrl Pts',(46.0695988200946,0.0820810236181339,
25.6933337013367));
#49267=CARTESIAN_POINT('Ctrl Pts',(45.9306873296062,2.79534736890921,24.9605260826201));
#49268=CARTESIAN_POINT('Ctrl Pts',(45.7917758391174,4.82757071625747,23.019163279578));
#49269=CARTESIAN_POINT('Ctrl Pts',(45.6528643486289,5.68363139060459,20.3422282059583));
#49270=CARTESIAN_POINT('Ctrl Pts',(45.5139528581401,5.15496349614729,17.5819145419136));
#49271=CARTESIAN_POINT('Ctrl Pts',(45.3750413676516,3.37036875955527,15.4107298669796));
#49272=CARTESIAN_POINT('Ctrl Pts',(45.2361298771628,0.764635988488109,14.3576496267665));
#49273=CARTESIAN_POINT('Ctrl Pts',(45.0972183866743,-2.02738847273789,14.6792404762263));
#49274=CARTESIAN_POINT('Ctrl Pts',(44.9583068961856,-4.32547120105949,16.2971517965187));
#49275=CARTESIAN_POINT('Ctrl Pts',(44.819395405697,-5.56972000982934,18.8172046071589));
#49276=CARTESIAN_POINT('Ctrl Pts',(44.6804839152083,-5.45699298962439,21.6254271562914));
#49277=CARTESIAN_POINT('Ctrl Pts',(44.5415724247197,-4.01475432920467,24.0376396081562));
#49278=CARTESIAN_POINT('Ctrl Pts',(44.4026609342311,-1.59438309221228,25.4661438404498));
#49279=CARTESIAN_POINT('Ctrl Pts',(44.2637494437424,1.21443483769103,25.5629069697615));
#49280=CARTESIAN_POINT('Ctrl Pts',(44.1248379532538,3.72737456946171,24.3043541615613));
#49281=CARTESIAN_POINT('Ctrl Pts',(43.9859264627651,5.33219734250401,21.9971122727109));
#49282=CARTESIAN_POINT('Ctrl Pts',(43.8470149722766,5.63791299771413,19.2033049771553));
#49283=CARTESIAN_POINT('Ctrl Pts',(43.7081034817879,4.57003866092117,16.6036000578693));
#49284=CARTESIAN_POINT('Ctrl Pts',(43.5691919912993,2.3887453390794,14.8313752666453));
#49285=CARTESIAN_POINT('Ctrl Pts',(43.4302805008106,-0.374528707284711,
14.3184056659561));
#49286=CARTESIAN_POINT('Ctrl Pts',(43.291369010322,-3.04655464743421,15.189668336859));
#49287=CARTESIAN_POINT('Ctrl Pts',(43.1524575198333,-4.97633483538731,17.2328936530502));
#49288=CARTESIAN_POINT('Ctrl Pts',(43.0135460293447,-5.69370828178274,19.9502814805321));
#49289=CARTESIAN_POINT('Ctrl Pts',(42.8746345388561,-5.0238980812484,22.6797824535675));
#49290=CARTESIAN_POINT('Ctrl Pts',(42.7357230483674,-3.13009309256387,24.7563960265209));
#49291=CARTESIAN_POINT('Ctrl Pts',(42.5968115578789,-0.473689506184257,
25.6741875348767));
#49292=CARTESIAN_POINT('Ctrl Pts',(42.4579000673901,2.29812117591949,25.2095513232916));
#49293=CARTESIAN_POINT('Ctrl Pts',(42.3189885769016,4.51003030421545,23.4756887927831));
#49294=CARTESIAN_POINT('Ctrl Pts',(42.1800770864129,5.62314055214332,20.8950286364474));
#49295=CARTESIAN_POINT('Ctrl Pts',(42.0411655959243,5.36625988513824,18.0963086451907));
#49296=CARTESIAN_POINT('Ctrl Pts',(41.9022541054356,3.8019732904961,15.7613935040425));
#49297=CARTESIAN_POINT('Ctrl Pts',(41.763342614947,1.31139491664314,14.4591490453341));
#49298=CARTESIAN_POINT('Ctrl Pts',(41.6244311244583,-1.49868447359569,14.5068469184063));
#49299=CARTESIAN_POINT('Ctrl Pts',(41.4855196339697,-3.94363265394602,15.8928662768361));
#49300=CARTESIAN_POINT('Ctrl Pts',(41.3466081434811,-5.42777594997247,18.2795250172932));
#49301=CARTESIAN_POINT('Ctrl Pts',(41.2076966529924,-5.58952588399778,21.0853507826221));
#49302=CARTESIAN_POINT('Ctrl Pts',(41.0687851625038,-4.38947459522761,23.6267476762343));
#49303=CARTESIAN_POINT('Ctrl Pts',(40.9298736720151,-2.11999595335694,25.2845437917544));
#49304=CARTESIAN_POINT('Ctrl Pts',(40.7909621815266,0.665986796647139,25.6548428374192));
#49305=CARTESIAN_POINT('Ctrl Pts',(40.6520506910379,3.28971220088311,24.6474271984164));
#49306=CARTESIAN_POINT('Ctrl Pts',(40.5131392005492,5.11195028923897,22.5077380584042));
#49307=CARTESIAN_POINT('Ctrl Pts',(40.3742277100607,5.68874103568606,19.7570774647734));
#49308=CARTESIAN_POINT('Ctrl Pts',(40.235316219572,4.87955832761485,17.0656011762843));
#49309=CARTESIAN_POINT('Ctrl Pts',(40.0964047290834,2.88154697197056,15.0890456143895));
#49310=CARTESIAN_POINT('Ctrl Pts',(39.9574932385947,0.181491423060029,14.3089678622789));
#49311=CARTESIAN_POINT('Ctrl Pts',(39.8185817481061,-2.56278169402701,14.9154217561356));
#49312=CARTESIAN_POINT('Ctrl Pts',(39.6796702576174,-4.68267283004561,16.7606542179057));
#49313=CARTESIAN_POINT('Ctrl Pts',(39.5407587671288,-5.66170341397994,19.3951029993896));
#49314=CARTESIAN_POINT('Ctrl Pts',(39.4018472766402,-5.26134784025525,22.1769255460536));
#49315=CARTESIAN_POINT('Ctrl Pts',(39.2629357861515,-3.57914653021792,24.4283739729666));
#49316=CARTESIAN_POINT('Ctrl Pts',(39.1240242956629,-1.02494172246551,25.6009178171769));
#49317=CARTESIAN_POINT('Ctrl Pts',(38.9851128051742,1.77897422714662,25.4088849708944));
#49318=CARTESIAN_POINT('Ctrl Pts',(38.8462013146857,4.14947071898586,23.8990612564435));
#49319=CARTESIAN_POINT('Ctrl Pts',(38.707289824197,5.50901307690715,21.4392917868471));
#49320=CARTESIAN_POINT('Ctrl Pts',(38.5683783337084,5.52636990778647,18.6288612136141));
#49321=CARTESIAN_POINT('Ctrl Pts',(38.4294668432197,4.19731248918724,16.1524873233045));
#49322=CARTESIAN_POINT('Ctrl Pts',(38.2905553527311,1.84564503194526,14.6135001768054));
#49323=CARTESIAN_POINT('Ctrl Pts',(38.1516438622425,-0.955685189815839,
14.3868501046929));
#49324=CARTESIAN_POINT('Ctrl Pts',(38.0127323717538,-3.52417754891945,15.527756879047));
#49325=CARTESIAN_POINT('Ctrl Pts',(37.8738208812652,-5.23405874939034,17.7582562730879));
#49326=CARTESIAN_POINT('Ctrl Pts',(37.7349093907765,-5.66874277696523,20.5349217305587));
#49327=CARTESIAN_POINT('Ctrl Pts',(37.5959979002879,-4.72232561535253,23.1812618112637));
#49328=CARTESIAN_POINT('Ctrl Pts',(37.4570864097993,-2.62538711599339,25.0525368301869));
#49329=CARTESIAN_POINT('Ctrl Pts',(37.3181749193106,0.111186203754847,25.6928396743027));
#49330=CARTESIAN_POINT('Ctrl Pts',(37.179263428822,2.82067073075507,24.9461704942188));
#49331=CARTESIAN_POINT('Ctrl Pts',(37.0403519383333,4.84294261575957,22.9944436461018));
#49332=CARTESIAN_POINT('Ctrl Pts',(36.9014404478447,5.68530670304713,20.3131670824126));
#49333=CARTESIAN_POINT('Ctrl Pts',(36.7625289573561,5.14253405765722,17.5555922199733));
#49334=CARTESIAN_POINT('Ctrl Pts',(36.6236174668674,3.34686280989496,15.3935593718185));
#49335=CARTESIAN_POINT('Ctrl Pts',(36.4847059763788,0.735780387440389,14.3538142830157));
#49336=CARTESIAN_POINT('Ctrl Pts',(36.3457944858902,-2.05456350586516,14.6896747058597));
#49337=CARTESIAN_POINT('Ctrl Pts',(36.2068829954015,-4.34434489124707,16.3193134614429));
#49338=CARTESIAN_POINT('Ctrl Pts',(36.0679715049129,-5.57569407541445,18.8456943617015));
#49339=CARTESIAN_POINT('Ctrl Pts',(35.9290600144243,-5.44861194225475,21.6533039139669));
#49340=CARTESIAN_POINT('Ctrl Pts',(35.7901485239356,-3.99406008098396,24.0581116296512));
#49341=CARTESIAN_POINT('Ctrl Pts',(35.651237033447,-1.56641747550996,25.4742234354871));
#49342=CARTESIAN_POINT('Ctrl Pts',(35.5123255429583,1.24285843443888,25.5566256704194));
#49343=CARTESIAN_POINT('Ctrl Pts',(35.3734140524697,3.74933117808945,24.2852423089279));
#49344=CARTESIAN_POINT('Ctrl Pts',(35.2345025619811,5.34233757612298,21.9698261730325));
#49345=CARTESIAN_POINT('Ctrl Pts',(35.0955910714924,5.63376634579655,19.1744924650922));
#49346=CARTESIAN_POINT('Ctrl Pts',(34.9566795810039,4.55261539084379,16.5802808547672));
#49347=CARTESIAN_POINT('Ctrl Pts',(34.8177680905151,2.36229036015804,14.8192307343866));
#49348=CARTESIAN_POINT('Ctrl Pts',(34.6788566000265,-0.403570050061598,
14.3203946313223));
#49349=CARTESIAN_POINT('Ctrl Pts',(34.5399451095379,-3.07110688166949,15.2053062193106));
#49350=CARTESIAN_POINT('Ctrl Pts',(34.4010336190492,-4.99041619030151,17.258370525254));
#49351=CARTESIAN_POINT('Ctrl Pts',(34.2621221285606,-5.69388805381733,19.9793902980198));
#49352=CARTESIAN_POINT('Ctrl Pts',(34.123210638072,-5.01013247173753,22.7054313047758));
#49353=CARTESIAN_POINT('Ctrl Pts',(33.9842991475833,-3.10573587859945,24.7723359669663));
#49354=CARTESIAN_POINT('Ctrl Pts',(33.8453876570947,-0.444674944883789,
25.6765350454843));
#49355=CARTESIAN_POINT('Ctrl Pts',(33.7064761666061,2.32472413704993,25.1977344695393));
#49356=CARTESIAN_POINT('Ctrl Pts',(33.5675646761174,4.5277402666191,23.45258656767));
#49357=CARTESIAN_POINT('Ctrl Pts',(33.4286531856288,5.62764275836893,20.8662695385371));
#49358=CARTESIAN_POINT('Ctrl Pts',(33.2897416951401,5.35645744252075,18.0688993822994));
#49359=CARTESIAN_POINT('Ctrl Pts',(33.1508302046515,3.78025441202889,15.7420119176358));
#49360=CARTESIAN_POINT('Ctrl Pts',(33.0119187141629,1.28305106995122,14.4525171581053));
#49361=CARTESIAN_POINT('Ctrl Pts',(32.8730072236743,-1.52674775021,14.5145804867405));
#49362=CARTESIAN_POINT('Ctrl Pts',(32.7340957331856,-3.96457817872488,15.9130811368468));
#49363=CARTESIAN_POINT('Ctrl Pts',(32.595184242697,-5.43650067091328,18.3072961321073));
#49364=CARTESIAN_POINT('Ctrl Pts',(32.4562727522083,-5.58390415826564,21.1139121511696));
#49365=CARTESIAN_POINT('Ctrl Pts',(32.3173612617197,-4.37087606903851,23.6491407643891));
#49366=CARTESIAN_POINT('Ctrl Pts',(32.1784497712311,-2.09295186893649,25.2953128711658));
#49367=CARTESIAN_POINT('Ctrl Pts',(32.0395382807424,0.694887567899583,25.651364189043));
#49368=CARTESIAN_POINT('Ctrl Pts',(31.9006267902538,3.31342843464045,24.630548340935));
#49369=CARTESIAN_POINT('Ctrl Pts',(31.7617152997652,5.12470389326207,22.4815712634547));
#49370=CARTESIAN_POINT('Ctrl Pts',(31.6228038092765,5.68742479231206,19.7279978657925));
#49371=CARTESIAN_POINT('Ctrl Pts',(31.4838923187879,4.86449291911151,17.0406935661994));
#49372=CARTESIAN_POINT('Ctrl Pts',(31.3449808282992,2.85640285127925,15.0743783457899));
#49373=CARTESIAN_POINT('Ctrl Pts',(31.2060693378107,0.15239456490814,14.3081143874981));
#49374=CARTESIAN_POINT('Ctrl Pts',(31.0671578473219,-2.58874229178292,14.9285900110567));
#49375=CARTESIAN_POINT('Ctrl Pts',(30.9282463568333,-4.69917227071445,16.7846359616106));
#49376=CARTESIAN_POINT('Ctrl Pts',(30.7893348663447,-5.66472186494181,19.4240554522615));
#49377=CARTESIAN_POINT('Ctrl Pts',(30.6504233758561,-5.25014990278475,22.2037948923411));
#49378=CARTESIAN_POINT('Ctrl Pts',(30.5115118853674,-3.55646040796889,24.4466139135042));
#49379=CARTESIAN_POINT('Ctrl Pts',(30.3726003948788,-0.996294536997184,
25.606084473567));
#49380=CARTESIAN_POINT('Ctrl Pts',(30.2336889043902,1.80660303374739,25.3997195675029));
#49381=CARTESIAN_POINT('Ctrl Pts',(30.0947774139015,4.16934981683632,23.8777968015442));
#49382=CARTESIAN_POINT('Ctrl Pts',(29.9558659234129,5.51629923237306,21.4111090348162));
#49383=CARTESIAN_POINT('Ctrl Pts',(29.8169544329242,5.51928796218196,18.6006264545402));
#49384=CARTESIAN_POINT('Ctrl Pts',(29.6780429424356,4.17758784863518,16.131079517985));
#49385=CARTESIAN_POINT('Ctrl Pts',(29.539131451947,1.81808329895651,14.6041350047212));
#49386=CARTESIAN_POINT('Ctrl Pts',(29.4002199614583,-0.984369026802969,
14.3918092446592));
#49387=CARTESIAN_POINT('Ctrl Pts',(29.2613084709697,-3.54699511824443,15.5458321135851));
#49388=CARTESIAN_POINT('Ctrl Pts',(29.122396980481,-5.24545090445421,17.7850438518607));
#49389=CARTESIAN_POINT('Ctrl Pts',(28.9834854899925,-5.66593399601205,20.5638952757866));
#49390=CARTESIAN_POINT('Ctrl Pts',(28.8445739995038,-4.70600021426455,23.2053623683698));
#49391=CARTESIAN_POINT('Ctrl Pts',(28.7056625090152,-2.59952252534805,25.0658926725136));
#49392=CARTESIAN_POINT('Ctrl Pts',(28.5667510185265,0.140288477908783,25.6921968581722));
#49393=CARTESIAN_POINT('Ctrl Pts',(28.4278395280379,2.84592037103622,24.9316856318038));
#49394=CARTESIAN_POINT('Ctrl Pts',(28.2889280375492,4.8581879392303,22.9696457493002));
#49395=CARTESIAN_POINT('Ctrl Pts',(28.1500165470606,5.68683342327686,20.2840977738751));
#49396=CARTESIAN_POINT('Ctrl Pts',(28.0111050565719,5.12997021295922,17.5293337855205));
#49397=CARTESIAN_POINT('Ctrl Pts',(27.8721935660834,3.32326938601791,15.3765092714297));
#49398=CARTESIAN_POINT('Ctrl Pts',(27.7332820755947,0.706905555902332,14.3501265090045));
#49399=CARTESIAN_POINT('Ctrl Pts',(27.5943705851061,-2.08168484054595,14.7002477271234));
#49400=CARTESIAN_POINT('Ctrl Pts',(27.4554590946174,-4.36310503684432,16.3415713254618));
#49401=CARTESIAN_POINT('Ctrl Pts',(27.3165476041288,-5.58152241364238,18.8742142853867));
#49402=CARTESIAN_POINT('Ctrl Pts',(27.1776361136402,-5.44008848896973,21.6811374605898));
#49403=CARTESIAN_POINT('Ctrl Pts',(27.0387246231515,-3.97326144328056,24.0784775876005));
#49404=CARTESIAN_POINT('Ctrl Pts',(26.8998131326629,-1.53841091863481,25.4821599552224));
#49405=CARTESIAN_POINT('Ctrl Pts',(26.7609016421743,1.27124954761199,25.5501991420953));
#49406=CARTESIAN_POINT('Ctrl Pts',(26.6219901516856,3.77118979351376,24.2660184564201));
#49407=CARTESIAN_POINT('Ctrl Pts',(26.483078661197,5.35233818143281,21.942488589618));
#49408=CARTESIAN_POINT('Ctrl Pts',(26.3441671707083,5.62947244873437,19.1457015286446));
#49409=CARTESIAN_POINT('Ctrl Pts',(26.2052556802197,4.53507313278025,16.5570510300682));
#49410=CARTESIAN_POINT('Ctrl Pts',(26.066344189731,2.33577363998504,14.8072216076583));
#49411=CARTESIAN_POINT('Ctrl Pts',(25.9274326992424,-0.432600845057991,
14.3225320398901));
#49412=CARTESIAN_POINT('Ctrl Pts',(25.7885212087538,-3.09557884889517,15.2210694167531));
#49413=CARTESIAN_POINT('Ctrl Pts',(25.6496097182651,-5.00436711478803,17.2839190531857));
#49414=CARTESIAN_POINT('Ctrl Pts',(25.5106982277766,-5.69391900935539,20.0084996541662));
#49415=CARTESIAN_POINT('Ctrl Pts',(25.3717867372879,-4.99623591649071,22.7310094463381));
#49416=CARTESIAN_POINT('Ctrl Pts',(25.2328752467993,-3.08129749255576,24.7881511767684));
#49417=CARTESIAN_POINT('Ctrl Pts',(25.0939637563106,-0.415648761477922,
25.6787341931368));
#49418=CARTESIAN_POINT('Ctrl Pts',(24.955052265822,2.35126633876631,25.1857817668509));
#49419=CARTESIAN_POINT('Ctrl Pts',(24.8161407753333,4.54533189117739,23.4293941051249));
#49420=CARTESIAN_POINT('Ctrl Pts',(24.6772292848448,5.6319978794971,20.8374877996482));
#49421=CARTESIAN_POINT('Ctrl Pts',(24.538317794356,5.34651500255474,18.0415405910062));
#49422=CARTESIAN_POINT('Ctrl Pts',(24.3994063038675,3.75843673214303,15.7227416187822));
#49423=CARTESIAN_POINT('Ctrl Pts',(24.2604948133787,1.25467368920259,14.4460302608997));
#49424=CARTESIAN_POINT('Ctrl Pts',(24.1215833228902,-1.55477112346663,14.5224574229995));
#49425=CARTESIAN_POINT('Ctrl Pts',(23.9826718324015,-3.98542008456542,15.9334028133141));
#49426=CARTESIAN_POINT('Ctrl Pts',(23.8437603419129,-5.4450833024811,18.3351114877383));
#49427=CARTESIAN_POINT('Ctrl Pts',(23.7048488514242,-5.57813649059611,21.1424444063059));
#49428=CARTESIAN_POINT('Ctrl Pts',(23.5659373609356,-4.35216330483543,23.6714384779352));
#49429=CARTESIAN_POINT('Ctrl Pts',(23.4270258704469,-2.06585308274432,25.3059435513144));
#49430=CARTESIAN_POINT('Ctrl Pts',(23.2881143799584,0.723770177443836,25.6477378355818));
#49431=CARTESIAN_POINT('Ctrl Pts',(23.1492028894697,3.33705806802798,24.6135484585977));
#49432=CARTESIAN_POINT('Ctrl Pts',(23.0102913989811,5.13732355708965,22.455339609706));
#49433=CARTESIAN_POINT('Ctrl Pts',(22.8713799084924,5.68595990136651,19.6989253759089));
#49434=CARTESIAN_POINT('Ctrl Pts',(22.7324684180038,4.84930037133414,17.0158633010872));
#49435=CARTESIAN_POINT('Ctrl Pts',(22.5935569275151,2.83118407512215,15.0598398141362));
#49436=CARTESIAN_POINT('Ctrl Pts',(22.4546454370266,0.123293723744183,14.3074096768778));
#49437=CARTESIAN_POINT('Ctrl Pts',(22.3157339465378,-2.61463522969817,14.9418908132741));
#49438=CARTESIAN_POINT('Ctrl Pts',(22.1768224560493,-4.71554889295985,16.8087017426564));
#49439=CARTESIAN_POINT('Ctrl Pts',(22.0379109655606,-5.66759226169997,19.4530229581252));
#49440=CARTESIAN_POINT('Ctrl Pts',(21.898999475072,-5.23881474643893,22.2306066398434));
#49441=CARTESIAN_POINT('Ctrl Pts',(21.7600879845833,-3.53368133342206,24.4647376365296));
#49442=CARTESIAN_POINT('Ctrl Pts',(21.6211764940947,-0.967621312193158,
25.611104608311));
#49443=CARTESIAN_POINT('Ctrl Pts',(21.4822650036061,1.83418462264175,25.3904130360561));
#49444=CARTESIAN_POINT('Ctrl Pts',(21.3433535131174,4.1891199437996,23.8564309958406));
#49445=CARTESIAN_POINT('Ctrl Pts',(21.2044420226288,5.52344121283625,21.3828894017822));
#49446=CARTESIAN_POINT('Ctrl Pts',(21.0655305321402,5.51206176346074,18.5724282697484));
#49447=CARTESIAN_POINT('Ctrl Pts',(20.9266190416515,4.1577540218852,16.1097728314767));
#49448=CARTESIAN_POINT('Ctrl Pts',(20.7877075511629,1.79047404821108,14.5949108599485));
#49449=CARTESIAN_POINT('Ctrl Pts',(20.6487960606742,-1.01302713614174,14.3969149613218));
#49450=CARTESIAN_POINT('Ctrl Pts',(20.5098845701856,-3.56971998265816,15.5640237630674));
#49451=CARTESIAN_POINT('Ctrl Pts',(20.3709730796969,-5.25670596345662,17.8118893211313));
#49452=CARTESIAN_POINT('Ctrl Pts',(20.2320615892084,-5.66297712917468,20.5928540829446));
#49453=CARTESIAN_POINT('Ctrl Pts',(20.0931500987197,-4.68955181629675,23.2293791495406));
#49454=CARTESIAN_POINT('Ctrl Pts',(19.9542386082311,-2.57358999310786,25.0791161117457));
#49455=CARTESIAN_POINT('Ctrl Pts',(19.8153271177424,0.169387085457532,25.6914052697466));
#49456=CARTESIAN_POINT('Ctrl Pts',(19.6764156272538,2.8710956298236,24.9170718739538));
#49457=CARTESIAN_POINT('Ctrl Pts',(19.5375041367652,4.87330628821509,22.9447702372957));
#49458=CARTESIAN_POINT('Ctrl Pts',(19.3985926462765,5.68821151139114,20.2550210401063));
#49459=CARTESIAN_POINT('Ctrl Pts',(19.2596811557879,5.11727229042419,17.5031399248504));
#49460=CARTESIAN_POINT('Ctrl Pts',(19.1207696652992,3.2995891045661,15.3595800114377));
#49461=CARTESIAN_POINT('Ctrl Pts',(18.9818581748106,0.678012248551709,14.3465864011172));
#49462=CARTESIAN_POINT('Ctrl Pts',(18.8429466843219,-2.10875176793216,14.710959263679));
#49463=CARTESIAN_POINT('Ctrl Pts',(18.7040351938334,-4.38175114753269,16.3639248068398));
#49464=CARTESIAN_POINT('Ctrl Pts',(18.5651237033447,-5.58720487218263,18.9027636328128));
#49465=CARTESIAN_POINT('Ctrl Pts',(18.4262122128561,-5.43142285253985,21.7089270686976));
#49466=CARTESIAN_POINT('Ctrl Pts',(18.2873007223674,-3.95235895969151,24.0987369497158));
#49467=CARTESIAN_POINT('Ctrl Pts',(18.1483892318788,-1.51036415357132,25.4899531922255));
#49468=CARTESIAN_POINT('Ctrl Pts',(18.0094777413901,1.29960743517518,25.5436275527543));
#49469=CARTESIAN_POINT('Ctrl Pts',(17.8705662509015,3.79294984443393,24.2466831064759));
#49470=CARTESIAN_POINT('Ctrl Pts',(17.7316547604129,5.36219889705587,21.9151002369674));
#49471=CARTESIAN_POINT('Ctrl Pts',(17.5927432699243,5.62503141875362,19.1169329202976));
#49472=CARTESIAN_POINT('Ctrl Pts',(17.4538317794356,4.51741234521826,16.5339111909114));
#49473=CARTESIAN_POINT('Ctrl Pts',(17.314920288947,2.30919587160617,14.795348200333));
#49474=CARTESIAN_POINT('Ctrl Pts',(17.1760087984583,-0.461620333519894,
14.3248178357959));
#49475=CARTESIAN_POINT('Ctrl Pts',(17.0370973079697,-3.11996990950757,15.236957517197));
#49476=CARTESIAN_POINT('Ctrl Pts',(16.8981858174811,-5.01818724422305,17.3095385691044));
#49477=CARTESIAN_POINT('Ctrl Pts',(16.7592743269924,-5.69380114758782,20.0376087881643));
#49478=CARTESIAN_POINT('Ctrl Pts',(16.6203628365038,-4.98220877871081,22.7565162097395));
#49479=CARTESIAN_POINT('Ctrl Pts',(16.4814513460152,-3.05677857315876,24.8038412425784));
#49480=CARTESIAN_POINT('Ctrl Pts',(16.3425398555265,-0.386611714600087,
25.6807849203568));
#49481=CARTESIAN_POINT('Ctrl Pts',(16.2036283650379,2.37774708735693,25.1736935276246));
#49482=CARTESIAN_POINT('Ctrl Pts',(16.0647168745492,4.56280471811248,23.40611201131));
#49483=CARTESIAN_POINT('Ctrl Pts',(15.9258053840606,5.63620580170163,20.8086841720254));
#49484=CARTESIAN_POINT('Ctrl Pts',(15.786893893572,5.33643282509756,18.0142329863651));
#49485=CARTESIAN_POINT('Ctrl Pts',(15.6479824030833,3.73652082106924,15.7035831111337));
#49486=CARTESIAN_POINT('Ctrl Pts',(15.5090709125947,1.22626351607354,14.43968852326));
#49487=CARTESIAN_POINT('Ctrl Pts',(15.3701594221061,-1.58275386094172,14.5304775213102));
#49488=CARTESIAN_POINT('Ctrl Pts',(15.2312479316174,-4.00615782673987,15.9538307751071));
#49489=CARTESIAN_POINT('Ctrl Pts',(15.0923364411288,-5.45352362035877,18.3629703571992));
#49490=CARTESIAN_POINT('Ctrl Pts',(14.9534249506401,-5.57222303173398,21.1709468023069));
#49491=CARTESIAN_POINT('Ctrl Pts',(14.8145134601515,-4.3333367916985,23.6936402340958));
#49492=CARTESIAN_POINT('Ctrl Pts',(14.6756019696629,-2.03870030303929,25.3164355543547));
#49493=CARTESIAN_POINT('Ctrl Pts',(14.5366904791742,0.752633870398657,25.6439638718146));
#49494=CARTESIAN_POINT('Ctrl Pts',(14.3977789886856,3.36060048345727,24.5964279957165));
#49495=CARTESIAN_POINT('Ctrl Pts',(14.258867498197,5.14980895089188,22.4290437827535));
#49496=CARTESIAN_POINT('Ctrl Pts',(14.1199560077083,5.68434640113603,19.6698607549666));
#49497=CARTESIAN_POINT('Ctrl Pts',(13.9810445172197,4.83398108135788,16.991111029916));
#49498=CARTESIAN_POINT('Ctrl Pts',(13.842133026731,2.80589130262175,15.0454303994099));
#49499=CARTESIAN_POINT('Ctrl Pts',(13.7032215362424,0.094189660152942,14.3068537488363));
#49500=CARTESIAN_POINT('Ctrl Pts',(13.5643100457538,-2.64045983103022,14.9553238151557));
#49501=CARTESIAN_POINT('Ctrl Pts',(13.4253985552652,-4.73180226875942,16.8328509320553));
#49502=CARTESIAN_POINT('Ctrl Pts',(13.2864870647765,-5.67031452923321,19.4820047598806));
#49503=CARTESIAN_POINT('Ctrl Pts',(13.1475755742879,-5.22734266747552,22.2573600878037));
#49504=CARTESIAN_POINT('Ctrl Pts',(13.0086640837993,-3.51080990193549,24.4827446683579));
#49505=CARTESIAN_POINT('Ctrl Pts',(12.8697525933106,-0.938922797462035,
25.6159780902017));
#49506=CARTESIAN_POINT('Ctrl Pts',(12.730841102822,1.86171827295241,25.3809656197912));
#49507=CARTESIAN_POINT('Ctrl Pts',(12.5919296123333,4.20878058316006,23.8349643977531));
#49508=CARTESIAN_POINT('Ctrl Pts',(12.4530181218447,5.5304388316326,21.3546336252986));
#49509=CARTESIAN_POINT('Ctrl Pts',(12.3141066313561,5.50469150048808,18.5442673962318));
#49510=CARTESIAN_POINT('Ctrl Pts',(12.1751951408674,4.13781152731789,16.0885678206551));
#49511=CARTESIAN_POINT('Ctrl Pts',(12.0362836503788,1.76281800130937,14.5858279835714));
#49512=CARTESIAN_POINT('Ctrl Pts',(11.8973721598901,-1.04165876881856,14.4021671212367));
#49513=CARTESIAN_POINT('Ctrl Pts',(11.7584606694015,-3.59235154821945,15.5823313520337));
#49514=CARTESIAN_POINT('Ctrl Pts',(11.6195491789129,-5.26782363223333,17.8387919792617));
#49515=CARTESIAN_POINT('Ctrl Pts',(11.4806376884243,-5.65987225373433,20.6217973951602));
#49516=CARTESIAN_POINT('Ctrl Pts',(11.3417261979356,-4.67298085134745,23.2533115270689));
#49517=CARTESIAN_POINT('Ctrl Pts',(11.202814707447,-2.5475901970503,25.0922068022728));
#49518=CARTESIAN_POINT('Ctrl Pts',(11.0639032169583,0.198481265874501,25.690464929715));
#49519=CARTESIAN_POINT('Ctrl Pts',(10.9249917264697,2.89619584913197,24.9023296026165));
#49520=CARTESIAN_POINT('Ctrl Pts',(10.7860802359811,4.888297267578,22.9198177602393));
#49521=CARTESIAN_POINT('Ctrl Pts',(10.6471687454924,5.68944093137202,20.2259376410611));
#49522=CARTESIAN_POINT('Ctrl Pts',(10.5082572550038,5.10444062192735,17.4770113225705));
#49523=CARTESIAN_POINT('Ctrl Pts',(10.3693457645152,3.27582258445175,15.3427720343089));
#49524=CARTESIAN_POINT('Ctrl Pts',(10.2304342740265,0.649101220549331,14.3431940518787));
#49525=CARTESIAN_POINT('Ctrl Pts',(10.0915227835379,-2.13576358059751,14.7218090355679));
#49526=CARTESIAN_POINT('Ctrl Pts',(9.95261129304924,-4.40028273597386,16.3863733213419));
#49527=CARTESIAN_POINT('Ctrl Pts',(9.8136998025606,-5.5927413025174,18.9313416578085));
#49528=CARTESIAN_POINT('Ctrl Pts',(9.67478831207196,-5.42261525945185,21.7366720119756));
#49529=CARTESIAN_POINT('Ctrl Pts',(9.53587682158334,-3.93135317652793,24.1188891864947));
#49530=CARTESIAN_POINT('Ctrl Pts',(9.3969653310947,-1.48227791335496,25.4976029428106));
#49531=CARTESIAN_POINT('Ctrl Pts',(9.25805384060606,1.3279313559613,25.5369110741526));
#49532=CARTESIAN_POINT('Ctrl Pts',(9.11914235011741,3.81461076212522,24.2272367644477));
#49533=CARTESIAN_POINT('Ctrl Pts',(8.98023085962878,5.37191946527065,21.8876618309077));
#49534=CARTESIAN_POINT('Ctrl Pts',(8.84131936914014,5.62044337192589,19.0881873919529));
#49535=CARTESIAN_POINT('Ctrl Pts',(8.70240787865151,4.49963348974343,16.5108619420839));
#49536=CARTESIAN_POINT('Ctrl Pts',(8.56349638816287,2.282557749663,14.7836108227364));
#49537=CARTESIAN_POINT('Ctrl Pts',(8.42458489767425,-0.490627756988433,
14.3272519592977));
#49538=CARTESIAN_POINT('Ctrl Pts',(8.2856734071856,-3.14427942601743,15.2529701053877));
#49539=CARTESIAN_POINT('Ctrl Pts',(8.14676191669697,-5.03187621740111,17.3352284034138));
#49540=CARTESIAN_POINT('Ctrl Pts',(8.00785042620833,-5.6935344715951,20.0667169392121));
#49541=CARTESIAN_POINT('Ctrl Pts',(7.8689389357197,-4.96805142501369,22.7819509283305));
#49542=CARTESIAN_POINT('Ctrl Pts',(7.73002744523106,-3.03217976123968,24.8194057543175));
#49543=CARTESIAN_POINT('Ctrl Pts',(7.59111595474241,-0.357564563168171,
25.6826871735461));
#49544=CARTESIAN_POINT('Ctrl Pts',(7.45220446425379,2.404165690716,25.1614700678008));
#49545=CARTESIAN_POINT('Ctrl Pts',(7.31329297376515,4.58015829075132,23.3827408947304));
#49546=CARTESIAN_POINT('Ctrl Pts',(7.17438148327652,5.64026641500344,20.7798594084857));
#49547=CARTESIAN_POINT('Ctrl Pts',(7.03546999278788,5.32621117365894,17.9869772820929));
#49548=CARTESIAN_POINT('Ctrl Pts',(6.89655850229923,3.71450725160592,15.6845368954205));
#49549=CARTESIAN_POINT('Ctrl Pts',(6.7576470118106,1.19782129309763,14.4334921109351));
#49550=CARTESIAN_POINT('Ctrl Pts',(6.61873552132196,-1.61069523127324,14.5386405720578));
#49551=CARTESIAN_POINT('Ctrl Pts',(6.47982403083333,-4.02679086324272,15.9743644883169));
#49552=CARTESIAN_POINT('Ctrl Pts',(6.34091254034469,-5.46182140394848,18.3908720123652));
#49553=CARTESIAN_POINT('Ctrl Pts',(6.20200104985606,-5.56616393623456,21.1994185942286));
#49554=CARTESIAN_POINT('Ctrl Pts',(6.06308955936741,-4.31439702168094,23.7157454526016));
#49555=CARTESIAN_POINT('Ctrl Pts',(5.92417806887878,-2.01149423949129,25.3267886060659));
#49556=CARTESIAN_POINT('Ctrl Pts',(5.78526657839015,0.781477892377476,25.6400423963783));
#49557=CARTESIAN_POINT('Ctrl Pts',(5.6463550879015,3.38405506561942,24.579187399755));
#49558=CARTESIAN_POINT('Ctrl Pts',(5.50744359741287,5.16215974834815,22.4026844698698));
#49559=CARTESIAN_POINT('Ctrl Pts',(5.36853210692423,5.68258433379142,19.640804762604));
#49560=CARTESIAN_POINT('Ctrl Pts',(5.22962061643561,4.81853544957058,16.9664373996156));
#49561=CARTESIAN_POINT('Ctrl Pts',(5.09070912594697,2.78052519483453,15.0311504782184));
#49562=CARTESIAN_POINT('Ctrl Pts',(4.95179763545833,0.0650831348035412,
14.3064466179034));
#49563=CARTESIAN_POINT('Ctrl Pts',(4.81288614496969,-2.66621542082262,14.968888665614));
#49564=CARTESIAN_POINT('Ctrl Pts',(4.67397465448106,-4.74793197331199,16.85708289864));
#49565=CARTESIAN_POINT('Ctrl Pts',(4.53506316399242,-5.67288859639181,19.5110001000541));
#49566=CARTESIAN_POINT('Ctrl Pts',(4.39615167350378,-5.21573396573087,22.2840545369891));
#49567=CARTESIAN_POINT('Ctrl Pts',(4.25724018301514,-3.48784671128103,24.5006345383542));
#49568=CARTESIAN_POINT('Ctrl Pts',(4.11832869252652,-0.910199742873642,
25.6207047918644));
#49569=CARTESIAN_POINT('Ctrl Pts',(3.97941720203787,1.88920326505482,25.3713775656284));
#49570=CARTESIAN_POINT('Ctrl Pts',(3.84050571154924,4.22833122106338,23.8133975683351));
#49571=CARTESIAN_POINT('Ctrl Pts',(3.70159422106059,5.5372919058718,21.3263424438669));
#49572=CARTESIAN_POINT('Ctrl Pts',(3.56268273057196,5.4971773658931,18.5161445700008));
#49573=CARTESIAN_POINT('Ctrl Pts',(3.42377124008332,4.11776088615646,16.0674650397519));
#49574=CARTESIAN_POINT('Ctrl Pts',(3.28485974959469,1.73511588106992,14.5768866129545));
#49575=CARTESIAN_POINT('Ctrl Pts',(3.14594825910605,-1.07026317650166,14.4075655871855));
#49576=CARTESIAN_POINT('Ctrl Pts',(3.00703676861742,-3.6148892234453,15.6007544018894));
#49577=CARTESIAN_POINT('Ctrl Pts',(2.86812527812878,-5.27880362017199,17.8657511233237));
#49578=CARTESIAN_POINT('Ctrl Pts',(2.72921378764014,-5.65661945091725,20.6507244555628));
#49579=CARTESIAN_POINT('Ctrl Pts',(2.59030229715152,-4.65628775236742,23.277158876247));
#49580=CARTESIAN_POINT('Ctrl Pts',(2.45139080666287,-2.521523817008,25.1051644003928));
#49581=CARTESIAN_POINT('Ctrl Pts',(2.31247931617424,0.227570259334219,25.6893758657282));
#49582=CARTESIAN_POINT('Ctrl Pts',(2.1735678256856,2.92122037178518,24.8874591970467));
#49583=CARTESIAN_POINT('Ctrl Pts',(2.03465633519697,4.9031604877807,22.8947889822085));
#49584=CARTESIAN_POINT('Ctrl Pts',(1.89574484470833,5.69052164662065,20.1968483134104));
#49585=CARTESIAN_POINT('Ctrl Pts',(1.7568333542197,5.09147555163317,17.4509487077672));
#49586=CARTESIAN_POINT('Ctrl Pts',(1.61792186373106,3.25197042952828,15.3260856884126));
#49587=CARTESIAN_POINT('Ctrl Pts',(1.47901037324242,0.620173261604023,14.3399497289677));
#49588=CARTESIAN_POINT('Ctrl Pts',(1.34009888275378,-2.16271963966253,14.7327964067747));
#49589=CARTESIAN_POINT('Ctrl Pts',(1.20118739226515,-4.41869918570553,16.4089169761365));
#49590=CARTESIAN_POINT('Ctrl Pts',(1.06227590177651,-5.5981318200567,18.9599462473385));
#49591=CARTESIAN_POINT('Ctrl Pts',(0.923364411287872,-5.41366542779912,
21.7643742548674));
#49592=CARTESIAN_POINT('Ctrl Pts',(0.784452920799232,-3.91024565102259,
24.138928475994));
#49593=CARTESIAN_POINT('Ctrl Pts',(0.645541430310592,-1.45415094708632,
25.5051194323653));
#49594=CARTESIAN_POINT('Ctrl Pts',(0.506629939821954,1.35621666180418,25.5300293552048));
#49595=CARTESIAN_POINT('Ctrl Pts',(0.367718449333321,3.83617967324551,24.207720366993));
#49596=CARTESIAN_POINT('Ctrl Pts',(0.228806958844687,5.38148449802081,21.8600943129511));
#49597=CARTESIAN_POINT('Ctrl Pts',(0.0898954683560495,5.61573809242548,
19.0596248185465));
#49598=CARTESIAN_POINT('Ctrl Pts',(-0.0490160221325763,4.48168004880515,
16.4875673042026));
#49599=CARTESIAN_POINT('Ctrl Pts',(-0.141623682458336,2.99785669531383,
15.3445018393813));
#49600=CARTESIAN_POINT('Ctrl Pts',(-0.187927512621213,2.16407317598292,
14.9847270910257));
#49601=CARTESIAN_POINT('Ctrl Pts',(50.5637825378637,-1.32667918156829,15.0375285480223));
#49602=CARTESIAN_POINT('Ctrl Pts',(50.5174787077008,-2.15168451764989,15.2580874801298));
#49603=CARTESIAN_POINT('Ctrl Pts',(50.4248710473751,-3.68873492200737,16.1183991355923));
#49604=CARTESIAN_POINT('Ctrl Pts',(50.2859595568864,-5.09604146002229,18.3561196065066));
#49605=CARTESIAN_POINT('Ctrl Pts',(50.1470480663978,-5.26156574360687,20.9937156315332));
#49606=CARTESIAN_POINT('Ctrl Pts',(50.0081365759091,-4.14529719998611,23.3895155338352));
#49607=CARTESIAN_POINT('Ctrl Pts',(49.8692250854205,-2.01903759094086,24.9593576609462));
#49608=CARTESIAN_POINT('Ctrl Pts',(49.7303135949318,0.599101898234613,25.321007862679));
#49609=CARTESIAN_POINT('Ctrl Pts',(49.5914021044432,3.07129336959566,24.3862371798792));
#49610=CARTESIAN_POINT('Ctrl Pts',(49.4524906139546,4.79520484297246,22.3828481604625));
#49611=CARTESIAN_POINT('Ctrl Pts',(49.3135791234659,5.35084266186257,19.7989048767012));
#49612=CARTESIAN_POINT('Ctrl Pts',(49.1746676329773,4.60282890398964,17.2639605279354));
#49613=CARTESIAN_POINT('Ctrl Pts',(49.0357561424887,2.73340824983943,15.3956070723818));
#49614=CARTESIAN_POINT('Ctrl Pts',(48.8968446520001,0.19803463412749,14.6490438348891));
#49615=CARTESIAN_POINT('Ctrl Pts',(48.7579331615113,-2.38558680835433,15.2061573259097));
#49616=CARTESIAN_POINT('Ctrl Pts',(48.6190216710228,-4.38799717418834,16.9312165240447));
#49617=CARTESIAN_POINT('Ctrl Pts',(48.4801101805341,-5.32134007622315,19.4039370066215));
#49618=CARTESIAN_POINT('Ctrl Pts',(48.3411986900456,-4.95822109602027,22.021879075434));
#49619=CARTESIAN_POINT('Ctrl Pts',(48.2022871995568,-3.38710848985947,24.1472216448687));
#49620=CARTESIAN_POINT('Ctrl Pts',(48.0633757090683,-0.990779481809887,
25.262158055552));
#49621=CARTESIAN_POINT('Ctrl Pts',(47.9244642185795,1.64693757250601,25.0950513217741));
#49622=CARTESIAN_POINT('Ctrl Pts',(47.785552728091,3.88340384844544,23.6866144231869));
#49623=CARTESIAN_POINT('Ctrl Pts',(47.6466412376023,5.17373905472326,21.3799911398092));
#49624=CARTESIAN_POINT('Ctrl Pts',(47.5077297471137,5.20357304491207,18.7371544365421));
#49625=CARTESIAN_POINT('Ctrl Pts',(47.368818256625,3.96563723118361,16.4019904525415));
#49626=CARTESIAN_POINT('Ctrl Pts',(47.2299067661365,1.76153545929722,14.9434256480188));
#49627=CARTESIAN_POINT('Ctrl Pts',(47.0909952756476,-0.871737085184379,
14.7168166976175));
#49628=CARTESIAN_POINT('Ctrl Pts',(46.9520837851592,-3.29262441972186,15.7773733550559));
#49629=CARTESIAN_POINT('Ctrl Pts',(46.8131722946704,-4.91131492144359,17.8667074522167));
#49630=CARTESIAN_POINT('Ctrl Pts',(46.6742608041819,-5.33343977443084,20.4757851663839));
#49631=CARTESIAN_POINT('Ctrl Pts',(46.5353493136931,-4.45615481032689,22.9689452097341));
#49632=CARTESIAN_POINT('Ctrl Pts',(46.3964378232046,-2.49319689370494,24.7387678357613));
#49633=CARTESIAN_POINT('Ctrl Pts',(46.2575263327159,0.0771897474612934,
25.354063232247));
#49634=CARTESIAN_POINT('Ctrl Pts',(46.1186148422274,2.62877030477265,24.6649242262618));
#49635=CARTESIAN_POINT('Ctrl Pts',(45.9797033517386,4.5398917802619,22.8392488400151));
#49636=CARTESIAN_POINT('Ctrl Pts',(45.8407918612501,5.34493909024452,20.3218345438155));
#49637=CARTESIAN_POINT('Ctrl Pts',(45.7018803707613,4.84777495333142,17.7260102564282));
#49638=CARTESIAN_POINT('Ctrl Pts',(45.5629688802728,3.16952569465798,15.6842082739178));
#49639=CARTESIAN_POINT('Ctrl Pts',(45.4240573897841,0.71907069684952,14.6938819571226));
#49640=CARTESIAN_POINT('Ctrl Pts',(45.2851458992955,-1.90657471505998,14.9963089416001));
#49641=CARTESIAN_POINT('Ctrl Pts',(45.1462344088068,-4.06771279089063,16.5178075867578));
#49642=CARTESIAN_POINT('Ctrl Pts',(45.0073229183182,-5.23781578296322,18.8876883639203));
#49643=CARTESIAN_POINT('Ctrl Pts',(44.8684114278295,-5.13180625922525,21.5285666062667));
#49644=CARTESIAN_POINT('Ctrl Pts',(44.7294999373409,-3.77551179468938,23.7970333209202));
#49645=CARTESIAN_POINT('Ctrl Pts',(44.5905884468524,-1.49937248366909,25.1404118032734));
#49646=CARTESIAN_POINT('Ctrl Pts',(44.4516769563636,1.14206566021501,25.231408737594));
#49647=CARTESIAN_POINT('Ctrl Pts',(44.312765465875,3.50525723276716,24.0478541332601));
#49648=CARTESIAN_POINT('Ctrl Pts',(44.1738539753864,5.01444728804201,21.87810269886));
#49649=CARTESIAN_POINT('Ctrl Pts',(44.0349424848978,5.3019450942392,19.2507806931946));
#49650=CARTESIAN_POINT('Ctrl Pts',(43.8960309944091,4.29770627332817,16.805994342489));
#49651=CARTESIAN_POINT('Ctrl Pts',(43.7571195039205,2.24639802654879,15.1393778938973));
#49652=CARTESIAN_POINT('Ctrl Pts',(43.6182080134318,-0.35221023152451,14.6569765764292));
#49653=CARTESIAN_POINT('Ctrl Pts',(43.4792965229433,-2.86500793358189,15.4763199834063));
#49654=CARTESIAN_POINT('Ctrl Pts',(43.3403850324545,-4.67979092236272,17.3977878113058));
#49655=CARTESIAN_POINT('Ctrl Pts',(43.201473541966,-5.35441549113415,19.953244248272));
#49656=CARTESIAN_POINT('Ctrl Pts',(43.0625620514773,-4.7245198350227,22.5200919984187));
#49657=CARTESIAN_POINT('Ctrl Pts',(42.9236505609887,-2.94356825360016,24.4729584492162));
#49658=CARTESIAN_POINT('Ctrl Pts',(42.7847390705,-0.445461956316902,25.3360580016986));
#49659=CARTESIAN_POINT('Ctrl Pts',(42.6458275800114,2.16117423230435,24.89910984666));
#49660=CARTESIAN_POINT('Ctrl Pts',(42.5069160895227,4.2412738642828,23.2685696199054));
#49661=CARTESIAN_POINT('Ctrl Pts',(42.3680045990342,5.28805295093088,20.8416931389576));
#49662=CARTESIAN_POINT('Ctrl Pts',(42.2290931085454,5.04648001555839,18.2097511891956));
#49663=CARTESIAN_POINT('Ctrl Pts',(42.0901816180569,3.5754105542507,16.0139755745141));
#49664=CARTESIAN_POINT('Ctrl Pts',(41.9512701275682,1.23324780778372,14.7893329413007));
#49665=CARTESIAN_POINT('Ctrl Pts',(41.8123586370796,-1.40937662497005,14.8341884586248));
#49666=CARTESIAN_POINT('Ctrl Pts',(41.6734471465909,-3.70862831894497,16.1376137759235));
#49667=CARTESIAN_POINT('Ctrl Pts',(41.5345356561023,-5.10433028715659,18.3820495459895));
#49668=CARTESIAN_POINT('Ctrl Pts',(41.3956241656136,-5.25644140869157,21.0206738308635));
#49669=CARTESIAN_POINT('Ctrl Pts',(41.2567126751251,-4.12790216980831,23.4106267794218));
#49670=CARTESIAN_POINT('Ctrl Pts',(41.1178011846363,-1.99366363923406,24.9696334518365));
#49671=CARTESIAN_POINT('Ctrl Pts',(40.9788896941478,0.626300092027496,25.3178660707791));
#49672=CARTESIAN_POINT('Ctrl Pts',(40.8399782036591,3.09367552709713,24.3704831637998));
#49673=CARTESIAN_POINT('Ctrl Pts',(40.7010667131705,4.8073249390358,22.3582998712084));
#49674=CARTESIAN_POINT('Ctrl Pts',(40.5621552226818,5.34974424734503,19.7715534197766));
#49675=CARTESIAN_POINT('Ctrl Pts',(40.4232437321932,4.58878140681505,17.2404644317412));
#49676=CARTESIAN_POINT('Ctrl Pts',(40.2843322417046,2.70983320211814,15.3816934522798));
#49677=CARTESIAN_POINT('Ctrl Pts',(40.1454207512159,0.170676198893053,14.6481011792871));
#49678=CARTESIAN_POINT('Ctrl Pts',(40.0065092607273,-2.4100634110107,15.218415983492));
#49679=CARTESIAN_POINT('Ctrl Pts',(39.8675977702387,-4.40362847905842,16.9536895150949));
#49680=CARTESIAN_POINT('Ctrl Pts',(39.72868627975,-5.32431781990231,19.4311493124838));
#49681=CARTESIAN_POINT('Ctrl Pts',(39.5897747892614,-4.9478197662925,22.0472007503668));
#49682=CARTESIAN_POINT('Ctrl Pts',(39.4508632987728,-3.36586222510812,24.1644835014209));
#49683=CARTESIAN_POINT('Ctrl Pts',(39.3119518082841,-0.963864596617645,
25.2671544871405));
#49684=CARTESIAN_POINT('Ctrl Pts',(39.1730403177955,1.67296368003944,25.0865650371627));
#49685=CARTESIAN_POINT('Ctrl Pts',(39.0341288273068,3.90220032326434,23.6667129679227));
#49686=CARTESIAN_POINT('Ctrl Pts',(38.8952173368182,5.18072642643651,21.3535231975993));
#49687=CARTESIAN_POINT('Ctrl Pts',(38.7563058463296,5.19704894939304,18.7105685091368));
#49688=CARTESIAN_POINT('Ctrl Pts',(38.617394355841,3.94719116276856,16.3817637892781));
#49689=CARTESIAN_POINT('Ctrl Pts',(38.4784828653523,1.73566151637966,14.9344861610518));
#49690=CARTESIAN_POINT('Ctrl Pts',(38.3395713748637,-0.898735118089893,
14.7213423543926));
#49691=CARTESIAN_POINT('Ctrl Pts',(38.200659884375,-3.3141688909171,15.7942615494429));
#49692=CARTESIAN_POINT('Ctrl Pts',(38.0617483938864,-4.92215685494637,17.8918436378386));
#49693=CARTESIAN_POINT('Ctrl Pts',(37.9228369033977,-5.33093770141904,20.5030453017433));
#49694=CARTESIAN_POINT('Ctrl Pts',(37.7839254129091,-4.44091832205815,22.9916877859873));
#49695=CARTESIAN_POINT('Ctrl Pts',(37.6450139224205,-2.46893812404761,24.7514519772004));
#49696=CARTESIAN_POINT('Ctrl Pts',(37.5061024319319,0.104560525815868,25.353598644693));
#49697=CARTESIAN_POINT('Ctrl Pts',(37.3671909414432,2.65258462651949,24.6514240992592));
#49698=CARTESIAN_POINT('Ctrl Pts',(37.2282794509546,4.55434765554542,22.8160022699645));
#49699=CARTESIAN_POINT('Ctrl Pts',(37.0893679604659,5.34651456943153,20.2945051966832));
#49700=CARTESIAN_POINT('Ctrl Pts',(36.9504564699773,4.83608619537201,17.701256503446));
#49701=CARTESIAN_POINT('Ctrl Pts',(36.8115449794886,3.1474204839998,15.6680609827797));
#49702=CARTESIAN_POINT('Ctrl Pts',(36.6726334890001,0.691934624959393,14.6902751646814));
#49703=CARTESIAN_POINT('Ctrl Pts',(36.5337219985113,-1.93213036546348,15.0061213868506));
#49704=CARTESIAN_POINT('Ctrl Pts',(36.3948105080228,-4.08546178225335,16.5386486197203));
#49705=CARTESIAN_POINT('Ctrl Pts',(36.2558990175341,-5.24343384903385,18.9144803904014));
#49706=CARTESIAN_POINT('Ctrl Pts',(36.1169875270455,-5.1239246454075,21.5547821648715));
#49707=CARTESIAN_POINT('Ctrl Pts',(35.9780760365568,-3.75605073385406,23.8162853977043));
#49708=CARTESIAN_POINT('Ctrl Pts',(35.8391645460682,-1.47307336122034,25.148009928553));
#49709=CARTESIAN_POINT('Ctrl Pts',(35.7002530555796,1.16879547129917,25.2255017460802));
#49710=CARTESIAN_POINT('Ctrl Pts',(35.5613415650909,3.52590542890769,24.0298811717489));
#49711=CARTESIAN_POINT('Ctrl Pts',(35.4224300746023,5.02398325674396,21.8524426004531));
#49712=CARTESIAN_POINT('Ctrl Pts',(35.2835185841136,5.29804554474264,19.2236851425809));
#49713=CARTESIAN_POINT('Ctrl Pts',(35.1446070936251,4.28132127034039,16.784064750007));
#49714=CARTESIAN_POINT('Ctrl Pts',(35.0056956031363,2.2215195217249,15.127957064371));
#49715=CARTESIAN_POINT('Ctrl Pts',(34.8667841126478,-0.379520976640382,
14.6588470177024));
#49716=CARTESIAN_POINT('Ctrl Pts',(34.7278726221591,-2.88809707985093,15.491025991495));
#49717=CARTESIAN_POINT('Ctrl Pts',(34.5889611316705,-4.69303315767885,17.4217464956014));
#49718=CARTESIAN_POINT('Ctrl Pts',(34.4500496411818,-5.35458455040435,19.9806184472246));
#49719=CARTESIAN_POINT('Ctrl Pts',(34.3111381506932,-4.7115745295799,22.5442124133474));
#49720=CARTESIAN_POINT('Ctrl Pts',(34.1722266602045,-2.92066250618256,24.4879485154128));
#49721=CARTESIAN_POINT('Ctrl Pts',(34.0333151697159,-0.418176396747093,
25.3382656222055));
#49722=CARTESIAN_POINT('Ctrl Pts',(33.8944036792273,2.18619190095496,24.8879971690065));
#49723=CARTESIAN_POINT('Ctrl Pts',(33.7554921887387,4.25792847536376,23.2468440755145));
#49724=CARTESIAN_POINT('Ctrl Pts',(33.61658069825,5.29228686695988,20.814647819503));
#49725=CARTESIAN_POINT('Ctrl Pts',(33.4776692077614,5.03726170861247,18.1839752669736));
#49726=CARTESIAN_POINT('Ctrl Pts',(33.3387577172727,3.55498592173361,15.9957489528886));
#49727=CARTESIAN_POINT('Ctrl Pts',(33.1998462267842,1.20659299438363,14.7830962537228));
#49728=CARTESIAN_POINT('Ctrl Pts',(33.0609347362954,-1.43576758769577,14.841461177219));
#49729=CARTESIAN_POINT('Ctrl Pts',(32.9220232458069,-3.7283256825603,16.156624015689));
#49730=CARTESIAN_POINT('Ctrl Pts',(32.7831117553182,-5.11253509475286,18.4081657570785));
#49731=CARTESIAN_POINT('Ctrl Pts',(32.6442002648296,-5.25115468625036,21.0475332038116));
#49732=CARTESIAN_POINT('Ctrl Pts',(32.5052887743409,-4.11041194519357,23.4316854449129));
#49733=CARTESIAN_POINT('Ctrl Pts',(32.3663772838523,-1.96823113419552,24.9797607928896));
#49734=CARTESIAN_POINT('Ctrl Pts',(32.2274657933636,0.65347864239245,25.3145947179398));
#49735=CARTESIAN_POINT('Ctrl Pts',(32.0885543028751,3.11597849084889,24.3546101314106));
#49736=CARTESIAN_POINT('Ctrl Pts',(31.9496428123863,4.81931854523574,22.3336923772348));
#49737=CARTESIAN_POINT('Ctrl Pts',(31.8107313218978,5.34850644000348,19.7442066981756));
#49738=CARTESIAN_POINT('Ctrl Pts',(31.6718198314091,4.57461375847793,17.2170410867637));
#49739=CARTESIAN_POINT('Ctrl Pts',(31.5329083409205,2.68618744039703,15.3679002183599));
#49740=CARTESIAN_POINT('Ctrl Pts',(31.3939968504318,0.143313246609341,14.6472985637752));
#49741=CARTESIAN_POINT('Ctrl Pts',(31.2550853599433,-2.43447699525212,15.2307995311997));
#49742=CARTESIAN_POINT('Ctrl Pts',(31.1161738694545,-4.41914470439699,16.9762421668366));
#49743=CARTESIAN_POINT('Ctrl Pts',(30.977262378966,-5.32715639887223,19.4583764647177));
#49744=CARTESIAN_POINT('Ctrl Pts',(30.8383508884772,-4.93728912318725,22.0724689300624));
#49745=CARTESIAN_POINT('Ctrl Pts',(30.6994393979887,-3.34452798766702,24.1816365088));
#49746=CARTESIAN_POINT('Ctrl Pts',(30.5605279075,-0.93692452064997,25.2720132581986));
#49747=CARTESIAN_POINT('Ctrl Pts',(30.4216164170114,1.69894606317944,25.0779458077478));
#49748=CARTESIAN_POINT('Ctrl Pts',(30.2827049265227,3.92089480921487,23.646715679497));
#49749=CARTESIAN_POINT('Ctrl Pts',(30.1437934360341,5.18757839386559,21.327019879096));
#49750=CARTESIAN_POINT('Ctrl Pts',(30.0048819455454,5.19038902279063,18.6840162827332));
#49751=CARTESIAN_POINT('Ctrl Pts',(29.8659704550569,3.92864192987812,16.3616316928023));
#49752=CARTESIAN_POINT('Ctrl Pts',(29.7270589645682,1.7097422098796,14.925679067326));
#49753=CARTESIAN_POINT('Ctrl Pts',(29.5881474740796,-0.925709661482013,
14.7260059751024));
#49754=CARTESIAN_POINT('Ctrl Pts',(29.4492359835909,-3.33562674239409,15.8112596657894));
#49755=CARTESIAN_POINT('Ctrl Pts',(29.3103244931023,-4.93287014205778,17.9170349226135));
#49756=CARTESIAN_POINT('Ctrl Pts',(29.1714130026136,-5.3282962980484,20.5302922894222));
#49757=CARTESIAN_POINT('Ctrl Pts',(29.0325015121251,-4.4255657651377,23.0143521709412));
#49758=CARTESIAN_POINT('Ctrl Pts',(28.8935900216363,-2.44461482577355,24.7640119338248));
#49759=CARTESIAN_POINT('Ctrl Pts',(28.7546785311478,0.13192857135758,25.352994134508));
#49760=CARTESIAN_POINT('Ctrl Pts',(28.6157670406591,2.67632961983071,24.6378024017883));
#49761=CARTESIAN_POINT('Ctrl Pts',(28.4768555501705,4.56868449756808,22.7926821003648));
#49762=CARTESIAN_POINT('Ctrl Pts',(28.3379440596818,5.3479503111387,20.2671681523096));
#49763=CARTESIAN_POINT('Ctrl Pts',(28.1990325691932,4.82427104058186,17.676562830843));
#49764=CARTESIAN_POINT('Ctrl Pts',(28.0601210787045,3.12523301178589,15.6520269119898));
#49765=CARTESIAN_POINT('Ctrl Pts',(27.9212095882159,0.664780468539763,14.6868071481768));
#49766=CARTESIAN_POINT('Ctrl Pts',(27.7822980977273,-1.95763551735538,15.0160643530232));
#49767=CARTESIAN_POINT('Ctrl Pts',(27.6433866072387,-4.10310399524189,16.5595801191937));
#49768=CARTESIAN_POINT('Ctrl Pts',(27.50447511675,-5.24891487176117,18.941300788221));
#49769=CARTESIAN_POINT('Ctrl Pts',(27.3655636262614,-5.11590911176077,21.5809570874062));
#49770=CARTESIAN_POINT('Ctrl Pts',(27.2266521357728,-3.73649150419176,23.8354377313574));
#49771=CARTESIAN_POINT('Ctrl Pts',(27.0877406452841,-1.44673573825756,25.1554735045062));
#49772=CARTESIAN_POINT('Ctrl Pts',(26.9488291547955,1.19549473453172,25.2194581798999));
#49773=CARTESIAN_POINT('Ctrl Pts',(26.8099176643069,3.5464614713409,24.0118028845286));
#49774=CARTESIAN_POINT('Ctrl Pts',(26.6710061738182,5.03338791770333,21.8267340862685));
#49775=CARTESIAN_POINT('Ctrl Pts',(26.5320946833296,5.29400752456154,19.1966098818738));
#49776=CARTESIAN_POINT('Ctrl Pts',(26.3931831928409,4.26482436995908,16.762219209795));
#49777=CARTESIAN_POINT('Ctrl Pts',(26.2542717023523,2.19658295486167,15.1166635714475));
#49778=CARTESIAN_POINT('Ctrl Pts',(26.1153602118636,-0.40682180252673,14.6608570563239));
#49779=CARTESIAN_POINT('Ctrl Pts',(25.976448721375,-2.91111074228793,15.5058498469507));
#49780=CARTESIAN_POINT('Ctrl Pts',(25.8375372308863,-4.70615273502447,17.4457725656006));
#49781=CARTESIAN_POINT('Ctrl Pts',(25.6986257403978,-5.35461366127627,20.0079931527372));
#49782=CARTESIAN_POINT('Ctrl Pts',(25.5597142499091,-4.69850608156596,22.5682663322764));
#49783=CARTESIAN_POINT('Ctrl Pts',(25.4208027594205,-2.89768042379711,24.5028212837687));
#49784=CARTESIAN_POINT('Ctrl Pts',(25.2818912689318,-0.39087990764277,25.3403337208285));
#49785=CARTESIAN_POINT('Ctrl Pts',(25.1429797784432,2.2111524308953,24.8767567377677));
#49786=CARTESIAN_POINT('Ctrl Pts',(25.0040682879546,4.27447180044954,23.2250336710147));
#49787=CARTESIAN_POINT('Ctrl Pts',(24.8651567974659,5.29638246281417,20.7875812082645));
#49788=CARTESIAN_POINT('Ctrl Pts',(24.7262453069773,5.02791174687594,18.1582468087054));
#49789=CARTESIAN_POINT('Ctrl Pts',(24.5873338164886,3.53446837545621,15.9776269870987));
#49790=CARTESIAN_POINT('Ctrl Pts',(24.448422326,1.17990664524902,14.7769959160925));
#49791=CARTESIAN_POINT('Ctrl Pts',(24.3095108355114,-1.46212102493793,14.8488687203245));
#49792=CARTESIAN_POINT('Ctrl Pts',(24.1705993450227,-3.74792560197564,16.1757347066302));
#49793=CARTESIAN_POINT('Ctrl Pts',(24.0316878545341,-5.12060628019952,18.4343235726376));
#49794=CARTESIAN_POINT('Ctrl Pts',(23.8927763640455,-5.24573071867263,21.074365198241));
#49795=CARTESIAN_POINT('Ctrl Pts',(23.7538648735568,-4.09281429010269,23.4526544192474));
#49796=CARTESIAN_POINT('Ctrl Pts',(23.6149533830683,-1.94274718710914,24.9897579820064));
#49797=CARTESIAN_POINT('Ctrl Pts',(23.4760418925795,0.680640113320448,25.3111844618838));
#49798=CARTESIAN_POINT('Ctrl Pts',(23.337130402091,3.13820001481857,24.3386232861369));
#49799=CARTESIAN_POINT('Ctrl Pts',(23.1982189116023,4.83118619284732,22.3090238894517));
#49800=CARTESIAN_POINT('Ctrl Pts',(23.0593074211137,5.34712884312223,19.7168666620349));
#49801=CARTESIAN_POINT('Ctrl Pts',(22.920395930625,4.56032654720136,17.1936904777079));
#49802=CARTESIAN_POINT('Ctrl Pts',(22.7814844401364,2.66247147199116,15.3542280498446));
#49803=CARTESIAN_POINT('Ctrl Pts',(22.6425729496478,0.11594654866455,14.6466358474442));
#49804=CARTESIAN_POINT('Ctrl Pts',(22.5036614591591,-2.4588269515588,15.2433077276005));
#49805=CARTESIAN_POINT('Ctrl Pts',(22.3647499686705,-4.43454543016366,16.9988738480645));
#49806=CARTESIAN_POINT('Ctrl Pts',(22.2258384781818,-5.32985574631102,19.4856177729232));
#49807=CARTESIAN_POINT('Ctrl Pts',(22.0869269876932,-4.92662943819308,22.097682943332));
#49808=CARTESIAN_POINT('Ctrl Pts',(21.9480154972046,-3.3231063370325,24.1986802241647));
#49809=CARTESIAN_POINT('Ctrl Pts',(21.8091040067159,-0.90995995705217,25.2767342389567));
#49810=CARTESIAN_POINT('Ctrl Pts',(21.6701925162273,1.72488404235526,25.0691938602154));
#49811=CARTESIAN_POINT('Ctrl Pts',(21.5312810257386,3.93948681794363,23.6266230798452));
#49812=CARTESIAN_POINT('Ctrl Pts',(21.39236953525,5.19429477779974,21.3004818773591));
#49813=CARTESIAN_POINT('Ctrl Pts',(21.2534580447613,5.18359343923419,18.65749845112));
#49814=CARTESIAN_POINT('Ctrl Pts',(21.1145465542728,3.9099900172857,16.341594689384));
#49815=CARTESIAN_POINT('Ctrl Pts',(20.9756350637841,1.68377821724532,14.9170045969775));
#49816=CARTESIAN_POINT('Ctrl Pts',(20.8367235732955,-0.952660010357647,
14.7308074378818));
#49817=CARTESIAN_POINT('Ctrl Pts',(20.6978120828068,-3.35699741332223,15.8283672598172));
#49818=CARTESIAN_POINT('Ctrl Pts',(20.5589005923182,-4.94345450277555,17.9422806481434));
#49819=CARTESIAN_POINT('Ctrl Pts',(20.4199891018296,-5.32551563335403,20.5575254172851));
#49820=CARTESIAN_POINT('Ctrl Pts',(20.2810776113409,-4.41009754082334,23.0369377722372));
#49821=CARTESIAN_POINT('Ctrl Pts',(20.1421661208523,-2.42022763460054,24.7764473773646));
#49822=CARTESIAN_POINT('Ctrl Pts',(20.0032546303637,0.159293168790149,25.3522497174921));
#49823=CARTESIAN_POINT('Ctrl Pts',(19.864343139875,2.70000466410295,24.6240594898681));
#49824=CARTESIAN_POINT('Ctrl Pts',(19.7254316493864,4.58290193161955,22.7692889407165));
#49825=CARTESIAN_POINT('Ctrl Pts',(19.5865201588977,5.34924627784126,20.2398241251803));
#49826=CARTESIAN_POINT('Ctrl Pts',(19.4476086684091,4.812329797764,17.6519298840176));
#49827=CARTESIAN_POINT('Ctrl Pts',(19.3086971779205,3.10296385791202,15.6361064806175));
#49828=CARTESIAN_POINT('Ctrl Pts',(19.1697856874318,0.63760893729653,14.6834779982496));
#49829=CARTESIAN_POINT('Ctrl Pts',(19.0308741969432,-1.98308950412843,15.0261375802468));
#49830=CARTESIAN_POINT('Ctrl Pts',(18.8919627064546,-4.12063896875621,16.5806015381087));
#49831=CARTESIAN_POINT('Ctrl Pts',(18.7530512159659,-5.25425870789218,18.9681488563963));
#49832=CARTESIAN_POINT('Ctrl Pts',(18.6141397254773,-5.10775986778052,21.6070906897583));
#49833=CARTESIAN_POINT('Ctrl Pts',(18.4752282349886,-3.7168346169061,23.8544898213103));
#49834=CARTESIAN_POINT('Ctrl Pts',(18.3363167445,-1.42036030314568,25.1628023360638));
#49835=CARTESIAN_POINT('Ctrl Pts',(18.1974052540114,1.22216275209595,25.2132781970087));
#49836=CARTESIAN_POINT('Ctrl Pts',(18.0584937635228,3.56692482281038,23.9936197440964));
#49837=CARTESIAN_POINT('Ctrl Pts',(17.9195822730341,5.04266102511817,21.8009778282287));
#49838=CARTESIAN_POINT('Ctrl Pts',(17.7806707825454,5.28983113923432,19.1695556187174));
#49839=CARTESIAN_POINT('Ctrl Pts',(17.6417592920568,4.24821600335025,16.7404582928123));
#49840=CARTESIAN_POINT('Ctrl Pts',(17.5028478015682,2.17158897770571,15.1054977102953));
#49841=CARTESIAN_POINT('Ctrl Pts',(17.3639363110796,-0.434111995644343,
14.6630066397592));
#49842=CARTESIAN_POINT('Ctrl Pts',(17.2250248205909,-2.93404831940373,15.5207911623345));
#49843=CARTESIAN_POINT('Ctrl Pts',(17.0861133301023,-4.719149311504,17.4698653933539));
#49844=CARTESIAN_POINT('Ctrl Pts',(16.9472018396136,-5.35450282298902,20.0353676493391));
#49845=CARTESIAN_POINT('Ctrl Pts',(16.808290349125,-4.6853148325402,22.5922531265283));
#49846=CARTESIAN_POINT('Ctrl Pts',(16.6693788586364,-2.87462260710757,24.5175763655663));
#49847=CARTESIAN_POINT('Ctrl Pts',(16.5304673681477,-0.363573202429767,
25.3422622435156));
#49848=CARTESIAN_POINT('Ctrl Pts',(16.3915558776591,2.23605516975252,24.8653888467254));
#49849=CARTESIAN_POINT('Ctrl Pts',(16.2526443871705,4.29090340716083,23.2031389764468));
#49850=CARTESIAN_POINT('Ctrl Pts',(16.1137328966818,5.30033963145057,20.7604940126599));
#49851=CARTESIAN_POINT('Ctrl Pts',(15.9748214061932,5.01843037472102,18.1325664868343));
#49852=CARTESIAN_POINT('Ctrl Pts',(15.8359099157046,3.51385845166871,15.9596101507833));
#49853=CARTESIAN_POINT('Ctrl Pts',(15.6969984252159,1.15318945785908,14.7710320878495));
#49854=CARTESIAN_POINT('Ctrl Pts',(15.5580869347273,-1.48843624791842,14.8564108943366));
#49855=CARTESIAN_POINT('Ctrl Pts',(15.4191754442387,-3.76742756492399,16.1949453492666));
#49856=CARTESIAN_POINT('Ctrl Pts',(15.28026395375,-5.12854363254664,18.4605223090014));
#49857=CARTESIAN_POINT('Ctrl Pts',(15.1413524632614,-5.24016964772018,21.1011691128656));
#49858=CARTESIAN_POINT('Ctrl Pts',(15.0024409727727,-4.07510966447109,23.4735331543762));
#49859=CARTESIAN_POINT('Ctrl Pts',(14.8635294822841,-1.91721246402803,24.9996247578986));
#49860=CARTESIAN_POINT('Ctrl Pts',(14.7246179917955,0.707783794914243,25.3076353917422));
#49861=CARTESIAN_POINT('Ctrl Pts',(14.5857065013068,3.16033951822035,24.3225230458138));
#49862=CARTESIAN_POINT('Ctrl Pts',(14.4467950108182,4.84292757169553,22.284295052599));
#49863=CARTESIAN_POINT('Ctrl Pts',(14.3078835203295,5.3456114927064,19.6895340259188));
#49864=CARTESIAN_POINT('Ctrl Pts',(14.1689720298409,4.54592014639849,17.1704132148695));
#49865=CARTESIAN_POINT('Ctrl Pts',(14.0300605393523,2.63868591674534,15.3406773040723));
#49866=CARTESIAN_POINT('Ctrl Pts',(13.8911490488637,0.0885768203195806,
14.6461130476149));
#49867=CARTESIAN_POINT('Ctrl Pts',(13.752237558375,-2.48311264351585,15.255940245778));
#49868=CARTESIAN_POINT('Ctrl Pts',(13.6133260678864,-4.44983025384227,17.0215839672727));
#49869=CARTESIAN_POINT('Ctrl Pts',(13.4744145773977,-5.33241579166802,19.5128725251163));
#49870=CARTESIAN_POINT('Ctrl Pts',(13.3355030869091,-4.91584098991347,22.1228421311778));
#49871=CARTESIAN_POINT('Ctrl Pts',(13.1965915964205,-3.30159783308474,24.2156142020573));
#49872=CARTESIAN_POINT('Ctrl Pts',(13.0576801059318,-0.882971610574968,
25.2813173060266));
#49873=CARTESIAN_POINT('Ctrl Pts',(12.9187686154432,1.75077693964727,25.0603094233076));
#49874=CARTESIAN_POINT('Ctrl Pts',(12.7798571249545,3.95797586352647,23.6064356941111));
#49875=CARTESIAN_POINT('Ctrl Pts',(12.6409456344659,5.20087540269829,21.2739098859907));
#49876=CARTESIAN_POINT('Ctrl Pts',(12.5020341439773,5.17666237633432,18.6310157073721));
#49877=CARTESIAN_POINT('Ctrl Pts',(12.3631226534886,3.89123591248115,16.3216533027141));
#49878=CARTESIAN_POINT('Ctrl Pts',(12.224211163,1.65777021707646,14.9084629767239));
#49879=CARTESIAN_POINT('Ctrl Pts',(12.0852996725114,-0.979585460337544,
14.7357466172389));
#49880=CARTESIAN_POINT('Ctrl Pts',(11.9463881820227,-3.37828034515378,15.8455838843991));
#49881=CARTESIAN_POINT('Ctrl Pts',(11.8074766915341,-4.95390966046493,17.9675801546016));
#49882=CARTESIAN_POINT('Ctrl Pts',(11.6685652010455,-5.32259578001186,20.584743973562));
#49883=CARTESIAN_POINT('Ctrl Pts',(11.5296537105568,-4.3945140533954,23.0594439995737));
#49884=CARTESIAN_POINT('Ctrl Pts',(11.3907422200682,-2.39577718791672,24.7887579828046));
#49885=CARTESIAN_POINT('Ctrl Pts',(11.2518307295796,0.18665360290738,25.3513654131015));
#49886=CARTESIAN_POINT('Ctrl Pts',(11.1129192390909,2.72360914056088,24.6101957226858));
#49887=CARTESIAN_POINT('Ctrl Pts',(10.9740077486023,4.59699958611036,22.7458234024274));
#49888=CARTESIAN_POINT('Ctrl Pts',(10.8350962581136,5.35040243566758,20.212473829964));
#49889=CARTESIAN_POINT('Ctrl Pts',(10.696184767625,4.80026277901695,17.6273583067809));
#49890=CARTESIAN_POINT('Ctrl Pts',(10.5572732771364,3.0806136044089,15.620300104762));
#49891=CARTESIAN_POINT('Ctrl Pts',(10.4183617866477,0.610420741389864,14.6802878019109));
#49892=CARTESIAN_POINT('Ctrl Pts',(10.2794502961591,-2.00849166051248,15.0363408052457));
#49893=CARTESIAN_POINT('Ctrl Pts',(10.1405388056705,-4.13806624449883,16.6017123270453));
#49894=CARTESIAN_POINT('Ctrl Pts',(10.0016273151818,-5.2594652177594,18.9950238932212));
#49895=CARTESIAN_POINT('Ctrl Pts',(9.86271582469318,-5.09947712645691,21.6331822888948));
#49896=CARTESIAN_POINT('Ctrl Pts',(9.72380433420456,-3.6970805857531,23.8734411696145));
#49897=CARTESIAN_POINT('Ctrl Pts',(9.58489284371592,-1.39394774523797,25.1699962316778));
#49898=CARTESIAN_POINT('Ctrl Pts',(9.44598135322729,1.24879882699148,25.2069619589279));
#49899=CARTESIAN_POINT('Ctrl Pts',(9.30706986273864,3.58729494848217,23.9753322256902));
#49900=CARTESIAN_POINT('Ctrl Pts',(9.16815837225,5.05180233662483,21.775174499504));
#49901=CARTESIAN_POINT('Ctrl Pts',(9.02924688176137,5.28551649791576,19.1425230602066));
#49902=CARTESIAN_POINT('Ctrl Pts',(8.89033539127272,4.23149660459327,16.7187825678062));
#49903=CARTESIAN_POINT('Ctrl Pts',(8.7514239007841,2.14653824350431,15.0944597727477));
#49904=CARTESIAN_POINT('Ctrl Pts',(8.61251241029546,-0.461390842731537,
14.6652957118262));
#49905=CARTESIAN_POINT('Ctrl Pts',(8.47360091980683,-2.95690921169756,15.5358495471372));
#49906=CARTESIAN_POINT('Ctrl Pts',(8.33468942931818,-4.73202254743652,17.4940243491667));
#49907=CARTESIAN_POINT('Ctrl Pts',(8.19577793882955,-5.3542520384395,20.0627412215658));
#49908=CARTESIAN_POINT('Ctrl Pts',(8.05686644834092,-4.67200112727156,22.6161721691797));
#49909=CARTESIAN_POINT('Ctrl Pts',(7.91795495785228,-2.85148965875746,24.5322133751641));
#49910=CARTESIAN_POINT('Ctrl Pts',(7.77904346736365,-0.336256994801425,
25.3440511398624));
#49911=CARTESIAN_POINT('Ctrl Pts',(7.640131976875,2.26089946666399,24.8538937929929));
#49912=CARTESIAN_POINT('Ctrl Pts',(7.50122048638638,4.30722286603815,23.1811605640544));
#49913=CARTESIAN_POINT('Ctrl Pts',(7.36230899589773,5.30415826944371,20.7333869406452));
#49914=CARTESIAN_POINT('Ctrl Pts',(7.22339750540911,5.00881783995471,18.1069349725462));
#49915=CARTESIAN_POINT('Ctrl Pts',(7.08448601492045,3.49315668903596,15.9416989148339));
#49916=CARTESIAN_POINT('Ctrl Pts',(6.94557452443183,1.1264421304992,14.7652049248654));
#49917=CARTESIAN_POINT('Ctrl Pts',(6.80666303394318,-1.51471256885767,14.8640875021315));
#49918=CARTESIAN_POINT('Ctrl Pts',(6.66775154345456,-3.78683106169839,16.2142554415052));
#49919=CARTESIAN_POINT('Ctrl Pts',(6.52884005296591,-5.13634694434205,18.4867612814347));
#49920=CARTESIAN_POINT('Ctrl Pts',(6.38992856247729,-5.23447161873823,21.1279442471333));
#49921=CARTESIAN_POINT('Ctrl Pts',(6.25101707198864,-4.05729853103018,23.4943211046092));
#49922=CARTESIAN_POINT('Ctrl Pts',(6.11210558150001,-1.89162763233226,25.0093608626864));
#49923=CARTESIAN_POINT('Ctrl Pts',(5.97319409101137,0.734908977741772,25.303947600274));
#49924=CARTESIAN_POINT('Ctrl Pts',(5.83428260052273,3.18239642241211,24.3063098312401));
#49925=CARTESIAN_POINT('Ctrl Pts',(5.69537111003409,4.85454237490546,22.2595065129944));
#49926=CARTESIAN_POINT('Ctrl Pts',(5.55645961954546,5.34395442841376,19.6622095041981));
#49927=CARTESIAN_POINT('Ctrl Pts',(5.41754812905682,4.53139493259768,17.1472099066274));
#49928=CARTESIAN_POINT('Ctrl Pts',(5.27863663856819,2.61483139632318,15.3272483352077));
#49929=CARTESIAN_POINT('Ctrl Pts',(5.13972514807955,0.0612047769146592,
14.6457301779514));
#49930=CARTESIAN_POINT('Ctrl Pts',(5.00081365759091,-2.50733343638805,15.2686967555665));
#49931=CARTESIAN_POINT('Ctrl Pts',(4.86190216710228,-4.46499877594587,17.0443719309055));
#49932=CARTESIAN_POINT('Ctrl Pts',(4.72299067661364,-5.33483646803344,19.540140008962));
#49933=CARTESIAN_POINT('Ctrl Pts',(4.584079186125,-4.90492406031727,22.1479458360344));
#49934=CARTESIAN_POINT('Ctrl Pts',(4.44516769563637,-3.28000303797389,24.2324379998885));
#49935=CARTESIAN_POINT('Ctrl Pts',(4.30625620514774,-0.855960186590904,
25.2857623396237));
#49936=CARTESIAN_POINT('Ctrl Pts',(4.16734471465909,1.77662407831394,25.0512927292309));
#49937=CARTESIAN_POINT('Ctrl Pts',(4.02843322417046,3.97636146273007,23.5861540499144));
#49938=CARTESIAN_POINT('Ctrl Pts',(3.88952173368182,5.20732009656954,21.2473045994844));
#49939=CARTESIAN_POINT('Ctrl Pts',(3.75061024319318,5.16959601524122,18.6045687436407));
#49940=CARTESIAN_POINT('Ctrl Pts',(3.61169875270455,3.87238010562758,16.3018080539971));
#49941=CARTESIAN_POINT('Ctrl Pts',(3.47278726221591,1.6317188891182,14.9000544297852));
#49942=CARTESIAN_POINT('Ctrl Pts',(3.33387577172727,-1.00648530768362,14.740823384132));
#49943=CARTESIAN_POINT('Ctrl Pts',(3.19496428123864,-3.39947498165274,15.8629090894604));
#49944=CARTESIAN_POINT('Ctrl Pts',(3.05605279075,-4.96423534183138,17.992932780948));
#49945=CARTESIAN_POINT('Ctrl Pts',(2.91714130026136,-5.31953681440784,20.611947246485));
#49946=CARTESIAN_POINT('Ctrl Pts',(2.77822980977274,-4.37881571000473,23.0818702654696));
#49947=CARTESIAN_POINT('Ctrl Pts',(2.6393183192841,-2.37126412504296,24.8009434269244));
#49948=CARTESIAN_POINT('Ctrl Pts',(2.50040682879546,0.214009159162442,25.3503412473393));
#49949=CARTESIAN_POINT('Ctrl Pts',(2.36149533830682,2.74714243118999,24.596211456896));
#49950=CARTESIAN_POINT('Ctrl Pts',(2.22258384781819,4.61097709471508,22.7222861100022));
#49951=CARTESIAN_POINT('Ctrl Pts',(2.08367235732956,5.35141875019975,20.1851179594327));
#49952=CARTESIAN_POINT('Ctrl Pts',(1.94476086684092,4.7880703079961,17.6028487847724));
#49953=CARTESIAN_POINT('Ctrl Pts',(1.80584937635228,3.05818281914584,15.6046081120332));
#49954=CARTESIAN_POINT('Ctrl Pts',(1.66693788586364,0.583216623469168,14.6772368108884));
#49955=CARTESIAN_POINT('Ctrl Pts',(1.528026395375,-2.03384138569939,15.0466734299052));
#49956=CARTESIAN_POINT('Ctrl Pts',(1.38911490488637,-4.15538524274299,16.6229125867855));
#49957=CARTESIAN_POINT('Ctrl Pts',(1.25020341439773,-5.26453450989542,19.0219239115778));
#49958=CARTESIAN_POINT('Ctrl Pts',(1.11129192390909,-5.09106062268244,21.6592337321965));
#49959=CARTESIAN_POINT('Ctrl Pts',(0.972380433420454,-3.67723087516871,
23.8922863012608));
#49960=CARTESIAN_POINT('Ctrl Pts',(0.833468942931815,-1.36749688817716,
25.1770648073967));
#49961=CARTESIAN_POINT('Ctrl Pts',(0.694557452443176,1.2753985880402,25.2004903273098));
#49962=CARTESIAN_POINT('Ctrl Pts',(0.555645961954543,3.60757855033071,23.9569788265186));
#49963=CARTESIAN_POINT('Ctrl Pts',(0.416734471465908,5.06079738115399,21.749249752767));
#49964=CARTESIAN_POINT('Ctrl Pts',(0.277822980977272,5.28109160991654,19.1156625541981));
#49965=CARTESIAN_POINT('Ctrl Pts',(0.138911490488646,4.21461302406515,16.6968760766832));
#49966=CARTESIAN_POINT('Ctrl Pts',(0.046303830162886,2.8192119327481,15.6219268293179));
#49967=CARTESIAN_POINT('Ctrl Pts',(8.88178419700125E-15,2.03511426366979,
15.2835913560944));
#49968=CARTESIAN_POINT('Ctrl Pts',(8.88178419700125E-15,2.03511426366979,
15.2835913560944));
#49969=CARTESIAN_POINT('Ctrl Pts',(9.32284291588981E-15,2.1755902259129,
15.3291667179724));
#49970=CARTESIAN_POINT('Ctrl Pts',(2.51669497179419E-15,2.31375853724984,
15.3808402235287));
#49971=CARTESIAN_POINT('Ctrl Pts',(3.88578058618805E-15,2.44931788544433,
15.4382685188975));
#49972=CARTESIAN_POINT('Ctrl Pts',(5.27910699501164E-15,2.58727742414413,
15.4967136297874));
#49973=CARTESIAN_POINT('Ctrl Pts',(1.13067933023619E-14,2.72253541261565,
15.5611192658562));
#49974=CARTESIAN_POINT('Ctrl Pts',(9.76996261670138E-15,2.85477467194667,
15.6311776903917));
#49975=CARTESIAN_POINT('Ctrl Pts',(8.21074211962818E-15,2.98894050139723,
15.702256783585));
#49976=CARTESIAN_POINT('Ctrl Pts',(2.17675697203127E-14,3.11999970392103,
15.7791547732152));
#49977=CARTESIAN_POINT('Ctrl Pts',(2.56461518688411E-14,3.24761139159044,
15.861602893881));
#49978=CARTESIAN_POINT('Ctrl Pts',(2.9518609317083E-14,3.3750215666168,
15.9439208200559));
#49979=CARTESIAN_POINT('Ctrl Pts',(8.03728488918813E-15,3.4989958079745,
16.0317717068427));
#49980=CARTESIAN_POINT('Ctrl Pts',(8.04911692853238E-15,3.6191747643727,
16.1249358268418));
#49981=CARTESIAN_POINT('Ctrl Pts',(8.05250885098475E-15,3.65362678812349,
16.1516434349882));
#49982=CARTESIAN_POINT('Ctrl Pts',(1.34374591162967E-14,3.68776674753865,
16.1787879738458));
#49983=CARTESIAN_POINT('Ctrl Pts',(1.32116539930394E-14,3.72158574495427,
16.2063649308754));
#49984=CARTESIAN_POINT('Ctrl Pts',(1.30778498935537E-14,3.74162568217725,
16.2227060565711));
#49985=CARTESIAN_POINT('Ctrl Pts',(5.34802515091838E-15,3.76155291509913,
16.239199023854));
#49986=CARTESIAN_POINT('Ctrl Pts',(5.16253706450698E-15,3.78136555481421,
16.255842940216));
#49987=CARTESIAN_POINT('Ctrl Pts',(5.02425027734796E-15,3.79613645651655,
16.2682514660894));
#49988=CARTESIAN_POINT('Ctrl Pts',(1.38281244415282E-14,3.81084283987857,
16.2807432594011));
#49989=CARTESIAN_POINT('Ctrl Pts',(1.38777878078145E-14,3.82547437708717,
16.2933095461151));
#49990=CARTESIAN_POINT('Ctrl Pts',(1.42788781872578E-14,3.94364133292775,
16.3947971633111));
#49991=CARTESIAN_POINT('Ctrl Pts',(2.05682746198613E-14,4.05709628359361,
16.5012804183751));
#49992=CARTESIAN_POINT('Ctrl Pts',(1.84297022087776E-14,4.16550570005553,
16.6124427404842));
#49993=CARTESIAN_POINT('Ctrl Pts',(1.79821344800749E-14,4.18819399250913,
16.6357071704216));
#49994=CARTESIAN_POINT('Ctrl Pts',(6.4338797725629E-15,4.21066124423878,
16.6591767169253));
#49995=CARTESIAN_POINT('Ctrl Pts',(6.0507154842071E-15,4.2329043100469,
16.6828487513009));
#49996=CARTESIAN_POINT('Ctrl Pts',(4.23927623984675E-15,4.33806014931527,
16.7947601516193));
#49997=CARTESIAN_POINT('Ctrl Pts',(1.36309249628105E-14,4.4382076506583,
16.9111934994602));
#49998=CARTESIAN_POINT('Ctrl Pts',(1.2490009027033E-14,4.5332160691296,
17.0317215451736));
#49999=CARTESIAN_POINT('Ctrl Pts',(1.1335668032986E-14,4.62934244337141,
17.1536678338847));
#50000=CARTESIAN_POINT('Ctrl Pts',(6.63949211684557E-15,4.72020856568058,
17.2798062617839));
#50001=CARTESIAN_POINT('Ctrl Pts',(6.93889390390723E-15,4.80564662961519,
17.4097367836627));
#50002=CARTESIAN_POINT('Ctrl Pts',(7.23151701427986E-15,4.88915031293694,
17.5367255829536));
#50003=CARTESIAN_POINT('Ctrl Pts',(-4.03556871303723E-15,4.96746921735247,
17.6673373941001));
#50004=CARTESIAN_POINT('Ctrl Pts',(-6.16173778666962E-15,5.0404106198303,
17.8012298339498));
#50005=CARTESIAN_POINT('Ctrl Pts',(-6.60825461783724E-15,5.05572904596076,
17.8293485892739));
#50006=CARTESIAN_POINT('Ctrl Pts',(3.02869902184406E-15,5.07081016404348,
17.8576121252524));
#50007=CARTESIAN_POINT('Ctrl Pts',(3.10862446895044E-15,5.08565196321491,
17.8860174072779));
#50008=CARTESIAN_POINT('Ctrl Pts',(3.15744306202177E-15,5.0947173582853,
17.9033673997332));
#50009=CARTESIAN_POINT('Ctrl Pts',(1.36778384139571E-15,5.10369272421503,
17.9207689458792));
#50010=CARTESIAN_POINT('Ctrl Pts',(1.4432899320127E-15,5.11257226278412,
17.9382105143602));
#50011=CARTESIAN_POINT('Ctrl Pts',(2.05664622361767E-15,5.18470314392759,
18.079893068388));
#50012=CARTESIAN_POINT('Ctrl Pts',(7.16626964594806E-16,5.25061395420093,
18.2244048189638));
#50013=CARTESIAN_POINT('Ctrl Pts',(-1.11022302462516E-15,5.31017458672414,
18.3712949565427));
#50014=CARTESIAN_POINT('Ctrl Pts',(-2.95761469161467E-15,5.37040493779473,
18.519836773182));
#50015=CARTESIAN_POINT('Ctrl Pts',(1.14248619537007E-14,5.42414199716124,
18.6708113453056));
#50016=CARTESIAN_POINT('Ctrl Pts',(9.76996261670138E-15,5.47121450010452,
18.8237908267476));
#50017=CARTESIAN_POINT('Ctrl Pts',(8.88107335987433E-15,5.49649835950476,
18.9059600647965));
#50018=CARTESIAN_POINT('Ctrl Pts',(-1.31658901812416E-14,5.51985879624915,
18.9887083281946));
#50019=CARTESIAN_POINT('Ctrl Pts',(-1.43218770176645E-14,5.54126420042667,
19.0719728906149));
#50020=CARTESIAN_POINT('Ctrl Pts',(-1.64684981599728E-14,5.5809146660826,
19.226208645531));
#50021=CARTESIAN_POINT('Ctrl Pts',(7.69447901493824E-15,5.61385999669503,
19.3822149699441));
#50022=CARTESIAN_POINT('Ctrl Pts',(8.32667268468867E-15,5.64014328124797,
19.5395658386989));
#50023=CARTESIAN_POINT('Ctrl Pts',(8.72173319680612E-15,5.65656781751344,
19.6378950655905));
#50024=CARTESIAN_POINT('Ctrl Pts',(-8.32468647422183E-15,5.67038981606524,
19.7367497662378));
#50025=CARTESIAN_POINT('Ctrl Pts',(-9.04831765069503E-15,5.68160986215254,
19.8360286798643));
#50026=CARTESIAN_POINT('Ctrl Pts',(-9.32229125156183E-15,5.68585787761729,
19.873616614631));
#50027=CARTESIAN_POINT('Ctrl Pts',(-9.03082511654983E-15,5.68973283677329,
19.911265372205));
#50028=CARTESIAN_POINT('Ctrl Pts',(-9.10382880192628E-15,5.69323448040224,
19.948969495901));
#50029=CARTESIAN_POINT('Ctrl Pts',(-9.14545097407185E-15,5.69523090035235,
19.9704660480131));
#50030=CARTESIAN_POINT('Ctrl Pts',(-1.69075485132513E-14,5.69710600165537,
19.991981655482));
#50031=CARTESIAN_POINT('Ctrl Pts',(-1.68198788230711E-14,5.69885847879252,
20.013498207624));
#50032=CARTESIAN_POINT('Ctrl Pts',(-1.61588887191719E-14,5.71207136961703,
20.1757233507338));
#50033=CARTESIAN_POINT('Ctrl Pts',(6.30550755751366E-15,5.71833945842108,
20.3382232791638));
#50034=CARTESIAN_POINT('Ctrl Pts',(3.96904731303493E-15,5.7177783220589,
20.500534488949));
#50035=CARTESIAN_POINT('Ctrl Pts',(1.60991114576845E-15,5.71721173972995,
20.6644209690473));
#50036=CARTESIAN_POINT('Ctrl Pts',(-2.78263791069445E-14,5.70968286987112,
20.8281157599009));
#50037=CARTESIAN_POINT('Ctrl Pts',(-2.39530617562878E-14,5.69526111488175,
20.9911627693061));
#50038=CARTESIAN_POINT('Ctrl Pts',(-2.00744932912372E-14,5.68081980810295,
21.154430823986));
#50039=CARTESIAN_POINT('Ctrl Pts',(-1.1625797255892E-14,5.65946699454297,
21.3170501028641));
#50040=CARTESIAN_POINT('Ctrl Pts',(-1.21846976952611E-14,5.63122133755543,
21.4785725032748));
#50041=CARTESIAN_POINT('Ctrl Pts',(-1.26905279506821E-14,5.60565773645204,
21.6247576040562));
#50042=CARTESIAN_POINT('Ctrl Pts',(1.23920388915437E-16,5.57444757028604,
21.7700447797953));
#50043=CARTESIAN_POINT('Ctrl Pts',(7.49400541621981E-16,5.53756786262954,
21.9141008375364));
#50044=CARTESIAN_POINT('Ctrl Pts',(1.06565608626021E-15,5.52213270144179,
21.9743922176096));
#50045=CARTESIAN_POINT('Ctrl Pts',(-1.01203093583408E-14,5.50570400498667,
22.0344678920767));
#50046=CARTESIAN_POINT('Ctrl Pts',(-1.09356967925578E-14,5.48829300650687,
22.0943080987843));
#50047=CARTESIAN_POINT('Ctrl Pts',(-1.13800492473829E-14,5.4788047318649,
22.1269185384746));
#50048=CARTESIAN_POINT('Ctrl Pts',(-2.68295561497439E-15,5.46902471491014,
22.1594590442228));
#50049=CARTESIAN_POINT('Ctrl Pts',(-2.24820162486594E-15,5.45895464414269,
22.1919263783269));
#50050=CARTESIAN_POINT('Ctrl Pts',(-1.96639678768615E-15,5.45242728679215,
22.2129715027168));
#50051=CARTESIAN_POINT('Ctrl Pts',(-7.76142744149267E-15,5.44578086478645,
22.2339768276455));
#50052=CARTESIAN_POINT('Ctrl Pts',(-7.66053886991358E-15,5.43901644566141,
22.2549406076277));
#50053=CARTESIAN_POINT('Ctrl Pts',(-6.90260989493124E-15,5.38819850688457,
22.4124317488445));
#50054=CARTESIAN_POINT('Ctrl Pts',(-6.54588297085908E-15,5.33072013492139,
22.5675950757115));
#50055=CARTESIAN_POINT('Ctrl Pts',(-5.78703751585863E-15,5.26688451533375,
22.720075001107));
#50056=CARTESIAN_POINT('Ctrl Pts',(-5.01909383498359E-15,5.20228353452266,
22.8743830942717));
#50057=CARTESIAN_POINT('Ctrl Pts',(-2.52391800493359E-15,5.13117177003407,
23.0259437296997));
#50058=CARTESIAN_POINT('Ctrl Pts',(-2.63677968348475E-16,5.05381061639661,
23.1743822794189));
#50059=CARTESIAN_POINT('Ctrl Pts',(6.63362861739138E-16,5.02208082357648,
23.2352645725034));
#50060=CARTESIAN_POINT('Ctrl Pts',(-4.63064774168416E-15,4.98929913677184,
23.295621526562));
#50061=CARTESIAN_POINT('Ctrl Pts',(-4.95437024738976E-15,4.95548117923701,
23.3554265883461));
#50062=CARTESIAN_POINT('Ctrl Pts',(-5.1966435182712E-15,4.9301718879703,
23.4001845760619));
#50063=CARTESIAN_POINT('Ctrl Pts',(-3.73619989753743E-15,4.90428215327493,
23.4446334404272));
#50064=CARTESIAN_POINT('Ctrl Pts',(-3.52495810318487E-15,4.87781803474678,
23.4887618409189));
#50065=CARTESIAN_POINT('Ctrl Pts',(-3.41302455827604E-15,4.86379513454929,
23.5121447529667));
#50066=CARTESIAN_POINT('Ctrl Pts',(-5.11817456332583E-15,4.84961584756207,
23.5354295002362));
#50067=CARTESIAN_POINT('Ctrl Pts',(-5.37070388162419E-15,4.83528275213712,
23.5586123876325));
#50068=CARTESIAN_POINT('Ctrl Pts',(-6.94795543784049E-15,4.74576088110552,
23.7034084274336));
#50069=CARTESIAN_POINT('Ctrl Pts',(9.10527509405812E-15,4.65022657721916,
23.844259359632));
#50070=CARTESIAN_POINT('Ctrl Pts',(6.18255446838134E-15,4.54896272516647,
23.9807849350336));
#50071=CARTESIAN_POINT('Ctrl Pts',(3.25413836088581E-15,4.44750154107212,
24.1175765567093));
#50072=CARTESIAN_POINT('Ctrl Pts',(-5.59205196868429E-15,4.34028815806525,
24.2500266576816));
#50073=CARTESIAN_POINT('Ctrl Pts',(-5.15212872365112E-15,4.22755843067459,
24.3777346172277));
#50074=CARTESIAN_POINT('Ctrl Pts',(-5.0011400422891E-15,4.18886778842919,
24.4215660278862));
#50075=CARTESIAN_POINT('Ctrl Pts',(-3.56011120575155E-15,4.14952693581179,
24.4648386217493));
#50076=CARTESIAN_POINT('Ctrl Pts',(-4.29691004999455E-15,4.10954418789613,
24.5075354759874));
#50077=CARTESIAN_POINT('Ctrl Pts',(-5.03699156543988E-15,4.06880057339034,
24.5510448459126));
#50078=CARTESIAN_POINT('Ctrl Pts',(-5.30426572712612E-15,4.0273904007291,
24.5939563600081));
#50079=CARTESIAN_POINT('Ctrl Pts',(-5.27355936696949E-15,3.98533038287153,
24.6362610213063));
#50080=CARTESIAN_POINT('Ctrl Pts',(48.4490415053031,-5.1367692385953,19.9998673509107));
#50081=CARTESIAN_POINT('Ctrl Pts',(48.4130939002172,-5.13608619358257,20.6628267235351));
#50082=CARTESIAN_POINT('Ctrl Pts',(48.3771462951314,-5.00715967363253,21.3260440301722));
#50083=CARTESIAN_POINT('Ctrl Pts',(48.3411986900455,-4.75688882502728,21.9397791588711));
#50084=CARTESIAN_POINT('Ctrl Pts',(48.2948948598826,-4.43451689396667,22.7303265985789));
#50085=CARTESIAN_POINT('Ctrl Pts',(48.2485910297197,-3.91081269191307,23.4387741217238));
#50086=CARTESIAN_POINT('Ctrl Pts',(48.2022871995568,-3.24957242287801,23.9788206184102));
#50087=CARTESIAN_POINT('Ctrl Pts',(48.155983369394,-2.58833215384294,24.5188671150965));
#50088=CARTESIAN_POINT('Ctrl Pts',(48.1096795392311,-1.78955581782641,24.8905125853242));
#50089=CARTESIAN_POINT('Ctrl Pts',(48.0633757090682,-0.950548140765501,
25.0484841981418));
#50090=CARTESIAN_POINT('Ctrl Pts',(48.0170718789054,-0.111540463704582,
25.2064558109594));
#50091=CARTESIAN_POINT('Ctrl Pts',(47.9707680487424,0.767698554400724,25.1507535663667));
#50092=CARTESIAN_POINT('Ctrl Pts',(47.9244642185796,1.58006244277662,24.8881629609726));
#50093=CARTESIAN_POINT('Ctrl Pts',(47.8781603884167,2.3924263311525,24.6255723555784));
#50094=CARTESIAN_POINT('Ctrl Pts',(47.8318565582538,3.13791508979897,24.1560933893826));
#50095=CARTESIAN_POINT('Ctrl Pts',(47.7855527280909,3.72571533683517,23.5369166923885));
#50096=CARTESIAN_POINT('Ctrl Pts',(47.7392488979281,4.31351558387138,22.9177399953943));
#50097=CARTESIAN_POINT('Ctrl Pts',(47.6929450677652,4.74362731929732,22.1488655676018));
#50098=CARTESIAN_POINT('Ctrl Pts',(47.6466412376023,4.96365551870842,21.3239555698276));
#50099=CARTESIAN_POINT('Ctrl Pts',(47.6003374074394,5.18368371811953,20.4990455720535));
#50100=CARTESIAN_POINT('Ctrl Pts',(47.5540335772765,5.1936283815158,19.6181000042978));
#50101=CARTESIAN_POINT('Ctrl Pts',(47.5077297471137,4.99227807759252,18.7884332230865));
#50102=CARTESIAN_POINT('Ctrl Pts',(47.4614259169508,4.79092777366925,17.9587664418752));
#50103=CARTESIAN_POINT('Ctrl Pts',(47.4151220867879,4.37828250242643,17.1803784472083));
#50104=CARTESIAN_POINT('Ctrl Pts',(47.368818256625,3.80460957149062,16.5480903157878));
#50105=CARTESIAN_POINT('Ctrl Pts',(47.3225144264621,3.23093664055482,15.9158021843672));
#50106=CARTESIAN_POINT('Ctrl Pts',(47.2762105962993,2.49623604992602,15.429613916193));
#50107=CARTESIAN_POINT('Ctrl Pts',(47.2299067661364,1.69000699719802,15.1487516237057));
#50108=CARTESIAN_POINT('Ctrl Pts',(47.1836029359735,0.883777944470023,14.8678893312184));
#50109=CARTESIAN_POINT('Ctrl Pts',(47.1372991058106,0.00602042964282193,
14.7923530144179));
#50110=CARTESIAN_POINT('Ctrl Pts',(47.0909952756477,-0.836339550193692,
14.9313442989241));
#50111=CARTESIAN_POINT('Ctrl Pts',(47.0446914454848,-1.67869953003021,15.0703355834303));
#50112=CARTESIAN_POINT('Ctrl Pts',(46.998387615322,-2.48566197487603,15.4238544692431));
#50113=CARTESIAN_POINT('Ctrl Pts',(46.9520837851592,-3.1589249475859,15.9488362616763));
#50114=CARTESIAN_POINT('Ctrl Pts',(46.9057799549963,-3.83218792029577,16.4738180541095));
#50115=CARTESIAN_POINT('Ctrl Pts',(46.8594761248333,-4.37175142086969,17.1702627531631));
#50116=CARTESIAN_POINT('Ctrl Pts',(46.8131722946705,-4.71188731332118,17.9533313883844));
#50117=CARTESIAN_POINT('Ctrl Pts',(46.7751286982147,-4.99134567750053,18.596706829482));
#50118=CARTESIAN_POINT('Ctrl Pts',(46.7370851017589,-5.13618249371292,19.2985568643818));
#50119=CARTESIAN_POINT('Ctrl Pts',(46.6990415053031,-5.13689122437247,20.0001232958892));
#50120=CARTESIAN_POINT('Ctrl Pts',(50.,-1.57888188187519,14.0941590297752));
#50121=CARTESIAN_POINT('Ctrl Pts',(50.,-1.73782238409694,14.1503790437278));
#50122=CARTESIAN_POINT('Ctrl Pts',(50.,-1.89403686188134,14.2131930374271));
#50123=CARTESIAN_POINT('Ctrl Pts',(50.,-2.04718622138767,14.2823105486562));
#50124=CARTESIAN_POINT('Ctrl Pts',(50.,-2.20154651490249,14.3519745639334));
#50125=CARTESIAN_POINT('Ctrl Pts',(50.,-2.35279365452493,14.4280426063853));
#50126=CARTESIAN_POINT('Ctrl Pts',(50.,-2.50055566660814,14.510263994692));
#50127=CARTESIAN_POINT('Ctrl Pts',(50.,-2.64732566541585,14.5919333824703));
#50128=CARTESIAN_POINT('Ctrl Pts',(50.,-2.79065771652978,14.6796742843768));
#50129=CARTESIAN_POINT('Ctrl Pts',(50.,-2.93015429364071,14.7732797038493));
#50130=CARTESIAN_POINT('Ctrl Pts',(50.,-3.06797652569821,14.8657615991873));
#50131=CARTESIAN_POINT('Ctrl Pts',(50.,-3.20205526958666,14.9639685708035));
#50132=CARTESIAN_POINT('Ctrl Pts',(50.,-3.33196742199994,15.0677313572818));
#50133=CARTESIAN_POINT('Ctrl Pts',(50.,-3.39602842604199,15.1188978429456));
#50134=CARTESIAN_POINT('Ctrl Pts',(50.,-3.45907563529118,15.171415690102));
#50135=CARTESIAN_POINT('Ctrl Pts',(50.,-3.52105417041813,15.2252668229557));
#50136=CARTESIAN_POINT('Ctrl Pts',(50.,-3.53896050140773,15.2408250514144));
#50137=CARTESIAN_POINT('Ctrl Pts',(50.,-3.55677761137173,15.2564945776178));
#50138=CARTESIAN_POINT('Ctrl Pts',(50.,-3.57450413028377,15.2722749853259));
#50139=CARTESIAN_POINT('Ctrl Pts',(50.,-3.59054569823461,15.2865554249204));
#50140=CARTESIAN_POINT('Ctrl Pts',(50.,-3.60650718940738,15.3009214523991));
#50141=CARTESIAN_POINT('Ctrl Pts',(50.,-3.62238388236175,15.3153689794615));
#50142=CARTESIAN_POINT('Ctrl Pts',(50.,-3.74452419973748,15.4265146409519));
#50143=CARTESIAN_POINT('Ctrl Pts',(50.,-3.86172403164677,15.5425475076359));
#50144=CARTESIAN_POINT('Ctrl Pts',(50.,-3.97363113502738,15.6632438417377));
#50145=CARTESIAN_POINT('Ctrl Pts',(50.,-3.99801652637559,15.6895444719252));
#50146=CARTESIAN_POINT('Ctrl Pts',(50.,-4.02215045555051,15.7160666739607));
#50147=CARTESIAN_POINT('Ctrl Pts',(50.,-4.04602902731229,15.7428083472572));
#50148=CARTESIAN_POINT('Ctrl Pts',(50.,-4.15602108936427,15.8659887375226));
#50149=CARTESIAN_POINT('Ctrl Pts',(50.,-4.26059857444806,15.9938238149227));
#50150=CARTESIAN_POINT('Ctrl Pts',(50.,-4.35955084737223,16.1259088074266));
#50151=CARTESIAN_POINT('Ctrl Pts',(50.,-4.45831511238434,16.2577428403221));
#50152=CARTESIAN_POINT('Ctrl Pts',(50.,-4.55147580303531,16.3938113843476));
#50153=CARTESIAN_POINT('Ctrl Pts',(50.,-4.63877567630947,16.5337316036845));
#50154=CARTESIAN_POINT('Ctrl Pts',(50.,-4.72210041196483,16.6672806553821));
#50155=CARTESIAN_POINT('Ctrl Pts',(50.,-4.80008581751703,16.8043392665965));
#50156=CARTESIAN_POINT('Ctrl Pts',(50.,-4.87246387825708,16.9445822178997));
#50157=CARTESIAN_POINT('Ctrl Pts',(50.,-4.89325145258022,16.9848611469523));
#50158=CARTESIAN_POINT('Ctrl Pts',(50.,-4.9135761991606,17.0254027646812));
#50159=CARTESIAN_POINT('Ctrl Pts',(50.,-4.93343106432601,17.0661993776146));
#50160=CARTESIAN_POINT('Ctrl Pts',(50.,-4.94259505699603,17.085029012506));
#50161=CARTESIAN_POINT('Ctrl Pts',(50.,-4.95165540161899,17.1039057211666));
#50162=CARTESIAN_POINT('Ctrl Pts',(50.,-4.96060966400913,17.1228243828118));
#50163=CARTESIAN_POINT('Ctrl Pts',(50.,-5.02975007299816,17.2689049807083));
#50164=CARTESIAN_POINT('Ctrl Pts',(50.,-5.09260924613714,17.4175665636468));
#50165=CARTESIAN_POINT('Ctrl Pts',(50.,-5.14899613636606,17.5684268921343));
#50166=CARTESIAN_POINT('Ctrl Pts',(50.,-5.20491428920055,17.7180331369684));
#50167=CARTESIAN_POINT('Ctrl Pts',(50.,-5.25446750278863,17.8698024305613));
#50168=CARTESIAN_POINT('Ctrl Pts',(50.,-5.29742025272067,18.0233748357436));
#50169=CARTESIAN_POINT('Ctrl Pts',(50.,-5.32033847663536,18.1053161963004));
#50170=CARTESIAN_POINT('Ctrl Pts',(50.,-5.34137672674639,18.1877710486224));
#50171=CARTESIAN_POINT('Ctrl Pts',(50.,-5.3604931415221,18.2706851930074));
#50172=CARTESIAN_POINT('Ctrl Pts',(50.,-5.39658046805671,18.4272077333405));
#50173=CARTESIAN_POINT('Ctrl Pts',(50.,-5.42582196978831,18.5853677668178));
#50174=CARTESIAN_POINT('Ctrl Pts',(50.,-5.44817286598194,18.7447104220605));
#50175=CARTESIAN_POINT('Ctrl Pts',(50.,-5.46135993546014,18.8387228789805));
#50176=CARTESIAN_POINT('Ctrl Pts',(50.,-5.47214740383625,18.9331468712938));
#50177=CARTESIAN_POINT('Ctrl Pts',(50.,-5.48051784692699,19.0278866066674));
#50178=CARTESIAN_POINT('Ctrl Pts',(50.,-5.48369364859717,19.0638314911341));
#50179=CARTESIAN_POINT('Ctrl Pts',(50.,-5.48652145884549,19.0998218024007));
#50180=CARTESIAN_POINT('Ctrl Pts',(50.,-5.48900009920885,19.1358522102154));
#50181=CARTESIAN_POINT('Ctrl Pts',(50.,-5.49086720863181,19.162993184331));
#50182=CARTESIAN_POINT('Ctrl Pts',(50.,-5.49253636532794,19.1901616141891));
#50183=CARTESIAN_POINT('Ctrl Pts',(50.,-5.49400565178386,19.2173257522691));
#50184=CARTESIAN_POINT('Ctrl Pts',(50.,-5.50252096464157,19.3747566829964));
#50185=CARTESIAN_POINT('Ctrl Pts',(50.,-5.50434139752314,19.5322154392954));
#50186=CARTESIAN_POINT('Ctrl Pts',(50.,-5.49949900939921,19.6892750140735));
#50187=CARTESIAN_POINT('Ctrl Pts',(50.,-5.49466981791964,19.845906564642));
#50188=CARTESIAN_POINT('Ctrl Pts',(50.,-5.4832139338339,20.002141867127));
#50189=CARTESIAN_POINT('Ctrl Pts',(50.,-5.46511202446615,20.1575502879913));
#50190=CARTESIAN_POINT('Ctrl Pts',(50.,-5.44732254602162,20.3102764284718));
#50191=CARTESIAN_POINT('Ctrl Pts',(50.,-5.42311424356855,20.4622046334804));
#50192=CARTESIAN_POINT('Ctrl Pts',(50.,-5.39242225163155,20.6129089430498));
#50193=CARTESIAN_POINT('Ctrl Pts',(50.,-5.36589148603084,20.7431807325253));
#50194=CARTESIAN_POINT('Ctrl Pts',(50.,-5.33451520914545,20.8725379853212));
#50195=CARTESIAN_POINT('Ctrl Pts',(50.,-5.29822455763965,21.0006893772657));
#50196=CARTESIAN_POINT('Ctrl Pts',(50.,-5.28325270927048,21.0535587287069));
#50197=CARTESIAN_POINT('Ctrl Pts',(50.,-5.26744412774905,21.1062226322689));
#50198=CARTESIAN_POINT('Ctrl Pts',(50.,-5.25080526889494,21.15866198357));
#50199=CARTESIAN_POINT('Ctrl Pts',(50.,-5.24128177427378,21.1886764145133));
#50200=CARTESIAN_POINT('Ctrl Pts',(50.,-5.23148626960332,21.2186172713547));
#50201=CARTESIAN_POINT('Ctrl Pts',(50.,-5.22141988715224,21.2484808831291));
#50202=CARTESIAN_POINT('Ctrl Pts',(50.,-5.21445283316468,21.269149817228));
#50203=CARTESIAN_POINT('Ctrl Pts',(50.,-5.20735673023832,21.2897795084358));
#50204=CARTESIAN_POINT('Ctrl Pts',(50.,-5.20013577259056,21.3103584645419));
#50205=CARTESIAN_POINT('Ctrl Pts',(50.,-5.14900190778098,21.4560845040486));
#50206=CARTESIAN_POINT('Ctrl Pts',(50.,-5.09156138048567,21.59941655586));
#50207=CARTESIAN_POINT('Ctrl Pts',(50.,-5.02803474960281,21.7399684337231));
#50208=CARTESIAN_POINT('Ctrl Pts',(50.,-4.96447673958616,21.8805897375281));
#50209=CARTESIAN_POINT('Ctrl Pts',(50.,-4.8948261396364,22.0184287712917));
#50210=CARTESIAN_POINT('Ctrl Pts',(50.,-4.81926289989551,22.1530664186381));
#50211=CARTESIAN_POINT('Ctrl Pts',(50.,-4.79092668499267,22.2035555363929));
#50212=CARTESIAN_POINT('Ctrl Pts',(50.,-4.7617586292794,22.2535940833528));
#50213=CARTESIAN_POINT('Ctrl Pts',(50.,-4.73176694583031,22.3031584989639));
#50214=CARTESIAN_POINT('Ctrl Pts',(50.,-4.71610121865025,22.3290477630367));
#50215=CARTESIAN_POINT('Ctrl Pts',(50.,-4.7002107665672,22.3548076534927));
#50216=CARTESIAN_POINT('Ctrl Pts',(50.,-4.6840966920901,22.3804347158741));
#50217=CARTESIAN_POINT('Ctrl Pts',(50.,-4.6698029103653,22.4031668707023));
#50218=CARTESIAN_POINT('Ctrl Pts',(50.,-4.65533244367626,22.4257955041634));
#50219=CARTESIAN_POINT('Ctrl Pts',(50.,-4.6406958078698,22.4483035164937));
#50220=CARTESIAN_POINT('Ctrl Pts',(50.,-4.55820044210185,22.5751637277094));
#50221=CARTESIAN_POINT('Ctrl Pts',(50.,-4.47036188468475,22.6983041039959));
#50222=CARTESIAN_POINT('Ctrl Pts',(50.,-4.37736498984394,22.8173359791823));
#50223=CARTESIAN_POINT('Ctrl Pts',(50.,-4.28579405817417,22.9345426851469));
#50224=CARTESIAN_POINT('Ctrl Pts',(50.,-4.18922125200072,23.0477663844785));
#50225=CARTESIAN_POINT('Ctrl Pts',(50.,-4.08779202142556,23.1565964011001));
#50226=CARTESIAN_POINT('Ctrl Pts',(50.,-4.0549933858478,23.1917881898463));
#50227=CARTESIAN_POINT('Ctrl Pts',(50.,-4.02168672604364,23.2265202123558));
#50228=CARTESIAN_POINT('Ctrl Pts',(50.,-3.98787638414422,23.2607775544223));
#50229=CARTESIAN_POINT('Ctrl Pts',(50.,-3.95255838902044,23.2965624821128));
#50230=CARTESIAN_POINT('Ctrl Pts',(50.,-3.91669078391207,23.3318294533088));
#50231=CARTESIAN_POINT('Ctrl Pts',(50.,-3.88028650238535,23.3665676072239));
#50232=CARTESIAN_POINT('Origin',(50.,-18.,12.));
#50233=CARTESIAN_POINT('',(50.,-18.,12.));
#50234=CARTESIAN_POINT('',(50.,18.,12.));
#50235=CARTESIAN_POINT('',(50.,-18.,12.));
#50236=CARTESIAN_POINT('',(50.,18.,28.));
#50237=CARTESIAN_POINT('',(50.,18.,12.));
#50238=CARTESIAN_POINT('',(50.,12.,28.));
#50239=CARTESIAN_POINT('',(50.,-18.,28.));
#50240=CARTESIAN_POINT('',(50.,12.,48.));
#50241=CARTESIAN_POINT('',(50.,12.,28.));
#50242=CARTESIAN_POINT('',(50.,-12.,48.));
#50243=CARTESIAN_POINT('',(50.,-12.,48.));
#50244=CARTESIAN_POINT('',(50.,-12.,28.));
#50245=CARTESIAN_POINT('',(50.,-12.,28.));
#50246=CARTESIAN_POINT('',(50.,-18.,28.));
#50247=CARTESIAN_POINT('',(50.,-18.,28.));
#50248=CARTESIAN_POINT('',(50.,-18.,12.));
#50249=CARTESIAN_POINT('Origin',(25.,0.,20.));
#50250=CARTESIAN_POINT('Origin',(20.,-12.,48.));
#50251=CARTESIAN_POINT('',(20.,12.,48.));
#50252=CARTESIAN_POINT('',(20.,-12.,48.));
#50253=CARTESIAN_POINT('',(20.,-6.,48.));
#50254=CARTESIAN_POINT('',(20.,12.,73.));
#50255=CARTESIAN_POINT('',(20.,12.,48.));
#50256=CARTESIAN_POINT('',(20.,-12.,73.));
#50257=CARTESIAN_POINT('',(20.,-12.,73.));
#50258=CARTESIAN_POINT('',(20.,-12.,48.));
#50259=CARTESIAN_POINT('Origin',(10.,0.,73.));
#50260=CARTESIAN_POINT('',(0.,12.,73.));
#50261=CARTESIAN_POINT('',(0.,-12.,73.));
#50262=CARTESIAN_POINT('',(0.,12.,73.));
#50263=CARTESIAN_POINT('',(0.,-12.,73.));
#50264=CARTESIAN_POINT('',(20.,12.,73.));
#50265=CARTESIAN_POINT('Origin',(25.,0.,48.));
#50266=CARTESIAN_POINT('',(0.,-12.,48.));
#50267=CARTESIAN_POINT('',(50.,12.,48.));
#50268=CARTESIAN_POINT('Origin',(50.,12.,28.));
#50269=CARTESIAN_POINT('',(0.,12.,28.));
#50270=CARTESIAN_POINT('',(37.5,12.,28.));
#50271=CARTESIAN_POINT('',(0.,12.,28.));
#50272=CARTESIAN_POINT('Origin',(0.,-12.,28.));
#50273=CARTESIAN_POINT('',(0.,-12.,28.));
#50274=CARTESIAN_POINT('',(12.5,-12.,28.));
#50275=CARTESIAN_POINT('',(0.,-12.,28.));
#50276=CARTESIAN_POINT('Origin',(25.,0.,28.));
#50277=CARTESIAN_POINT('',(0.,18.,28.));
#50278=CARTESIAN_POINT('',(50.,18.,28.));
#50279=CARTESIAN_POINT('',(0.,18.,28.));
#50280=CARTESIAN_POINT('Origin',(25.,0.,28.));
#50281=CARTESIAN_POINT('',(0.,-18.,28.));
#50282=CARTESIAN_POINT('',(0.,18.,28.));
#50283=CARTESIAN_POINT('',(0.,-18.,28.));
#50284=CARTESIAN_POINT('Origin',(50.,18.,12.));
#50285=CARTESIAN_POINT('',(0.,18.,12.));
#50286=CARTESIAN_POINT('',(50.,18.,12.));
#50287=CARTESIAN_POINT('',(0.,18.,12.));
#50288=CARTESIAN_POINT('Origin',(0.,-18.,12.));
#50289=CARTESIAN_POINT('',(0.,-18.,12.));
#50290=CARTESIAN_POINT('',(0.,-18.,12.));
#50291=CARTESIAN_POINT('',(0.,-18.,12.));
#50292=CARTESIAN_POINT('Origin',(0.,18.,12.));
#50293=CARTESIAN_POINT('',(0.,18.,12.));
#50294=CARTESIAN_POINT('Origin',(25.,0.,12.));
#69469=UNCERTAINTY_MEASURE_WITH_UNIT(LENGTH_MEASURE(0.01),#69492,
'DISTANCE_ACCURACY_VALUE',
'Maximum model space distance between geometric entities at asserted c
onnectivities');
#69478=UNCERTAINTY_MEASURE_WITH_UNIT(LENGTH_MEASURE(0.01),#69492,
'DISTANCE_ACCURACY_VALUE',
'Maximum model space distance between geometric entities at asserted c
onnectivities');
#69482=(
GEOMETRIC_REPRESENTATION_CONTEXT(3)
GLOBAL_UNCERTAINTY_ASSIGNED_CONTEXT((#69469))
GLOBAL_UNIT_ASSIGNED_CONTEXT((#69492,#69494,#69495))
REPRESENTATION_CONTEXT('','3D')
);
#69491=(
GEOMETRIC_REPRESENTATION_CONTEXT(3)
GLOBAL_UNCERTAINTY_ASSIGNED_CONTEXT((#69478))
GLOBAL_UNIT_ASSIGNED_CONTEXT((#69492,#69494,#69495))
REPRESENTATION_CONTEXT('','3D')
);
#69492=(
LENGTH_UNIT()
NAMED_UNIT(*)
SI_UNIT(.MILLI.,.METRE.)
);
#69494=(
NAMED_UNIT(*)
PLANE_ANGLE_UNIT()
SI_UNIT($,.RADIAN.)
);
#69495=(
NAMED_UNIT(*)
SI_UNIT($,.STERADIAN.)
SOLID_ANGLE_UNIT()
);
#69499=SHAPE_DEFINITION_REPRESENTATION(#69511,#69573);
#69511=PRODUCT_DEFINITION_SHAPE('',$,#69586);
#69573=SHAPE_REPRESENTATION('',(#15370),#69482);
#69582=PRODUCT_DEFINITION_CONTEXT('part definition',#69620,'design');
#69586=PRODUCT_DEFINITION('Jaw','Jaw',#69598,#69582);
#69598=PRODUCT_DEFINITION_FORMATION('',$,#69625);
#69620=APPLICATION_CONTEXT(
'Core Data for Automotive Mechanical Design Process');
#69621=PRODUCT_CONTEXT('part definition',#69620,'mechanical');
#69625=PRODUCT('Jaw','Jaw',$,(#69621));
#69637=PRESENTATION_STYLE_ASSIGNMENT((#69647));
#69647=SURFACE_STYLE_USAGE(.BOTH.,#69657);
#69657=SURFACE_SIDE_STYLE('',(#69667));
#69667=SURFACE_STYLE_FILL_AREA(#69677);
#69677=FILL_AREA_STYLE('Sky blue',(#69687));
#69687=FILL_AREA_STYLE_COLOUR('Sky blue',#69697);
#69697=COLOUR_RGB('Sky blue',0.317647058823529,0.686274509803922,0.890196078431372);
ENDSEC;
END-ISO-10303-21;
